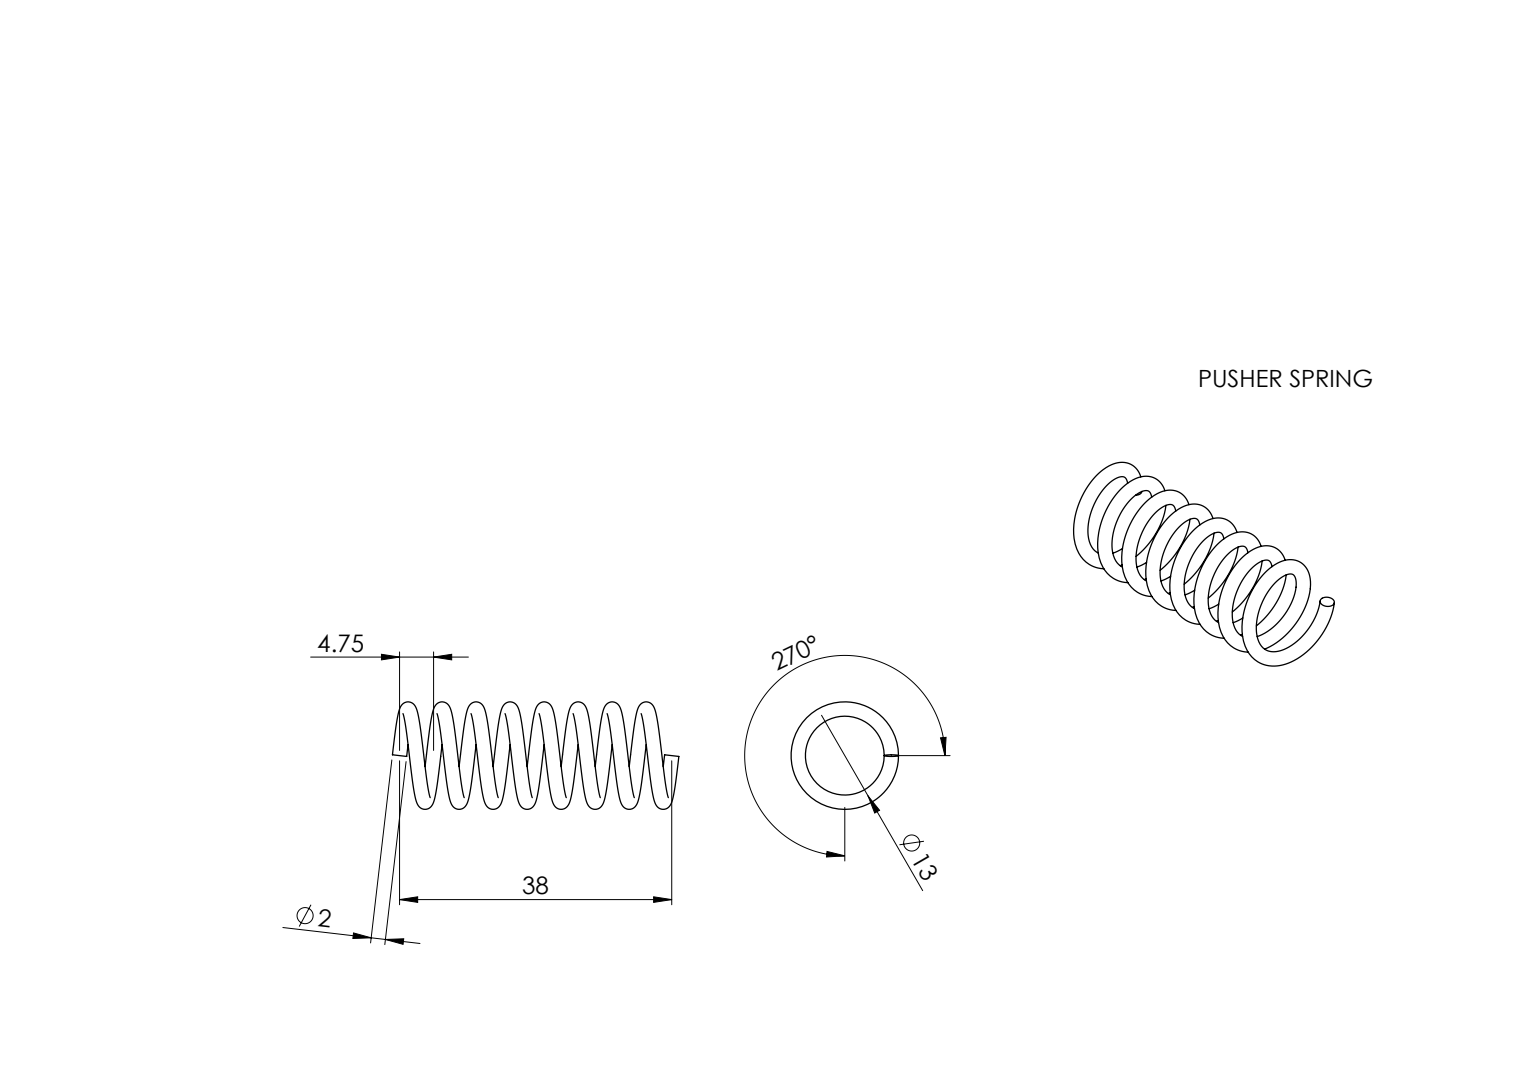
ISO-10303-21;
HEADER;
FILE_DESCRIPTION (('STEP AP214'),
    '1' );
FILE_NAME ('pusher spring.step',
    '2026-10-31T03:36:27',
    ( '' ),
    ( '' ),
    'SwSTEP 2.0',
    'SolidWorks 2026',
    '' );
FILE_SCHEMA (( 'AUTOMOTIVE_DESIGN' ));
ENDSEC;

DATA;
#2=CIRCLE ( 'NONE', #23019, 1.000000000000002220 ) ;
#26=CARTESIAN_POINT ( 'NONE',  ( -33.37127896937850124, 216.5309553116391612, 1.626142955000506873 ) ) ;
#28=( LENGTH_UNIT ( ) NAMED_UNIT ( * ) SI_UNIT ( .MILLI., .METRE. ) );
#30=CARTESIAN_POINT ( 'NONE',  ( -63.25669563604515844, 209.8844732041982297, -4.499999999999996447 ) ) ;
#31=CARTESIAN_POINT ( 'NONE',  ( -50.99330436395489841, 210.1155267958017134, -6.500000000000000888 ) ) ;
#37=CARTESIAN_POINT ( 'NONE',  ( -60.49330436395489130, 210.1155267958016850, -8.500000000000003553 ) ) ;
#42=CARTESIAN_POINT ( 'NONE',  ( -39.90997103062156270, 215.5714017266979852, 3.350049139982118618 ) ) ;
#53=CARTESIAN_POINT ( 'NONE',  ( -55.74330436395489841, 210.1155267958017134, -6.500000000000000888 ) ) ;
#71=( BOUNDED_CURVE ( )  B_SPLINE_CURVE ( 2, ( #25117, #31002, #36483, #31184, #33841, #22103, #11088, #7506, #25303, #25677, #37040, #22287, #37228, #16414, #5388, #22845, #19080, #4648, #7879, #11276, #5022, #24930, #13939, #16602, #28145, #33652, #16967, #25488, #30632, #10526, #31363, #36855, #10899, #7691, #16229, #4836, #13565, #22472, #28510, #14121, #27961, #34021, #8065, #19272, #19642, #36675, #30813, #10713, #22664, #5207, #2366, #16783, #28328, #1992, #34208, #8252, #19826, #3481, #14864, #31546, #34574, #20184, #28698, #32288, #14673, #14488, #2918, #17156, #23026, #25859, #2734, #8803, #31734, #28883, #12011, #11824, #37407, #31918, #8433, #630, #20376, #11637, #14307, #26045, #5947, #34761, #259, #29446, #34943, #8614, #26223, #17711, #6330, #5761, #23395, #72, #23211, #17527, #29061, #17341, #11458, #3105, #8987, #5571, #20744, #20558, #32102, #6133, #29251, #3292, #26411, #445, #23583, #35126, #9176, #17901, #15050, #26599, #12197, #34392, #20002, #7093, #10110, #21503, #12580, #29821, #21681, #33046, #32473, #15615, #24517, #12767, #24336, #33233, #18662, #30202, #27169, #26790, #4043, #21125, #18472, #15240, #20939, #21313, #35877, #26980, #35310, #4415, #12391, #4228, #1192, #9919, #1386, #15997, #12957, #1007, #27545, #6897, #30013, #18847, #24147, #35689, #36067, #15805, #32850, #27355, #9742, #7272, #30392, #1571, #23771, #9365, #6518, #18093, #29634, #3670, #821, #23961, #35504, #9551, #32664, #6705, #18277, #3855, #15431, #16364, #22423, #24885, #34157, #21865, #2129, #13326, #5344 ),
 .UNSPECIFIED., .F., .F. ) 
 B_SPLINE_CURVE_WITH_KNOTS ( ( 3, 2, 2, 2, 2, 2, 2, 2, 2, 2, 2, 2, 2, 2, 2, 2, 2, 2, 2, 2, 2, 2, 2, 2, 2, 2, 2, 2, 2, 2, 2, 2, 2, 2, 2, 2, 2, 2, 2, 2, 2, 2, 2, 2, 2, 2, 2, 2, 2, 2, 2, 2, 2, 2, 2, 2, 2, 2, 2, 2, 2, 2, 2, 2, 2, 2, 2, 2, 2, 2, 2, 2, 2, 2, 2, 2, 2, 2, 2, 2, 2, 2, 2, 2, 2, 2, 2, 2, 2, 2, 2, 2, 2, 2, 2, 2, 3 ),
 ( 0.000000000000000000, 0.01041666666666666609, 0.02083333333333333218, 0.03125000000000000000, 0.04166666666666666435, 0.05208333333333333565, 0.06250000000000000000, 0.07291666666666667129, 0.08333333333333332871, 0.09375000000000000000, 0.1041666666666666713, 0.1145833333333333287, 0.1250000000000000000, 0.1354166666666666574, 0.1458333333333333426, 0.1562500000000000000, 0.1666666666666666574, 0.1770833333333333426, 0.1875000000000000000, 0.1979166666666666574, 0.2083333333333333426, 0.2187500000000000000, 0.2291666666666666574, 0.2395833333333333426, 0.2500000000000000000, 0.2604166666666666852, 0.2708333333333333148, 0.2812500000000000000, 0.2916666666666666852, 0.3020833333333333148, 0.3125000000000000000, 0.3229166666666666852, 0.3333333333333333148, 0.3437500000000000000, 0.3541666666666666852, 0.3645833333333333148, 0.3750000000000000000, 0.3854166666666666852, 0.3958333333333333148, 0.4062500000000000000, 0.4166666666666666852, 0.4270833333333333148, 0.4375000000000000000, 0.4479166666666666852, 0.4583333333333333148, 0.4687500000000000000, 0.4791666666666666852, 0.4895833333333333148, 0.5000000000000000000, 0.5104166666666666297, 0.5208333333333333703, 0.5312500000000000000, 0.5416666666666666297, 0.5520833333333333703, 0.5625000000000000000, 0.5729166666666666297, 0.5833333333333333703, 0.5937500000000000000, 0.6041666666666666297, 0.6145833333333333703, 0.6250000000000000000, 0.6354166666666666297, 0.6458333333333333703, 0.6562500000000000000, 0.6666666666666666297, 0.6770833333333333703, 0.6875000000000000000, 0.6979166666666666297, 0.7083333333333333703, 0.7187500000000000000, 0.7291666666666666297, 0.7395833333333333703, 0.7500000000000000000, 0.7604166666666666297, 0.7708333333333333703, 0.7812500000000000000, 0.7916666666666666297, 0.8020833333333333703, 0.8125000000000000000, 0.8229166666666666297, 0.8333333333333333703, 0.8437500000000000000, 0.8541666666666666297, 0.8645833333333333703, 0.8750000000000000000, 0.8854166666666666297, 0.8958333333333333703, 0.9062500000000000000, 0.9166666666666666297, 0.9270833333333333703, 0.9375000000000000000, 0.9479166666666666297, 0.9583333333333333703, 0.9687500000000000000, 0.9791666666666666297, 0.9895833333333333703, 1.000000000000000000 ),
 .UNSPECIFIED. ) 
 CURVE ( )  GEOMETRIC_REPRESENTATION_ITEM ( )  RATIONAL_B_SPLINE_CURVE ( ( 1.000000000000000000, 0.9659258262890683122, 1.000000000000000000, 0.9659258262890683122, 1.000000000000000000, 0.9659258262890683122, 1.000000000000000000, 0.9659258262890683122, 1.000000000000000000, 0.9659258262890683122, 1.000000000000000000, 0.9659258262890683122, 1.000000000000000000, 0.9659258262890683122, 1.000000000000000000, 0.9659258262890683122, 1.000000000000000000, 0.9659258262890683122, 1.000000000000000000, 0.9659258262890683122, 1.000000000000000000, 0.9659258262890683122, 1.000000000000000000, 0.9659258262890683122, 1.000000000000000000, 0.9659258262890683122, 1.000000000000000000, 0.9659258262890683122, 1.000000000000000000, 0.9659258262890683122, 1.000000000000000000, 0.9659258262890683122, 1.000000000000000000, 0.9659258262890683122, 1.000000000000000000, 0.9659258262890683122, 1.000000000000000000, 0.9659258262890683122, 1.000000000000000000, 0.9659258262890683122, 1.000000000000000000, 0.9659258262890683122, 1.000000000000000000, 0.9659258262890683122, 1.000000000000000000, 0.9659258262890683122, 1.000000000000000000, 0.9659258262890683122, 1.000000000000000000, 0.9659258262890683122, 1.000000000000000000, 0.9659258262890683122, 1.000000000000000000, 0.9659258262890683122, 1.000000000000000000, 0.9659258262890683122, 1.000000000000000000, 0.9659258262890683122, 1.000000000000000000, 0.9659258262890683122, 1.000000000000000000, 0.9659258262890683122, 1.000000000000000000, 0.9659258262890683122, 1.000000000000000000, 0.9659258262890683122, 1.000000000000000000, 0.9659258262890683122, 1.000000000000000000, 0.9659258262890683122, 1.000000000000000000, 0.9659258262890683122, 1.000000000000000000, 0.9659258262890683122, 1.000000000000000000, 0.9659258262890683122, 1.000000000000000000, 0.9659258262890683122, 1.000000000000000000, 0.9659258262890683122, 1.000000000000000000, 0.9659258262890683122, 1.000000000000000000, 0.9659258262890683122, 1.000000000000000000, 0.9659258262890683122, 1.000000000000000000, 0.9659258262890683122, 1.000000000000000000, 0.9659258262890683122, 1.000000000000000000, 0.9659258262890683122, 1.000000000000000000, 0.9659258262890683122, 1.000000000000000000, 0.9659258262890683122, 1.000000000000000000, 0.9659258262890683122, 1.000000000000000000, 0.9659258262890683122, 1.000000000000000000, 0.9659258262890683122, 1.000000000000000000, 0.9659258262890683122, 1.000000000000000000, 0.9659258262890683122, 1.000000000000000000, 0.9659258262890683122, 1.000000000000000000, 0.9659258262890683122, 1.000000000000000000, 0.9659258262890683122, 1.000000000000000000, 0.9659258262890683122, 1.000000000000000000, 0.9659258262890683122, 1.000000000000000000, 0.9659258262890683122, 1.000000000000000000, 0.9659258262890683122, 1.000000000000000000, 0.9659258262890683122, 1.000000000000000000, 0.9659258262890683122, 1.000000000000000000, 0.9659258262890683122, 1.000000000000000000, 0.9659258262890683122, 1.000000000000000000, 0.9659258262890683122, 1.000000000000000000, 0.9659258262890683122, 1.000000000000000000, 0.9659258262890683122, 1.000000000000000000, 0.9659258262890683122, 1.000000000000000000, 0.9659258262890683122, 1.000000000000000000, 0.9659258262890683122, 1.000000000000000000, 0.9659258262890683122, 1.000000000000000000, 0.9659258262890683122, 1.000000000000000000, 0.9659258262890683122, 1.000000000000000000, 0.9659258262890683122, 1.000000000000000000, 0.9659258262890683122, 1.000000000000000000, 0.9659258262890683122, 1.000000000000000000, 0.9659258262890683122, 1.000000000000000000, 0.9659258262890683122, 1.000000000000000000, 0.9659258262890683122, 1.000000000000000000, 0.9659258262890683122, 1.000000000000000000, 0.9659258262890683122, 1.000000000000000000, 0.9659258262890683122, 1.000000000000000000, 0.9659258262890683122, 1.000000000000000000, 0.9659258262890683122, 1.000000000000000000, 0.9659258262890683122, 1.000000000000000000, 0.9659258262890683122, 1.000000000000000000, 0.9659258262890683122, 1.000000000000000000, 0.9659258262890683122, 1.000000000000000000, 0.9659258262890683122, 1.000000000000000000, 0.9659258262890683122, 1.000000000000000000, 0.9659258262890683122, 1.000000000000000000, 0.9659258262890683122, 1.000000000000000000, 0.9659258262890683122, 1.000000000000000000, 0.9659258262890683122, 1.000000000000000000, 0.9659258262890683122, 1.000000000000000000, 0.9659258262890683122, 1.000000000000000000 ) ) 
 REPRESENTATION_ITEM ( '' )  );
#72=CARTESIAN_POINT ( 'NONE',  ( -49.20461230271183695, 208.1428034533958851, -6.469044688360754414 ) ) ;
#74=CARTESIAN_POINT ( 'NONE',  ( -39.30877896937850124, 211.0902445701383101, -4.530955311639234040 ) ) ;
#77=CARTESIAN_POINT ( 'NONE',  ( -61.28497103062156981, 206.1606490808709111, -2.350049139982163027 ) ) ;
#78=CARTESIAN_POINT ( 'NONE',  ( -39.90997103062156270, 217.3034525342668815, 4.350049139982096413 ) ) ;
#83=CARTESIAN_POINT ( 'NONE',  ( -60.88169563604516554, 210.1155267958018271, 8.500000000000003553 ) ) ;
#96=CARTESIAN_POINT ( 'NONE',  ( -46.63913769728824121, 206.8500491399821044, -5.686928522499717253 ) ) ;
#124=CARTESIAN_POINT ( 'NONE',  ( -40.10788769728823411, 214.4690446883608104, 1.321298161741840893 ) ) ;
#129=CARTESIAN_POINT ( 'NONE',  ( -55.74330436395489841, 210.1155267958017134, -6.500000000000000888 ) ) ;
#180=CARTESIAN_POINT ( 'NONE',  ( -31.99330436395490196, 210.1155267958017134, -6.500000000000000888 ) ) ;
#216=CARTESIAN_POINT ( 'NONE',  ( -66.02752896937849414, 214.3500491399821897, 7.303452534266821949 ) ) ;
#218=FILL_AREA_STYLE ('',( #11593 ) ) ;
#220=CARTESIAN_POINT ( 'NONE',  ( -53.55877896937850124, 211.0902445701383101, -4.530955311639234040 ) ) ;
#221=CARTESIAN_POINT ( 'NONE',  ( -38.52455436395488420, 205.1570982666397356, 4.673758765035198159 ) ) ;
#227=CARTESIAN_POINT ( 'NONE',  ( -57.72247103062156270, 205.6499508600178956, 7.303452534266880569 ) ) ;
#233=CARTESIAN_POINT ( 'NONE',  ( -36.74330436395489841, 210.1155267958017134, -6.500000000000000888 ) ) ;
#244=CARTESIAN_POINT ( 'NONE',  ( -53.56622103062157692, 211.6261429550005744, 6.530955311639227823 ) ) ;
#259=CARTESIAN_POINT ( 'NONE',  ( -50.98586230271183695, 206.8500491399821328, 5.686928522499748340 ) ) ;
#262=CARTESIAN_POINT ( 'NONE',  ( -31.39211230271183339, 205.5309553116392465, 1.321298161741817356 ) ) ;
#266=CARTESIAN_POINT ( 'NONE',  ( -65.44122103062156270, 208.9097554298617752, -4.530955311639240257 ) ) ;
#267=CARTESIAN_POINT ( 'NONE',  ( -66.03497103062157692, 204.4285982733020148, -3.350049139982115509 ) ) ;
#271=CARTESIAN_POINT ( 'NONE',  ( -52.96502896937850124, 217.3034525342667962, -4.350049139982195001 ) ) ;
#281=CARTESIAN_POINT ( 'NONE',  ( -50.59747103062156270, 213.3500491399821328, -5.571401726697985168 ) ) ;
#307=CARTESIAN_POINT ( 'NONE',  ( -65.43377896937850835, 208.9097554298617183, 4.530955311639234040 ) ) ;
#311=CARTESIAN_POINT ( 'NONE',  ( -65.83705436395487709, 205.3262412349647263, -4.842901733360204020 ) ) ;
#312=CARTESIAN_POINT ( 'NONE',  ( -48.61086230271182984, 214.1499508600178387, -7.418979330068641964 ) ) ;
#327=CARTESIAN_POINT ( 'NONE',  ( -69.79538769728823411, 211.8571965466040012, -6.469044688360769513 ) ) ;
#365=CARTESIAN_POINT ( 'NONE',  ( -36.54538769728823411, 211.8571965466039444, -6.469044688360768625 ) ) ;
#400=CARTESIAN_POINT ( 'NONE',  ( -34.95461230271183695, 208.1428034533959135, -6.469044688360754414 ) ) ;
#403=CARTESIAN_POINT ( 'NONE',  ( -55.14211230271182984, 205.5309553116392465, 1.321298161741817356 ) ) ;
#404=CARTESIAN_POINT ( 'NONE',  ( -34.36830436395490551, 209.8844732041982581, 6.500000000000000888 ) ) ;
#410=CARTESIAN_POINT ( 'NONE',  ( -56.33705436395490551, 203.8621396198270475, -6.307003348497942419 ) ) ;
#417=CARTESIAN_POINT ( 'NONE',  ( -42.68080436395489841, 203.5000000000000000, -0.1155267958017335561 ) ) ;
#430=CARTESIAN_POINT ( 'NONE',  ( -58.51413769728823411, 213.1499508600178672, 5.686928522499718142 ) ) ;
#445=CARTESIAN_POINT ( 'NONE',  ( -46.03794563604517265, 205.3262412349648116, 4.842901733360249317 ) ) ;
#447=CARTESIAN_POINT ( 'NONE',  ( -64.64211230271182274, 203.5309553116391612, 1.857196546604092280 ) ) ;
#450=CARTESIAN_POINT ( 'NONE',  ( -63.26413769728823411, 212.1499508600178387, 3.954877714930865817 ) ) ;
#451=CARTESIAN_POINT ( 'NONE',  ( -32.38913769728823411, 205.8500491399820760, -7.418979330068584233 ) ) ;
#455=CARTESIAN_POINT ( 'NONE',  ( -56.72544563604517265, 216.3070033484980854, 6.137860380172893926 ) ) ;
#467=CARTESIAN_POINT ( 'NONE',  ( -46.83705436395489841, 205.3262412349647263, -4.842901733360204020 ) ) ;
#494=CARTESIAN_POINT ( 'NONE',  ( -33.18080436395489841, 205.4999999999999716, -0.1155267958017894420 ) ) ;
#498=CARTESIAN_POINT ( 'NONE',  ( -65.44122103062157692, 208.3738570449993404, -6.530955311639226935 ) ) ;
#499=CARTESIAN_POINT ( 'NONE',  ( -35.35044563604517265, 203.6929966515019430, -6.137860380172892150 ) ) ;
#504=CARTESIAN_POINT ( 'NONE',  ( -52.37127896937850124, 216.5309553116391612, 1.626142955000506873 ) ) ;
#548=CARTESIAN_POINT ( 'NONE',  ( -33.57663769728823411, 204.3130714775002730, 3.149950860017883603 ) ) ;
#566=FACE_OUTER_BOUND ( 'NONE', #21711, .T. ) ;
#583=CARTESIAN_POINT ( 'NONE',  ( -65.82961230271185116, 212.3930949314663792, 8.469044688360751749 ) ) ;
#587=CARTESIAN_POINT ( 'NONE',  ( -59.69419563604517265, 205.4999999999999716, 0.1155267958017633378 ) ) ;
#593=CARTESIAN_POINT ( 'NONE',  ( -61.68080436395489841, 201.5000000000000000, -0.1155267958017054536 ) ) ;
#600=CARTESIAN_POINT ( 'NONE',  ( -35.75372103062156981, 216.5309553116392181, -1.626142955000564383 ) ) ;
#613=CARTESIAN_POINT ( 'NONE',  ( -50.59747103062156270, 213.3500491399821328, -5.571401726697985168 ) ) ;
#630=CARTESIAN_POINT ( 'NONE',  ( -52.37127896937850124, 216.5309553116392181, 1.626142955000506429 ) ) ;
#632=CARTESIAN_POINT ( 'NONE',  ( -65.03794563604516554, 205.3262412349647832, 4.842901733360250205 ) ) ;
#635=CARTESIAN_POINT ( 'NONE',  ( -66.03497103062157692, 206.1606490808709111, -2.350049139982163027 ) ) ;
#636=CARTESIAN_POINT ( 'NONE',  ( -32.98288769728823411, 201.5309553116392181, -2.393094931466246855 ) ) ;
#641=CARTESIAN_POINT ( 'NONE',  ( -53.75669563604516554, 209.8844732041981729, -8.500000000000003553 ) ) ;
#652=CARTESIAN_POINT ( 'NONE',  ( -55.74330436395489841, 210.1155267958017134, -6.500000000000000888 ) ) ;
#680=CARTESIAN_POINT ( 'NONE',  ( -66.02752896937849414, 212.3500491399821613, 3.839350919129088435 ) ) ;
#684=CARTESIAN_POINT ( 'NONE',  ( -58.11830436395490551, 209.8844732041982581, 6.500000000000000888 ) ) ;
#685=CARTESIAN_POINT ( 'NONE',  ( -66.82663769728823411, 202.5810206699313767, 4.149950860017909804 ) ) ;
#690=CARTESIAN_POINT ( 'NONE',  ( -63.05877896937850835, 211.6261429550004607, -6.530955311639245586 ) ) ;
#697=CARTESIAN_POINT ( 'NONE',  ( -64.45163769728823411, 215.6869285224996986, -3.149950860017881382 ) ) ;
#736=CARTESIAN_POINT ( 'NONE',  ( -68.21205436395490551, 213.2096571498974242, 3.378800118222489601 ) ) ;
#777=CARTESIAN_POINT ( 'NONE',  ( -63.05877896937850835, 212.1620413398627534, -8.530955311639255356 ) ) ;
#780=CARTESIAN_POINT ( 'NONE',  ( -48.61086230271182984, 212.1499508600178387, -3.954877714930852495 ) ) ;
#781=CARTESIAN_POINT ( 'NONE',  ( -36.74330436395489841, 210.1155267958017134, -6.500000000000000888 ) ) ;
#786=CARTESIAN_POINT ( 'NONE',  ( -66.62872103062156270, 201.4690446883607819, 2.162041339862843525 ) ) ;
#793=CARTESIAN_POINT ( 'NONE',  ( -32.58705436395489841, 205.3262412349647548, -4.842901733360204908 ) ) ;
#821=CARTESIAN_POINT ( 'NONE',  ( -33.17336230271182984, 215.6869285224997270, 3.149950860017831200 ) ) ;
#823=CARTESIAN_POINT ( 'NONE',  ( -66.22544563604516554, 214.8429017333602360, 4.673758765035156415 ) ) ;
#828=CARTESIAN_POINT ( 'NONE',  ( -48.42038769728824832, 208.6787018382581778, 4.469044688360752637 ) ) ;
#829=CARTESIAN_POINT ( 'NONE',  ( -37.13913769728823411, 205.8500491399820760, -7.418979330068584233 ) ) ;
#833=CARTESIAN_POINT ( 'NONE',  ( -58.11086230271183695, 214.1499508600178387, -7.418979330068641964 ) ) ;
#842=CARTESIAN_POINT ( 'NONE',  ( -37.73288769728821279, 203.5309553116391612, -1.857196546604028775 ) ) ;
#871=CARTESIAN_POINT ( 'NONE',  ( -65.03794563604515133, 206.7903428501025758, 3.378800118222471838 ) ) ;
#875=CARTESIAN_POINT ( 'NONE',  ( -54.15997103062156981, 215.5714017266979852, 3.350049139982118618 ) ) ;
#876=CARTESIAN_POINT ( 'NONE',  ( -69.59747103062156270, 214.3500491399821044, -7.303452534266878793 ) ) ;
#881=CARTESIAN_POINT ( 'NONE',  ( -64.04836230271183695, 204.3130714775002446, -3.149950860017828091 ) ) ;
#888=CARTESIAN_POINT ( 'NONE',  ( -62.67038769728823411, 208.1428034533959703, 6.469044688360771289 ) ) ;
#893=CARTESIAN_POINT ( 'NONE',  ( -69.39955436395486288, 214.8429017333601792, -4.673758765035196383 ) ) ;
#965=CARTESIAN_POINT ( 'NONE',  ( -60.68377896937850835, 207.8379586601372750, 8.530955311639258909 ) ) ;
#969=CARTESIAN_POINT ( 'NONE',  ( -46.23586230271182984, 207.8500491399821613, 3.954877714930852495 ) ) ;
#974=CARTESIAN_POINT ( 'NONE',  ( -51.38913769728824121, 205.8500491399820760, -7.418979330068584233 ) ) ;
#1007=CARTESIAN_POINT ( 'NONE',  ( -37.32961230271182274, 211.8571965466040581, 6.469044688360755302 ) ) ;
#1008=CARTESIAN_POINT ( 'NONE',  ( -63.25669563604516554, 209.8844732041982013, -6.500000000000000888 ) ) ;
#1011=CARTESIAN_POINT ( 'NONE',  ( -44.85788769728823411, 214.4690446883608104, 1.321298161741840893 ) ) ;
#1012=CARTESIAN_POINT ( 'NONE',  ( -34.56622103062156981, 212.1620413398628671, 8.530955311639223382 ) ) ;
#1017=CARTESIAN_POINT ( 'NONE',  ( -50.78794563604517975, 203.8621396198271043, 6.307003348498029460 ) ) ;
#1031=CARTESIAN_POINT ( 'NONE',  ( -32.98288769728824121, 203.5309553116391612, -1.857196546604028775 ) ) ;
#1056=CARTESIAN_POINT ( 'NONE',  ( -34.17038769728823411, 208.6787018382581778, 4.469044688360752637 ) ) ;
#1061=CARTESIAN_POINT ( 'NONE',  ( -52.77455436395490551, 205.1570982666397356, 4.673758765035198159 ) ) ;
#1062=CARTESIAN_POINT ( 'NONE',  ( -67.61830436395490551, 209.8844732041983150, 8.500000000000003553 ) ) ;
#1069=CARTESIAN_POINT ( 'NONE',  ( -55.34002896937850124, 204.4285982733020433, 3.350049139982171020 ) ) ;
#1078=CARTESIAN_POINT ( 'NONE',  ( -69.39955436395487709, 214.8429017333601792, -4.673758765035197271 ) ) ;
#1082=CARTESIAN_POINT ( 'NONE',  ( -39.90997103062156270, 217.3034525342668815, 4.350049139982096413 ) ) ;
#1096=( BOUNDED_SURFACE ( )  B_SPLINE_SURFACE ( 3, 2, ( 
 ( #17208, #19878, #22527, #2787, #34446, #8486, #20056, #31601, #31421, #7933, #5265, #5624, #19508, #23080, #16843, #31054, #16469, #5076, #14361, #28202, #8124, #311, #26279, #498, #17583, #11877, #23446, #29308, #34999, #21179, #14915, #17398, #12254, #12064, #32344, #23638, #9227, #2973, #24016, #32154, #23824, #35366, #26464, #35561, #31973, #9418, #3160, #3347, #9042, #9605, #3538, #23266, #29499, #20993, #20801, #5816, #15293, #28938, #6003, #32528, #684, #35181, #14543, #6381, #26098, #17956, #11693, #20614, #34810, #26845, #15103, #26653, #129, #18145, #6571, #29687, #3721, #6194, #17766, #8855, #875, #12447, #20429, #29116, #14731, #13200, #6758, #1061, #29877, #18528, #30258, #30453, #27597, #13014, #12634, #9974, #15482, #33101, #21554, #24387, #16236, #1248, #24752, #18332, #24199, #3910, #30066, #4284, #4471, #1628, #24568, #35744, #36301, #27037, #9790, #27787, #30637, #16050, #36490, #10162, #1814, #7144, #10533, #7512, #15673, #13382, #32718, #24935, #21367, #12818, #32906, #10348, #21921, #33470, #35932, #6960, #18901, #4101, #18718, #19086, #27223, #15861, #27406, #1438, #36122, #4654, #21737, #33288, #7327, #2558, #14127, #25683, #8258, #19648, #16421, #10906, #37233, #25124, #31553, #22480, #13572, #17163, #28703, #28335, #13946, #31370, #16608, #5028, #16790, #33846, #28151, #2181, #8072, #13763, #37414, #31190, #33658, #28515, #2372, #11095, #25495, #37047, #19278, #2740, #34027, #11281, #22851, #5213, #14312, #10719, #34400, #19459, #22669 ),
 ( #34213, #25865, #5577, #22109, #22293, #8438, #16973, #19831, #7698, #5393, #30818, #20007, #27968, #25309, #36681, #4842, #1998, #7885, #31008, #36861, #635, #26606, #3297, #266, #23218, #31923, #29067, #34948, #3112, #26796, #20564, #23033, #17907, #17717, #450, #29256, #14869, #8621, #29639, #11829, #29451, #3486, #32106, #3676, #77, #15056, #8809, #8994, #14678, #15245, #9181, #28890, #35130, #12205, #26415, #11464, #20945, #34580, #11642, #23777, #6335, #6140, #20190, #12018, #31739, #23588, #17347, #5954, #2924, #32478, #20750, #32295, #5767, #35315, #9370, #6525, #18099, #23400, #26228, #14493, #26050, #34767, #20381, #17533, #6905, #18851, #12395, #6711, #35510, #24151, #35881, #36071, #33238, #18666, #18283, #7277, #9556, #3862, #33422, #36254, #10115, #4606, #15810, #7460, #27174, #16186, #13148, #21318, #19039, #828, #30591, #21131, #18477, #23967, #30398, #21686, #27549, #30018, #32669, #24522, #26985, #15620, #1577, #12585, #29826, #21869, #15436, #1011, #24702, #33051, #35694, #10297, #4421, #16002, #9746, #32856, #9924, #4048, #1198, #12771, #24341, #21507, #7098, #30207, #4234, #27360, #1390, #12963, #36998, #22247, #10668, #22430, #31142, #24890, #8392, #16557, #8208, #19784, #36814, #19961, #16371, #31321, #25074, #25263, #7835, #31504, #25445, #7650, #13897, #5349, #5161, #5526, #37184, #27735, #27916, #16926, #22617, #10857, #1766, #16740, #13332, #2325, #33611, #33798, #19227, #11227, #28287, #11041, #36440, #2505, #28468, #14078, #19594 ),
 ( #22798, #19408, #25628, #10479, #30771, #22058, #13517, #33978, #34164, #34349, #8019, #4793, #1946, #36628, #30958, #4976, #28103, #2135, #13714, #32060, #12156, #5905, #20893, #29406, #30, #23731, #32436, #35268, #25816, #34713, #9324, #23542, #26370, #6286, #23170, #17112, #3251, #5716, #31875, #17862, #28838, #28652, #587, #37361, #2689, #3438, #11784, #2872, #15007, #35087, #9137, #20702, #14825, #14632, #11415, #17485, #32246, #20140, #26559, #29017, #8572, #14265, #22983, #23352, #8948, #403, #11595, #8759, #34904, #14445, #20333, #3063, #26182, #220, #34533, #20521, #31687, #17297, #6089, #17673, #29210, #26001, #11970, #33197, #18239, #6480, #27511, #26748, #18052, #7238, #1159, #29783, #18812, #24483, #36029, #10073, #30166, #4003, #780, #32813, #21644, #9514, #15957, #6856, #35463, #1534, #13106, #12731, #35841, #15770, #969, #26938, #24298, #3814, #12545, #24110, #29973, #35654, #21831, #15578, #29594, #12920, #9883, #33005, #21464, #7055, #3631, #24661, #18432, #30356, #4380, #27132, #36213, #32627, #10255, #15391, #18625, #9700, #15200, #4193, #23922, #27320, #12348, #1348, #21087, #6664, #21277, #33572, #22574, #28251, #4933, #7425, #22388, #11185, #7980, #1723, #16328, #24848, #5310, #33938, #19553, #37143, #8170, #34120, #11002, #25223, #22206, #10627, #16144, #33755, #7795, #25029, #16888, #1907, #13857, #18994, #13292, #30551, #19184, #30914, #31102, #2280, #13675, #36398, #25405, #4568, #10444, #28424, #31282, #5123, #33385, #10817, #2465 ),
 ( #19745, #27876, #19372, #14039, #25588, #36956, #16703, #27695, #28062, #16515, #7608, #36772, #22019, #30733, #13477, #4756, #36588, #2097, #18152, #14922, #881, #35566, #29885, #35005, #12452, #690, #32726, #22759, #6576, #15109, #35188, #20999, #9233, #3916, #29693, #6763, #17963, #20808, #18337, #24021, #32350, #32536, #9612, #3546, #19925, #15489, #35372, #5485, #3726, #23831, #9048, #26471, #6388, #29505, #26660, #15299, #20620, #12261, #9424, #26852, #27043, #17068, #32160, #3354, #1069, #31463, #21186, #34308, #8352, #28608, #2645, #14221, #25771, #37323, #17772, #23452, #11884, #6199, #29314, #504, #12070, #23645, #4291, #9980, #1635, #16056, #13020, #24576, #36307, #1819, #33106, #1444, #33663, #27792, #4659, #27604, #10538, #7334, #36127, #24392, #24757, #33293, #7151, #12640, #7703, #27230, #1255, #30825, #10169, #18724, #24940, #12824, #21373, #4477, #27412, #32912, #18907, #13207, #21744, #4107, #6966, #30460, #10355, #30265, #4848, #13388, #22115, #16243, #36495, #35939, #21928, #15679, #33475, #7519, #27973, #16427, #19091, #30643, #35750, #21561, #19286, #24205, #15869, #9795, #18534, #30072, #13768, #17168, #16978, #11469, #2004, #22856, #31378, #13952, #37238, #25501, #20195, #34406, #23039, #34219, #37053, #34585, #28709, #11101, #11288, #2744, #19837, #36686, #31745, #14133, #22299, #8444, #2563, #25315, #5220, #22674, #8264, #5398, #20012, #36866, #28521, #25689, #31558, #5773, #33851, #10911, #19653, #8627, #10724, #5582, #17353, #14318, #37419 ),
 ( #25871, #13577, #25130, #7892, #2187, #19466, #31195, #22488, #31013, #5034, #2377, #16614, #28156, #34034, #8078, #28342, #16796, #6530, #20950, #6341, #26801, #23593, #29263, #3117, #3491, #12024, #11834, #28895, #12400, #5960, #17539, #9561, #26421, #23405, #3682, #29073, #83, #20755, #6145, #11647, #35135, #32301, #17722, #20387, #23223, #9187, #17911, #34954, #21137, #18104, #833, #32483, #15250, #14684, #29456, #31928, #12210, #455, #6717, #32674, #3303, #14873, #14498, #15062, #23973, #34772, #8999, #2930, #29644, #26612, #26055, #8813, #641, #26233, #23783, #35321, #271, #32111, #9376, #35516, #20569, #1583, #4053, #4239, #7282, #24708, #36445, #1017, #27179, #35887, #13337, #15441, #15815, #1771, #4426, #16192, #19045, #1395, #27742, #12590, #12776, #18483, #36260, #27365, #10303, #21874, #30023, #36076, #9931, #15626, #18856, #21692, #18672, #30214, #16008, #7466, #1203, #7103, #24896, #33426, #30596, #33242, #10485, #12970, #24527, #24346, #30404, #10120, #21512, #18289, #22065, #32864, #6912, #33616, #27556, #33056, #4611, #13153, #26989, #29832, #3868, #24156, #35699, #9751, #21324, #36634, #1952, #13903, #25451, #2140, #25823, #34355, #17120, #11234, #31510, #7841, #8215, #10673, #28475, #5168, #22990, #37370, #19599, #31149, #30775, #37004, #5533, #13522, #13720, #7655, #22252, #2696, #2514, #36820, #22806, #19968, #14272, #19413, #8400, #22623, #28658, #19232, #14085, #11047, #16746, #5355, #28293, #11423, #25635, #4798, #2332, #34170, #16376 ),
 ( #37191, #19790, #25079, #27921, #33804, #30963, #4981, #16563, #16933, #28109, #31327, #25268, #33982, #10862, #22435, #8025, #3637, #786, #15206, #5723, #14638, #26755, #3444, #6293, #23736, #3070, #12356, #20709, #23176, #11790, #35275, #8766, #34540, #18057, #17304, #8579, #9330, #29216, #20340, #20901, #15013, #26565, #593, #32252, #32068, #28845, #23358, #12163, #37, #6486, #34910, #26008, #29600, #20148, #3258, #26376, #17868, #29026, #17491, #14832, #31882, #26189, #227, #20526, #8954, #31694, #6096, #2879, #32442, #410, #23548, #11975, #35094, #14452, #11602, #17679, #34721, #5912, #9143, #29413, #26945, #10080, #35660, #1165, #6863, #1542, #27326, #29789, #4200, #24490, #7061, #13112, #4386, #24668, #974, #33204, #12926, #12737, #35469, #18632, #36219, #30172, #18245, #9707, #3820, #15964, #15777, #1354, #23928, #27517, #18818, #7244, #36036, #27138, #15584, #15398, #24304, #35847, #4010, #9521, #29980, #30362, #32633, #12551, #6671, #21093, #24117, #21283, #32819, #21650, #18439, #9889, #21472, #33012, #18920, #32738, #6774, #24033, #12837, #10368, #13031, #24771, #27617, #9991, #36321, #21199, #21385, #27056, #33307, #35952, #7347, #30471, #1082, #7162, #18547, #24217, #15881, #30276, #27243, #1266, #24587, #16069, #9807, #15692, #21943, #4492, #1648, #4302, #33488, #21572, #24404, #12652, #1458, #33118, #32925, #26864, #7533, #3928, #15501, #19106, #18735, #6977, #13220, #35762, #35578, #27425, #4119, #9622, #36139, #10180, #21756, #18349, #29897 ),
 ( #30657, #4672, #30086, #893, #12464, #27987, #36698, #33863, #2201, #7905, #31570, #25329, #27805, #22688, #22499, #5235, #34046, #19666, #13402, #34417, #5047, #34232, #8275, #36878, #8455, #4861, #19848, #13594, #13781, #19478, #20024, #13963, #33676, #2389, #31390, #31206, #16255, #25699, #1833, #16441, #5410, #11112, #10924, #24951, #16811, #36509, #28352, #22129, #10738, #7716, #37251, #25512, #37065, #10553, #16992, #19298, #30837, #2016, #25144, #8093, #28532, #2575, #14146, #22311, #11299, #31025, #16629, #22867, #28171, #14886, #9388, #20580, #652, #31939, #20962, #17923, #26068, #12222, #5592, #23793, #14329, #23234, #35332, #12035, #26433, #32312, #11658, #17179, #29275, #31755, #20398, #6354, #17365, #28720, #26622, #25883, #2757, #29468, #281, #28906, #3504, #23603, #35148, #9200, #3314, #3129, #37431, #5971, #20768, #8638, #15072, #17551, #34595, #11481, #23051, #11847, #34967, #467, #96, #34782, #23416, #2942, #8826, #29087, #14696, #26245, #20206, #9010, #5785, #14512, #32124, #6161, #17734, #35900, #29656, #13164, #21337, #12982, #24538, #4068, #24719, #21147, #36088, #29842, #30034, #12603, #36271, #30226, #12413, #18685, #10132, #9943, #10315, #4438, #32494, #32685, #21705, #27376, #15640, #6541, #21523, #18114, #7114, #842, #15452, #23985, #16019, #33070, #4252, #3692, #7294, #33255, #18868, #24358, #32876, #9761, #15260, #6923, #15826, #1406, #35529, #26813, #24167, #9573, #30416, #27567, #1596, #1031, #6729, #18302, #3878, #18494, #27004 ) ),
 .UNSPECIFIED., .T., .F., .F. ) 
 B_SPLINE_SURFACE_WITH_KNOTS ( ( 4, 3, 4 ),
 ( 3, 2, 2, 2, 2, 2, 2, 2, 2, 2, 2, 2, 2, 2, 2, 2, 2, 2, 2, 2, 2, 2, 2, 2, 2, 2, 2, 2, 2, 2, 2, 2, 2, 2, 2, 2, 2, 2, 2, 2, 2, 2, 2, 2, 2, 2, 2, 2, 2, 2, 2, 2, 2, 2, 2, 2, 2, 2, 2, 2, 2, 2, 2, 2, 2, 2, 2, 2, 2, 2, 2, 2, 2, 2, 2, 2, 2, 2, 2, 2, 2, 2, 2, 2, 2, 2, 2, 2, 2, 2, 2, 2, 2, 2, 2, 2, 3 ),
 ( 0.000000000000000000, 0.5000000000000000000, 1.000000000000000000 ),
 ( 0.000000000000000000, 0.01041666666666666609, 0.02083333333333333218, 0.03125000000000000000, 0.04166666666666666435, 0.05208333333333333565, 0.06250000000000000000, 0.07291666666666667129, 0.08333333333333332871, 0.09375000000000000000, 0.1041666666666666713, 0.1145833333333333287, 0.1250000000000000000, 0.1354166666666666574, 0.1458333333333333426, 0.1562500000000000000, 0.1666666666666666574, 0.1770833333333333426, 0.1875000000000000000, 0.1979166666666666574, 0.2083333333333333426, 0.2187500000000000000, 0.2291666666666666574, 0.2395833333333333426, 0.2500000000000000000, 0.2604166666666666852, 0.2708333333333333148, 0.2812500000000000000, 0.2916666666666666852, 0.3020833333333333148, 0.3125000000000000000, 0.3229166666666666852, 0.3333333333333333148, 0.3437500000000000000, 0.3541666666666666852, 0.3645833333333333148, 0.3750000000000000000, 0.3854166666666666852, 0.3958333333333333148, 0.4062500000000000000, 0.4166666666666666852, 0.4270833333333333148, 0.4375000000000000000, 0.4479166666666666852, 0.4583333333333333148, 0.4687500000000000000, 0.4791666666666666852, 0.4895833333333333148, 0.5000000000000000000, 0.5104166666666666297, 0.5208333333333333703, 0.5312500000000000000, 0.5416666666666666297, 0.5520833333333333703, 0.5625000000000000000, 0.5729166666666666297, 0.5833333333333333703, 0.5937500000000000000, 0.6041666666666666297, 0.6145833333333333703, 0.6250000000000000000, 0.6354166666666666297, 0.6458333333333333703, 0.6562500000000000000, 0.6666666666666666297, 0.6770833333333333703, 0.6875000000000000000, 0.6979166666666666297, 0.7083333333333333703, 0.7187500000000000000, 0.7291666666666666297, 0.7395833333333333703, 0.7500000000000000000, 0.7604166666666666297, 0.7708333333333333703, 0.7812500000000000000, 0.7916666666666666297, 0.8020833333333333703, 0.8125000000000000000, 0.8229166666666666297, 0.8333333333333333703, 0.8437500000000000000, 0.8541666666666666297, 0.8645833333333333703, 0.8750000000000000000, 0.8854166666666666297, 0.8958333333333333703, 0.9062500000000000000, 0.9166666666666666297, 0.9270833333333333703, 0.9375000000000000000, 0.9479166666666666297, 0.9583333333333333703, 0.9687500000000000000, 0.9791666666666666297, 0.9895833333333333703, 1.000000000000000000 ),
 .UNSPECIFIED. ) 
 GEOMETRIC_REPRESENTATION_ITEM ( )  RATIONAL_B_SPLINE_SURFACE ( (
 ( 1.000000000000000000, 0.9659258262890683122, 1.000000000000000000, 0.9659258262890683122, 1.000000000000000000, 0.9659258262890683122, 1.000000000000000000, 0.9659258262890683122, 1.000000000000000000, 0.9659258262890683122, 1.000000000000000000, 0.9659258262890683122, 1.000000000000000000, 0.9659258262890683122, 1.000000000000000000, 0.9659258262890683122, 1.000000000000000000, 0.9659258262890683122, 1.000000000000000000, 0.9659258262890683122, 1.000000000000000000, 0.9659258262890683122, 1.000000000000000000, 0.9659258262890683122, 1.000000000000000000, 0.9659258262890683122, 1.000000000000000000, 0.9659258262890683122, 1.000000000000000000, 0.9659258262890683122, 1.000000000000000000, 0.9659258262890683122, 1.000000000000000000, 0.9659258262890683122, 1.000000000000000000, 0.9659258262890683122, 1.000000000000000000, 0.9659258262890683122, 1.000000000000000000, 0.9659258262890683122, 1.000000000000000000, 0.9659258262890683122, 1.000000000000000000, 0.9659258262890683122, 1.000000000000000000, 0.9659258262890683122, 1.000000000000000000, 0.9659258262890683122, 1.000000000000000000, 0.9659258262890683122, 1.000000000000000000, 0.9659258262890683122, 1.000000000000000000, 0.9659258262890683122, 1.000000000000000000, 0.9659258262890683122, 1.000000000000000000, 0.9659258262890683122, 1.000000000000000000, 0.9659258262890683122, 1.000000000000000000, 0.9659258262890683122, 1.000000000000000000, 0.9659258262890683122, 1.000000000000000000, 0.9659258262890683122, 1.000000000000000000, 0.9659258262890683122, 1.000000000000000000, 0.9659258262890683122, 1.000000000000000000, 0.9659258262890683122, 1.000000000000000000, 0.9659258262890683122, 1.000000000000000000, 0.9659258262890683122, 1.000000000000000000, 0.9659258262890683122, 1.000000000000000000, 0.9659258262890683122, 1.000000000000000000, 0.9659258262890683122, 1.000000000000000000, 0.9659258262890683122, 1.000000000000000000, 0.9659258262890683122, 1.000000000000000000, 0.9659258262890683122, 1.000000000000000000, 0.9659258262890683122, 1.000000000000000000, 0.9659258262890683122, 1.000000000000000000, 0.9659258262890683122, 1.000000000000000000, 0.9659258262890683122, 1.000000000000000000, 0.9659258262890683122, 1.000000000000000000, 0.9659258262890683122, 1.000000000000000000, 0.9659258262890683122, 1.000000000000000000, 0.9659258262890683122, 1.000000000000000000, 0.9659258262890683122, 1.000000000000000000, 0.9659258262890683122, 1.000000000000000000, 0.9659258262890683122, 1.000000000000000000, 0.9659258262890683122, 1.000000000000000000, 0.9659258262890683122, 1.000000000000000000, 0.9659258262890683122, 1.000000000000000000, 0.9659258262890683122, 1.000000000000000000, 0.9659258262890683122, 1.000000000000000000, 0.9659258262890683122, 1.000000000000000000, 0.9659258262890683122, 1.000000000000000000, 0.9659258262890683122, 1.000000000000000000, 0.9659258262890683122, 1.000000000000000000, 0.9659258262890683122, 1.000000000000000000, 0.9659258262890683122, 1.000000000000000000, 0.9659258262890683122, 1.000000000000000000, 0.9659258262890683122, 1.000000000000000000, 0.9659258262890683122, 1.000000000000000000, 0.9659258262890683122, 1.000000000000000000, 0.9659258262890683122, 1.000000000000000000, 0.9659258262890683122, 1.000000000000000000, 0.9659258262890683122, 1.000000000000000000, 0.9659258262890683122, 1.000000000000000000, 0.9659258262890683122, 1.000000000000000000, 0.9659258262890683122, 1.000000000000000000, 0.9659258262890683122, 1.000000000000000000, 0.9659258262890683122, 1.000000000000000000, 0.9659258262890683122, 1.000000000000000000, 0.9659258262890683122, 1.000000000000000000, 0.9659258262890683122, 1.000000000000000000, 0.9659258262890683122, 1.000000000000000000, 0.9659258262890683122, 1.000000000000000000, 0.9659258262890683122, 1.000000000000000000, 0.9659258262890683122, 1.000000000000000000, 0.9659258262890683122, 1.000000000000000000, 0.9659258262890683122, 1.000000000000000000, 0.9659258262890683122, 1.000000000000000000, 0.9659258262890683122, 1.000000000000000000, 0.9659258262890683122, 1.000000000000000000, 0.9659258262890683122, 1.000000000000000000, 0.9659258262890683122, 1.000000000000000000, 0.9659258262890683122, 1.000000000000000000, 0.9659258262890683122, 1.000000000000000000, 0.9659258262890683122, 1.000000000000000000, 0.9659258262890683122, 1.000000000000000000),
 ( 0.3333333333333333703, 0.3219752754296894559, 0.3333333333333333703, 0.3219752754296894559, 0.3333333333333333703, 0.3219752754296894559, 0.3333333333333333703, 0.3219752754296894559, 0.3333333333333333703, 0.3219752754296894559, 0.3333333333333333703, 0.3219752754296894559, 0.3333333333333333703, 0.3219752754296894559, 0.3333333333333333703, 0.3219752754296894559, 0.3333333333333333703, 0.3219752754296894559, 0.3333333333333333703, 0.3219752754296894559, 0.3333333333333333703, 0.3219752754296894559, 0.3333333333333333703, 0.3219752754296894559, 0.3333333333333333703, 0.3219752754296894559, 0.3333333333333333703, 0.3219752754296894559, 0.3333333333333333703, 0.3219752754296894559, 0.3333333333333333703, 0.3219752754296894559, 0.3333333333333333703, 0.3219752754296894559, 0.3333333333333333703, 0.3219752754296894559, 0.3333333333333333703, 0.3219752754296894559, 0.3333333333333333703, 0.3219752754296894559, 0.3333333333333333703, 0.3219752754296894559, 0.3333333333333333703, 0.3219752754296894559, 0.3333333333333333703, 0.3219752754296894559, 0.3333333333333333703, 0.3219752754296894559, 0.3333333333333333703, 0.3219752754296894559, 0.3333333333333333703, 0.3219752754296894559, 0.3333333333333333703, 0.3219752754296894559, 0.3333333333333333703, 0.3219752754296894559, 0.3333333333333333703, 0.3219752754296894559, 0.3333333333333333703, 0.3219752754296894559, 0.3333333333333333703, 0.3219752754296894559, 0.3333333333333333703, 0.3219752754296894559, 0.3333333333333333703, 0.3219752754296894559, 0.3333333333333333703, 0.3219752754296894559, 0.3333333333333333703, 0.3219752754296894559, 0.3333333333333333703, 0.3219752754296894559, 0.3333333333333333703, 0.3219752754296894559, 0.3333333333333333703, 0.3219752754296894559, 0.3333333333333333703, 0.3219752754296894559, 0.3333333333333333703, 0.3219752754296894559, 0.3333333333333333703, 0.3219752754296894559, 0.3333333333333333703, 0.3219752754296894559, 0.3333333333333333703, 0.3219752754296894559, 0.3333333333333333703, 0.3219752754296894559, 0.3333333333333333703, 0.3219752754296894559, 0.3333333333333333703, 0.3219752754296894559, 0.3333333333333333703, 0.3219752754296894559, 0.3333333333333333703, 0.3219752754296894559, 0.3333333333333333703, 0.3219752754296894559, 0.3333333333333333703, 0.3219752754296894559, 0.3333333333333333703, 0.3219752754296894559, 0.3333333333333333703, 0.3219752754296894559, 0.3333333333333333703, 0.3219752754296894559, 0.3333333333333333703, 0.3219752754296894559, 0.3333333333333333703, 0.3219752754296894559, 0.3333333333333333703, 0.3219752754296894559, 0.3333333333333333703, 0.3219752754296894559, 0.3333333333333333703, 0.3219752754296894559, 0.3333333333333333703, 0.3219752754296894559, 0.3333333333333333703, 0.3219752754296894559, 0.3333333333333333703, 0.3219752754296894559, 0.3333333333333333703, 0.3219752754296894559, 0.3333333333333333703, 0.3219752754296894559, 0.3333333333333333703, 0.3219752754296894559, 0.3333333333333333703, 0.3219752754296894559, 0.3333333333333333703, 0.3219752754296894559, 0.3333333333333333703, 0.3219752754296894559, 0.3333333333333333703, 0.3219752754296894559, 0.3333333333333333703, 0.3219752754296894559, 0.3333333333333333703, 0.3219752754296894559, 0.3333333333333333703, 0.3219752754296894559, 0.3333333333333333703, 0.3219752754296894559, 0.3333333333333333703, 0.3219752754296894559, 0.3333333333333333703, 0.3219752754296894559, 0.3333333333333333703, 0.3219752754296894559, 0.3333333333333333703, 0.3219752754296894559, 0.3333333333333333703, 0.3219752754296894559, 0.3333333333333333703, 0.3219752754296894559, 0.3333333333333333703, 0.3219752754296894559, 0.3333333333333333703, 0.3219752754296894559, 0.3333333333333333703, 0.3219752754296894559, 0.3333333333333333703, 0.3219752754296894559, 0.3333333333333333703, 0.3219752754296894559, 0.3333333333333333703, 0.3219752754296894559, 0.3333333333333333703, 0.3219752754296894559, 0.3333333333333333703, 0.3219752754296894559, 0.3333333333333333703, 0.3219752754296894559, 0.3333333333333333703, 0.3219752754296894559, 0.3333333333333333703, 0.3219752754296894559, 0.3333333333333333703, 0.3219752754296894559, 0.3333333333333333703, 0.3219752754296894559, 0.3333333333333333703, 0.3219752754296894559, 0.3333333333333333703, 0.3219752754296894559, 0.3333333333333333703, 0.3219752754296894559, 0.3333333333333333703, 0.3219752754296894559, 0.3333333333333333703, 0.3219752754296894559, 0.3333333333333333703),
 ( 0.3333333333333333703, 0.3219752754296894559, 0.3333333333333333703, 0.3219752754296894559, 0.3333333333333333703, 0.3219752754296894559, 0.3333333333333333703, 0.3219752754296894559, 0.3333333333333333703, 0.3219752754296894559, 0.3333333333333333703, 0.3219752754296894559, 0.3333333333333333703, 0.3219752754296894559, 0.3333333333333333703, 0.3219752754296894559, 0.3333333333333333703, 0.3219752754296894559, 0.3333333333333333703, 0.3219752754296894559, 0.3333333333333333703, 0.3219752754296894559, 0.3333333333333333703, 0.3219752754296894559, 0.3333333333333333703, 0.3219752754296894559, 0.3333333333333333703, 0.3219752754296894559, 0.3333333333333333703, 0.3219752754296894559, 0.3333333333333333703, 0.3219752754296894559, 0.3333333333333333703, 0.3219752754296894559, 0.3333333333333333703, 0.3219752754296894559, 0.3333333333333333703, 0.3219752754296894559, 0.3333333333333333703, 0.3219752754296894559, 0.3333333333333333703, 0.3219752754296894559, 0.3333333333333333703, 0.3219752754296894559, 0.3333333333333333703, 0.3219752754296894559, 0.3333333333333333703, 0.3219752754296894559, 0.3333333333333333703, 0.3219752754296894559, 0.3333333333333333703, 0.3219752754296894559, 0.3333333333333333703, 0.3219752754296894559, 0.3333333333333333703, 0.3219752754296894559, 0.3333333333333333703, 0.3219752754296894559, 0.3333333333333333703, 0.3219752754296894559, 0.3333333333333333703, 0.3219752754296894559, 0.3333333333333333703, 0.3219752754296894559, 0.3333333333333333703, 0.3219752754296894559, 0.3333333333333333703, 0.3219752754296894559, 0.3333333333333333703, 0.3219752754296894559, 0.3333333333333333703, 0.3219752754296894559, 0.3333333333333333703, 0.3219752754296894559, 0.3333333333333333703, 0.3219752754296894559, 0.3333333333333333703, 0.3219752754296894559, 0.3333333333333333703, 0.3219752754296894559, 0.3333333333333333703, 0.3219752754296894559, 0.3333333333333333703, 0.3219752754296894559, 0.3333333333333333703, 0.3219752754296894559, 0.3333333333333333703, 0.3219752754296894559, 0.3333333333333333703, 0.3219752754296894559, 0.3333333333333333703, 0.3219752754296894559, 0.3333333333333333703, 0.3219752754296894559, 0.3333333333333333703, 0.3219752754296894559, 0.3333333333333333703, 0.3219752754296894559, 0.3333333333333333703, 0.3219752754296894559, 0.3333333333333333703, 0.3219752754296894559, 0.3333333333333333703, 0.3219752754296894559, 0.3333333333333333703, 0.3219752754296894559, 0.3333333333333333703, 0.3219752754296894559, 0.3333333333333333703, 0.3219752754296894559, 0.3333333333333333703, 0.3219752754296894559, 0.3333333333333333703, 0.3219752754296894559, 0.3333333333333333703, 0.3219752754296894559, 0.3333333333333333703, 0.3219752754296894559, 0.3333333333333333703, 0.3219752754296894559, 0.3333333333333333703, 0.3219752754296894559, 0.3333333333333333703, 0.3219752754296894559, 0.3333333333333333703, 0.3219752754296894559, 0.3333333333333333703, 0.3219752754296894559, 0.3333333333333333703, 0.3219752754296894559, 0.3333333333333333703, 0.3219752754296894559, 0.3333333333333333703, 0.3219752754296894559, 0.3333333333333333703, 0.3219752754296894559, 0.3333333333333333703, 0.3219752754296894559, 0.3333333333333333703, 0.3219752754296894559, 0.3333333333333333703, 0.3219752754296894559, 0.3333333333333333703, 0.3219752754296894559, 0.3333333333333333703, 0.3219752754296894559, 0.3333333333333333703, 0.3219752754296894559, 0.3333333333333333703, 0.3219752754296894559, 0.3333333333333333703, 0.3219752754296894559, 0.3333333333333333703, 0.3219752754296894559, 0.3333333333333333703, 0.3219752754296894559, 0.3333333333333333703, 0.3219752754296894559, 0.3333333333333333703, 0.3219752754296894559, 0.3333333333333333703, 0.3219752754296894559, 0.3333333333333333703, 0.3219752754296894559, 0.3333333333333333703, 0.3219752754296894559, 0.3333333333333333703, 0.3219752754296894559, 0.3333333333333333703, 0.3219752754296894559, 0.3333333333333333703, 0.3219752754296894559, 0.3333333333333333703, 0.3219752754296894559, 0.3333333333333333703, 0.3219752754296894559, 0.3333333333333333703, 0.3219752754296894559, 0.3333333333333333703, 0.3219752754296894559, 0.3333333333333333703, 0.3219752754296894559, 0.3333333333333333703, 0.3219752754296894559, 0.3333333333333333703, 0.3219752754296894559, 0.3333333333333333703, 0.3219752754296894559, 0.3333333333333333703, 0.3219752754296894559, 0.3333333333333333703, 0.3219752754296894559, 0.3333333333333333703),
 ( 1.000000000000000000, 0.9659258262890683122, 1.000000000000000000, 0.9659258262890683122, 1.000000000000000000, 0.9659258262890683122, 1.000000000000000000, 0.9659258262890683122, 1.000000000000000000, 0.9659258262890683122, 1.000000000000000000, 0.9659258262890683122, 1.000000000000000000, 0.9659258262890683122, 1.000000000000000000, 0.9659258262890683122, 1.000000000000000000, 0.9659258262890683122, 1.000000000000000000, 0.9659258262890683122, 1.000000000000000000, 0.9659258262890683122, 1.000000000000000000, 0.9659258262890683122, 1.000000000000000000, 0.9659258262890683122, 1.000000000000000000, 0.9659258262890683122, 1.000000000000000000, 0.9659258262890683122, 1.000000000000000000, 0.9659258262890683122, 1.000000000000000000, 0.9659258262890683122, 1.000000000000000000, 0.9659258262890683122, 1.000000000000000000, 0.9659258262890683122, 1.000000000000000000, 0.9659258262890683122, 1.000000000000000000, 0.9659258262890683122, 1.000000000000000000, 0.9659258262890683122, 1.000000000000000000, 0.9659258262890683122, 1.000000000000000000, 0.9659258262890683122, 1.000000000000000000, 0.9659258262890683122, 1.000000000000000000, 0.9659258262890683122, 1.000000000000000000, 0.9659258262890683122, 1.000000000000000000, 0.9659258262890683122, 1.000000000000000000, 0.9659258262890683122, 1.000000000000000000, 0.9659258262890683122, 1.000000000000000000, 0.9659258262890683122, 1.000000000000000000, 0.9659258262890683122, 1.000000000000000000, 0.9659258262890683122, 1.000000000000000000, 0.9659258262890683122, 1.000000000000000000, 0.9659258262890683122, 1.000000000000000000, 0.9659258262890683122, 1.000000000000000000, 0.9659258262890683122, 1.000000000000000000, 0.9659258262890683122, 1.000000000000000000, 0.9659258262890683122, 1.000000000000000000, 0.9659258262890683122, 1.000000000000000000, 0.9659258262890683122, 1.000000000000000000, 0.9659258262890683122, 1.000000000000000000, 0.9659258262890683122, 1.000000000000000000, 0.9659258262890683122, 1.000000000000000000, 0.9659258262890683122, 1.000000000000000000, 0.9659258262890683122, 1.000000000000000000, 0.9659258262890683122, 1.000000000000000000, 0.9659258262890683122, 1.000000000000000000, 0.9659258262890683122, 1.000000000000000000, 0.9659258262890683122, 1.000000000000000000, 0.9659258262890683122, 1.000000000000000000, 0.9659258262890683122, 1.000000000000000000, 0.9659258262890683122, 1.000000000000000000, 0.9659258262890683122, 1.000000000000000000, 0.9659258262890683122, 1.000000000000000000, 0.9659258262890683122, 1.000000000000000000, 0.9659258262890683122, 1.000000000000000000, 0.9659258262890683122, 1.000000000000000000, 0.9659258262890683122, 1.000000000000000000, 0.9659258262890683122, 1.000000000000000000, 0.9659258262890683122, 1.000000000000000000, 0.9659258262890683122, 1.000000000000000000, 0.9659258262890683122, 1.000000000000000000, 0.9659258262890683122, 1.000000000000000000, 0.9659258262890683122, 1.000000000000000000, 0.9659258262890683122, 1.000000000000000000, 0.9659258262890683122, 1.000000000000000000, 0.9659258262890683122, 1.000000000000000000, 0.9659258262890683122, 1.000000000000000000, 0.9659258262890683122, 1.000000000000000000, 0.9659258262890683122, 1.000000000000000000, 0.9659258262890683122, 1.000000000000000000, 0.9659258262890683122, 1.000000000000000000, 0.9659258262890683122, 1.000000000000000000, 0.9659258262890683122, 1.000000000000000000, 0.9659258262890683122, 1.000000000000000000, 0.9659258262890683122, 1.000000000000000000, 0.9659258262890683122, 1.000000000000000000, 0.9659258262890683122, 1.000000000000000000, 0.9659258262890683122, 1.000000000000000000, 0.9659258262890683122, 1.000000000000000000, 0.9659258262890683122, 1.000000000000000000, 0.9659258262890683122, 1.000000000000000000, 0.9659258262890683122, 1.000000000000000000, 0.9659258262890683122, 1.000000000000000000, 0.9659258262890683122, 1.000000000000000000, 0.9659258262890683122, 1.000000000000000000, 0.9659258262890683122, 1.000000000000000000, 0.9659258262890683122, 1.000000000000000000, 0.9659258262890683122, 1.000000000000000000, 0.9659258262890683122, 1.000000000000000000, 0.9659258262890683122, 1.000000000000000000, 0.9659258262890683122, 1.000000000000000000, 0.9659258262890683122, 1.000000000000000000, 0.9659258262890683122, 1.000000000000000000, 0.9659258262890683122, 1.000000000000000000),
 ( 0.3333333333333333703, 0.3219752754296894559, 0.3333333333333333703, 0.3219752754296894559, 0.3333333333333333703, 0.3219752754296894559, 0.3333333333333333703, 0.3219752754296894559, 0.3333333333333333703, 0.3219752754296894559, 0.3333333333333333703, 0.3219752754296894559, 0.3333333333333333703, 0.3219752754296894559, 0.3333333333333333703, 0.3219752754296894559, 0.3333333333333333703, 0.3219752754296894559, 0.3333333333333333703, 0.3219752754296894559, 0.3333333333333333703, 0.3219752754296894559, 0.3333333333333333703, 0.3219752754296894559, 0.3333333333333333703, 0.3219752754296894559, 0.3333333333333333703, 0.3219752754296894559, 0.3333333333333333703, 0.3219752754296894559, 0.3333333333333333703, 0.3219752754296894559, 0.3333333333333333703, 0.3219752754296894559, 0.3333333333333333703, 0.3219752754296894559, 0.3333333333333333703, 0.3219752754296894559, 0.3333333333333333703, 0.3219752754296894559, 0.3333333333333333703, 0.3219752754296894559, 0.3333333333333333703, 0.3219752754296894559, 0.3333333333333333703, 0.3219752754296894559, 0.3333333333333333703, 0.3219752754296894559, 0.3333333333333333703, 0.3219752754296894559, 0.3333333333333333703, 0.3219752754296894559, 0.3333333333333333703, 0.3219752754296894559, 0.3333333333333333703, 0.3219752754296894559, 0.3333333333333333703, 0.3219752754296894559, 0.3333333333333333703, 0.3219752754296894559, 0.3333333333333333703, 0.3219752754296894559, 0.3333333333333333703, 0.3219752754296894559, 0.3333333333333333703, 0.3219752754296894559, 0.3333333333333333703, 0.3219752754296894559, 0.3333333333333333703, 0.3219752754296894559, 0.3333333333333333703, 0.3219752754296894559, 0.3333333333333333703, 0.3219752754296894559, 0.3333333333333333703, 0.3219752754296894559, 0.3333333333333333703, 0.3219752754296894559, 0.3333333333333333703, 0.3219752754296894559, 0.3333333333333333703, 0.3219752754296894559, 0.3333333333333333703, 0.3219752754296894559, 0.3333333333333333703, 0.3219752754296894559, 0.3333333333333333703, 0.3219752754296894559, 0.3333333333333333703, 0.3219752754296894559, 0.3333333333333333703, 0.3219752754296894559, 0.3333333333333333703, 0.3219752754296894559, 0.3333333333333333703, 0.3219752754296894559, 0.3333333333333333703, 0.3219752754296894559, 0.3333333333333333703, 0.3219752754296894559, 0.3333333333333333703, 0.3219752754296894559, 0.3333333333333333703, 0.3219752754296894559, 0.3333333333333333703, 0.3219752754296894559, 0.3333333333333333703, 0.3219752754296894559, 0.3333333333333333703, 0.3219752754296894559, 0.3333333333333333703, 0.3219752754296894559, 0.3333333333333333703, 0.3219752754296894559, 0.3333333333333333703, 0.3219752754296894559, 0.3333333333333333703, 0.3219752754296894559, 0.3333333333333333703, 0.3219752754296894559, 0.3333333333333333703, 0.3219752754296894559, 0.3333333333333333703, 0.3219752754296894559, 0.3333333333333333703, 0.3219752754296894559, 0.3333333333333333703, 0.3219752754296894559, 0.3333333333333333703, 0.3219752754296894559, 0.3333333333333333703, 0.3219752754296894559, 0.3333333333333333703, 0.3219752754296894559, 0.3333333333333333703, 0.3219752754296894559, 0.3333333333333333703, 0.3219752754296894559, 0.3333333333333333703, 0.3219752754296894559, 0.3333333333333333703, 0.3219752754296894559, 0.3333333333333333703, 0.3219752754296894559, 0.3333333333333333703, 0.3219752754296894559, 0.3333333333333333703, 0.3219752754296894559, 0.3333333333333333703, 0.3219752754296894559, 0.3333333333333333703, 0.3219752754296894559, 0.3333333333333333703, 0.3219752754296894559, 0.3333333333333333703, 0.3219752754296894559, 0.3333333333333333703, 0.3219752754296894559, 0.3333333333333333703, 0.3219752754296894559, 0.3333333333333333703, 0.3219752754296894559, 0.3333333333333333703, 0.3219752754296894559, 0.3333333333333333703, 0.3219752754296894559, 0.3333333333333333703, 0.3219752754296894559, 0.3333333333333333703, 0.3219752754296894559, 0.3333333333333333703, 0.3219752754296894559, 0.3333333333333333703, 0.3219752754296894559, 0.3333333333333333703, 0.3219752754296894559, 0.3333333333333333703, 0.3219752754296894559, 0.3333333333333333703, 0.3219752754296894559, 0.3333333333333333703, 0.3219752754296894559, 0.3333333333333333703, 0.3219752754296894559, 0.3333333333333333703, 0.3219752754296894559, 0.3333333333333333703, 0.3219752754296894559, 0.3333333333333333703, 0.3219752754296894559, 0.3333333333333333703, 0.3219752754296894559, 0.3333333333333333703),
 ( 0.3333333333333333703, 0.3219752754296894559, 0.3333333333333333703, 0.3219752754296894559, 0.3333333333333333703, 0.3219752754296894559, 0.3333333333333333703, 0.3219752754296894559, 0.3333333333333333703, 0.3219752754296894559, 0.3333333333333333703, 0.3219752754296894559, 0.3333333333333333703, 0.3219752754296894559, 0.3333333333333333703, 0.3219752754296894559, 0.3333333333333333703, 0.3219752754296894559, 0.3333333333333333703, 0.3219752754296894559, 0.3333333333333333703, 0.3219752754296894559, 0.3333333333333333703, 0.3219752754296894559, 0.3333333333333333703, 0.3219752754296894559, 0.3333333333333333703, 0.3219752754296894559, 0.3333333333333333703, 0.3219752754296894559, 0.3333333333333333703, 0.3219752754296894559, 0.3333333333333333703, 0.3219752754296894559, 0.3333333333333333703, 0.3219752754296894559, 0.3333333333333333703, 0.3219752754296894559, 0.3333333333333333703, 0.3219752754296894559, 0.3333333333333333703, 0.3219752754296894559, 0.3333333333333333703, 0.3219752754296894559, 0.3333333333333333703, 0.3219752754296894559, 0.3333333333333333703, 0.3219752754296894559, 0.3333333333333333703, 0.3219752754296894559, 0.3333333333333333703, 0.3219752754296894559, 0.3333333333333333703, 0.3219752754296894559, 0.3333333333333333703, 0.3219752754296894559, 0.3333333333333333703, 0.3219752754296894559, 0.3333333333333333703, 0.3219752754296894559, 0.3333333333333333703, 0.3219752754296894559, 0.3333333333333333703, 0.3219752754296894559, 0.3333333333333333703, 0.3219752754296894559, 0.3333333333333333703, 0.3219752754296894559, 0.3333333333333333703, 0.3219752754296894559, 0.3333333333333333703, 0.3219752754296894559, 0.3333333333333333703, 0.3219752754296894559, 0.3333333333333333703, 0.3219752754296894559, 0.3333333333333333703, 0.3219752754296894559, 0.3333333333333333703, 0.3219752754296894559, 0.3333333333333333703, 0.3219752754296894559, 0.3333333333333333703, 0.3219752754296894559, 0.3333333333333333703, 0.3219752754296894559, 0.3333333333333333703, 0.3219752754296894559, 0.3333333333333333703, 0.3219752754296894559, 0.3333333333333333703, 0.3219752754296894559, 0.3333333333333333703, 0.3219752754296894559, 0.3333333333333333703, 0.3219752754296894559, 0.3333333333333333703, 0.3219752754296894559, 0.3333333333333333703, 0.3219752754296894559, 0.3333333333333333703, 0.3219752754296894559, 0.3333333333333333703, 0.3219752754296894559, 0.3333333333333333703, 0.3219752754296894559, 0.3333333333333333703, 0.3219752754296894559, 0.3333333333333333703, 0.3219752754296894559, 0.3333333333333333703, 0.3219752754296894559, 0.3333333333333333703, 0.3219752754296894559, 0.3333333333333333703, 0.3219752754296894559, 0.3333333333333333703, 0.3219752754296894559, 0.3333333333333333703, 0.3219752754296894559, 0.3333333333333333703, 0.3219752754296894559, 0.3333333333333333703, 0.3219752754296894559, 0.3333333333333333703, 0.3219752754296894559, 0.3333333333333333703, 0.3219752754296894559, 0.3333333333333333703, 0.3219752754296894559, 0.3333333333333333703, 0.3219752754296894559, 0.3333333333333333703, 0.3219752754296894559, 0.3333333333333333703, 0.3219752754296894559, 0.3333333333333333703, 0.3219752754296894559, 0.3333333333333333703, 0.3219752754296894559, 0.3333333333333333703, 0.3219752754296894559, 0.3333333333333333703, 0.3219752754296894559, 0.3333333333333333703, 0.3219752754296894559, 0.3333333333333333703, 0.3219752754296894559, 0.3333333333333333703, 0.3219752754296894559, 0.3333333333333333703, 0.3219752754296894559, 0.3333333333333333703, 0.3219752754296894559, 0.3333333333333333703, 0.3219752754296894559, 0.3333333333333333703, 0.3219752754296894559, 0.3333333333333333703, 0.3219752754296894559, 0.3333333333333333703, 0.3219752754296894559, 0.3333333333333333703, 0.3219752754296894559, 0.3333333333333333703, 0.3219752754296894559, 0.3333333333333333703, 0.3219752754296894559, 0.3333333333333333703, 0.3219752754296894559, 0.3333333333333333703, 0.3219752754296894559, 0.3333333333333333703, 0.3219752754296894559, 0.3333333333333333703, 0.3219752754296894559, 0.3333333333333333703, 0.3219752754296894559, 0.3333333333333333703, 0.3219752754296894559, 0.3333333333333333703, 0.3219752754296894559, 0.3333333333333333703, 0.3219752754296894559, 0.3333333333333333703, 0.3219752754296894559, 0.3333333333333333703, 0.3219752754296894559, 0.3333333333333333703, 0.3219752754296894559, 0.3333333333333333703, 0.3219752754296894559, 0.3333333333333333703),
 ( 1.000000000000000000, 0.9659258262890683122, 1.000000000000000000, 0.9659258262890683122, 1.000000000000000000, 0.9659258262890683122, 1.000000000000000000, 0.9659258262890683122, 1.000000000000000000, 0.9659258262890683122, 1.000000000000000000, 0.9659258262890683122, 1.000000000000000000, 0.9659258262890683122, 1.000000000000000000, 0.9659258262890683122, 1.000000000000000000, 0.9659258262890683122, 1.000000000000000000, 0.9659258262890683122, 1.000000000000000000, 0.9659258262890683122, 1.000000000000000000, 0.9659258262890683122, 1.000000000000000000, 0.9659258262890683122, 1.000000000000000000, 0.9659258262890683122, 1.000000000000000000, 0.9659258262890683122, 1.000000000000000000, 0.9659258262890683122, 1.000000000000000000, 0.9659258262890683122, 1.000000000000000000, 0.9659258262890683122, 1.000000000000000000, 0.9659258262890683122, 1.000000000000000000, 0.9659258262890683122, 1.000000000000000000, 0.9659258262890683122, 1.000000000000000000, 0.9659258262890683122, 1.000000000000000000, 0.9659258262890683122, 1.000000000000000000, 0.9659258262890683122, 1.000000000000000000, 0.9659258262890683122, 1.000000000000000000, 0.9659258262890683122, 1.000000000000000000, 0.9659258262890683122, 1.000000000000000000, 0.9659258262890683122, 1.000000000000000000, 0.9659258262890683122, 1.000000000000000000, 0.9659258262890683122, 1.000000000000000000, 0.9659258262890683122, 1.000000000000000000, 0.9659258262890683122, 1.000000000000000000, 0.9659258262890683122, 1.000000000000000000, 0.9659258262890683122, 1.000000000000000000, 0.9659258262890683122, 1.000000000000000000, 0.9659258262890683122, 1.000000000000000000, 0.9659258262890683122, 1.000000000000000000, 0.9659258262890683122, 1.000000000000000000, 0.9659258262890683122, 1.000000000000000000, 0.9659258262890683122, 1.000000000000000000, 0.9659258262890683122, 1.000000000000000000, 0.9659258262890683122, 1.000000000000000000, 0.9659258262890683122, 1.000000000000000000, 0.9659258262890683122, 1.000000000000000000, 0.9659258262890683122, 1.000000000000000000, 0.9659258262890683122, 1.000000000000000000, 0.9659258262890683122, 1.000000000000000000, 0.9659258262890683122, 1.000000000000000000, 0.9659258262890683122, 1.000000000000000000, 0.9659258262890683122, 1.000000000000000000, 0.9659258262890683122, 1.000000000000000000, 0.9659258262890683122, 1.000000000000000000, 0.9659258262890683122, 1.000000000000000000, 0.9659258262890683122, 1.000000000000000000, 0.9659258262890683122, 1.000000000000000000, 0.9659258262890683122, 1.000000000000000000, 0.9659258262890683122, 1.000000000000000000, 0.9659258262890683122, 1.000000000000000000, 0.9659258262890683122, 1.000000000000000000, 0.9659258262890683122, 1.000000000000000000, 0.9659258262890683122, 1.000000000000000000, 0.9659258262890683122, 1.000000000000000000, 0.9659258262890683122, 1.000000000000000000, 0.9659258262890683122, 1.000000000000000000, 0.9659258262890683122, 1.000000000000000000, 0.9659258262890683122, 1.000000000000000000, 0.9659258262890683122, 1.000000000000000000, 0.9659258262890683122, 1.000000000000000000, 0.9659258262890683122, 1.000000000000000000, 0.9659258262890683122, 1.000000000000000000, 0.9659258262890683122, 1.000000000000000000, 0.9659258262890683122, 1.000000000000000000, 0.9659258262890683122, 1.000000000000000000, 0.9659258262890683122, 1.000000000000000000, 0.9659258262890683122, 1.000000000000000000, 0.9659258262890683122, 1.000000000000000000, 0.9659258262890683122, 1.000000000000000000, 0.9659258262890683122, 1.000000000000000000, 0.9659258262890683122, 1.000000000000000000, 0.9659258262890683122, 1.000000000000000000, 0.9659258262890683122, 1.000000000000000000, 0.9659258262890683122, 1.000000000000000000, 0.9659258262890683122, 1.000000000000000000, 0.9659258262890683122, 1.000000000000000000, 0.9659258262890683122, 1.000000000000000000, 0.9659258262890683122, 1.000000000000000000, 0.9659258262890683122, 1.000000000000000000, 0.9659258262890683122, 1.000000000000000000, 0.9659258262890683122, 1.000000000000000000, 0.9659258262890683122, 1.000000000000000000, 0.9659258262890683122, 1.000000000000000000, 0.9659258262890683122, 1.000000000000000000, 0.9659258262890683122, 1.000000000000000000, 0.9659258262890683122, 1.000000000000000000, 0.9659258262890683122, 1.000000000000000000, 0.9659258262890683122, 1.000000000000000000) ) ) 
 REPRESENTATION_ITEM ( '' )  SURFACE ( )  );
#1155=CARTESIAN_POINT ( 'NONE',  ( -52.76711230271184405, 218.4690446883607535, -2.393094931466363651 ) ) ;
#1159=CARTESIAN_POINT ( 'NONE',  ( -50.19419563604517975, 205.4999999999999716, 0.1155267958017633378 ) ) ;
#1165=CARTESIAN_POINT ( 'NONE',  ( -53.56622103062157692, 212.1620413398628671, 8.530955311639223382 ) ) ;
#1192=CARTESIAN_POINT ( 'NONE',  ( -38.31919563604516554, 216.5000000000000000, -0.1155267958017906493 ) ) ;
#1194=CARTESIAN_POINT ( 'NONE',  ( -57.71502896937850124, 215.5714017266979567, -3.350049139982168800 ) ) ;
#1198=CARTESIAN_POINT ( 'NONE',  ( -42.68080436395489841, 205.4999999999999716, -0.1155267958017894420 ) ) ;
#1199=CARTESIAN_POINT ( 'NONE',  ( -51.78497103062156981, 204.4285982733020148, -3.350049139982115509 ) ) ;
#1203=CARTESIAN_POINT ( 'NONE',  ( -45.04836230271183695, 202.5810206699313767, -4.149950860017804111 ) ) ;
#1215=ADVANCED_FACE ( 'NONE', ( #29833 ), #3119, .T. ) ;
#1244=CARTESIAN_POINT ( 'NONE',  ( -50.78794563604517975, 206.7903428501025758, 3.378800118222471838 ) ) ;
#1248=CARTESIAN_POINT ( 'NONE',  ( -50.00372103062157692, 216.5309553116391612, -1.626142955000564383 ) ) ;
#1249=CARTESIAN_POINT ( 'NONE',  ( -30.99627896937850480, 201.4690446883607251, -2.162041339862721845 ) ) ;
#1255=CARTESIAN_POINT ( 'NONE',  ( -47.02752896937850124, 213.3500491399821613, 5.571401726697954970 ) ) ;
#1262=CARTESIAN_POINT ( 'NONE',  ( -49.40997103062156981, 215.5714017266979852, 3.350049139982118618 ) ) ;
#1266=CARTESIAN_POINT ( 'NONE',  ( -38.52455436395490551, 203.6929966515020283, 6.137860380172978303 ) ) ;
#1344=CARTESIAN_POINT ( 'NONE',  ( -51.77752896937850124, 214.3500491399821897, 7.303452534266821949 ) ) ;
#1348=CARTESIAN_POINT ( 'NONE',  ( -39.70461230271183695, 208.6787018382582346, -4.469044688360757966 ) ) ;
#1354=CARTESIAN_POINT ( 'NONE',  ( -48.81622103062156981, 212.1620413398628671, 8.530955311639223382 ) ) ;
#1386=CARTESIAN_POINT ( 'NONE',  ( -37.92336230271182984, 215.6869285224997270, 3.149950860017831200 ) ) ;
#1387=CARTESIAN_POINT ( 'NONE',  ( -49.99627896937850124, 203.4690446883607535, -1.626142955000504209 ) ) ;
#1390=CARTESIAN_POINT ( 'NONE',  ( -41.09747103062157692, 212.3500491399821613, -3.839350919129076445 ) ) ;
#1391=CARTESIAN_POINT ( 'NONE',  ( -62.27455436395490551, 205.1570982666397356, 4.673758765035198159 ) ) ;
#1395=CARTESIAN_POINT ( 'NONE',  ( -48.80877896937850124, 212.1620413398627534, -8.530955311639255356 ) ) ;
#1406=CARTESIAN_POINT ( 'NONE',  ( -34.56622103062155560, 211.6261429550005744, 6.530955311639227823 ) ) ;
#1434=CARTESIAN_POINT ( 'NONE',  ( -59.29836230271182984, 206.0451222850691977, -2.149950860017851184 ) ) ;
#1438=CARTESIAN_POINT ( 'NONE',  ( -41.69122103062155560, 208.3738570449993404, -6.530955311639226935 ) ) ;
#1439=CARTESIAN_POINT ( 'NONE',  ( -52.97247103062156270, 205.6499508600178956, 7.303452534266880569 ) ) ;
#1444=CARTESIAN_POINT ( 'NONE',  ( -49.99627896937850124, 203.4690446883607535, -1.626142955000504209 ) ) ;
#1453=CARTESIAN_POINT ( 'NONE',  ( -56.73288769728823411, 203.5309553116391896, -1.857196546604028997 ) ) ;
#1458=CARTESIAN_POINT ( 'NONE',  ( -35.95163769728824121, 217.4189793300686233, -4.149950860017907139 ) ) ;
#1482=CARTESIAN_POINT ( 'NONE',  ( -62.07663769728824121, 206.0451222850691408, 2.149950860017832532 ) ) ;
#1529=CARTESIAN_POINT ( 'NONE',  ( -53.75669563604516554, 209.8844732041981729, -8.500000000000003553 ) ) ;
#1534=CARTESIAN_POINT ( 'NONE',  ( -47.22544563604517265, 213.3788001182224718, 3.209657149897419348 ) ) ;
#1542=CARTESIAN_POINT ( 'NONE',  ( -53.17038769728823411, 207.6069050685337913, 8.469044688360781947 ) ) ;
#1571=CARTESIAN_POINT ( 'NONE',  ( -34.55877896937849414, 211.6261429550004891, -6.530955311639245586 ) ) ;
#1572=CARTESIAN_POINT ( 'NONE',  ( -57.91294563604515133, 214.6737587650350747, -4.842901733360249317 ) ) ;
#1577=CARTESIAN_POINT ( 'NONE',  ( -45.84747103062156981, 212.3500491399821613, -3.839350919129076445 ) ) ;
#1578=CARTESIAN_POINT ( 'NONE',  ( -57.72247103062156270, 206.6499508600178672, 5.571401726697986057 ) ) ;
#1583=CARTESIAN_POINT ( 'NONE',  ( -51.97544563604517265, 216.3070033484980854, 6.137860380172893926 ) ) ;
#1596=CARTESIAN_POINT ( 'NONE',  ( -33.18080436395490551, 203.5000000000000000, -0.1155267958017335561 ) ) ;
#1624=CARTESIAN_POINT ( 'NONE',  ( -54.35044563604515844, 206.6211998817775566, -3.209657149897419348 ) ) ;
#1628=CARTESIAN_POINT ( 'NONE',  ( -48.42038769728821990, 208.1428034533959703, 6.469044688360770401 ) ) ;
#1629=CARTESIAN_POINT ( 'NONE',  ( -51.58705436395489841, 203.8621396198270475, -6.307003348497942419 ) ) ;
#1635=CARTESIAN_POINT ( 'NONE',  ( -51.38169563604516554, 210.1155267958017703, 6.500000000000000888 ) ) ;
#1644=CARTESIAN_POINT ( 'NONE',  ( -52.57663769728823411, 204.3130714775002730, 3.149950860017883603 ) ) ;
#1648=CARTESIAN_POINT ( 'NONE',  ( -37.13913769728823411, 205.8500491399820760, -7.418979330068584233 ) ) ;
#1672=CARTESIAN_POINT ( 'NONE',  ( -50.39955436395490551, 213.3788001182225003, -3.209657149897400252 ) ) ;
#1719=CARTESIAN_POINT ( 'NONE',  ( -49.60044563604517265, 203.6929966515019430, -6.137860380172892150 ) ) ;
#1723=CARTESIAN_POINT ( 'NONE',  ( -37.32961230271184405, 211.3212981617417938, 4.469044688360757966 ) ) ;
#1762=CARTESIAN_POINT ( 'NONE',  ( -49.60044563604517265, 205.1570982666397072, -4.673758765035155527 ) ) ;
#1766=CARTESIAN_POINT ( 'NONE',  ( -34.76413769728823411, 212.1499508600178387, 3.954877714930865817 ) ) ;
#1767=CARTESIAN_POINT ( 'NONE',  ( -58.51413769728823411, 213.1499508600178672, 5.686928522499718142 ) ) ;
#1771=CARTESIAN_POINT ( 'NONE',  ( -49.60044563604517265, 203.6929966515019430, -6.137860380172892150 ) ) ;
#1809=CARTESIAN_POINT ( 'NONE',  ( -56.72544563604517265, 213.3788001182224718, 3.209657149897419348 ) ) ;
#1814=CARTESIAN_POINT ( 'NONE',  ( -46.24330436395489841, 210.1155267958017134, -6.500000000000000888 ) ) ;
#1815=CARTESIAN_POINT ( 'NONE',  ( -61.28497103062156981, 202.6965474657331185, -4.350049139982091084 ) ) ;
#1819=CARTESIAN_POINT ( 'NONE',  ( -50.39211230271182274, 203.5309553116391612, 1.857196546604092280 ) ) ;
#1828=CARTESIAN_POINT ( 'NONE',  ( -51.38913769728823411, 206.8500491399821044, -5.686928522499717253 ) ) ;
#1833=CARTESIAN_POINT ( 'NONE',  ( -62.47247103062156981, 206.6499508600178672, 5.571401726697986057 ) ) ;
#1857=CARTESIAN_POINT ( 'NONE',  ( -55.94122103062156981, 208.9097554298617752, -4.530955311639240257 ) ) ;
#1903=DIRECTION ( 'NONE',  ( -0.9933043639548644332, 0.1155267958017622554, 0.000000000000000000 ) ) ;
#1904=CARTESIAN_POINT ( 'NONE',  ( -40.29836230271183695, 202.5810206699313767, -4.149950860017804111 ) ) ;
#1907=CARTESIAN_POINT ( 'NONE',  ( -33.76711230271183695, 214.4690446883608104, -1.321298161741814914 ) ) ;
#1942=CARTESIAN_POINT ( 'NONE',  ( -55.34002896937850124, 204.4285982733020433, 3.350049139982171020 ) ) ;
#1946=CARTESIAN_POINT ( 'NONE',  ( -65.63169563604516554, 210.1155267958017703, 4.499999999999996447 ) ) ;
#1947=CARTESIAN_POINT ( 'NONE',  ( -53.96205436395489130, 214.6737587650352168, 4.842901733360204908 ) ) ;
#1952=CARTESIAN_POINT ( 'NONE',  ( -39.11086230271183695, 214.1499508600178387, -7.418979330068641964 ) ) ;
#1992=CARTESIAN_POINT ( 'NONE',  ( -57.51711230271182984, 216.4690446883607535, -1.857196546604089393 ) ) ;
#1994=CARTESIAN_POINT ( 'NONE',  ( -55.53794563604517975, 206.7903428501025758, 3.378800118222471838 ) ) ;
#1998=CARTESIAN_POINT ( 'NONE',  ( -66.82663769728823411, 206.0451222850691408, 2.149950860017832532 ) ) ;
#2000=CARTESIAN_POINT ( 'NONE',  ( -58.51413769728822700, 214.1499508600179240, 7.418979330068584233 ) ) ;
#2004=CARTESIAN_POINT ( 'NONE',  ( -38.31919563604516554, 216.5000000000000000, -0.1155267958017906493 ) ) ;
#2013=CARTESIAN_POINT ( 'NONE',  ( -54.75372103062155560, 216.5309553116392181, -1.626142955000564383 ) ) ;
#2016=CARTESIAN_POINT ( 'NONE',  ( -58.71205436395488420, 214.6737587650352168, 4.842901733360204908 ) ) ;
#2043=CARTESIAN_POINT ( 'NONE',  ( -55.54538769728824832, 211.3212981617418222, -4.469044688360751749 ) ) ;
#2050=( GEOMETRIC_REPRESENTATION_CONTEXT ( 3 ) GLOBAL_UNCERTAINTY_ASSIGNED_CONTEXT ( ( #9714 ) ) GLOBAL_UNIT_ASSIGNED_CONTEXT ( ( #28, #2687, #34711 ) ) REPRESENTATION_CONTEXT ( 'NONE', 'WORKASPACE' ) );
#2094=CARTESIAN_POINT ( 'NONE',  ( -40.49627896937850835, 201.4690446883607251, -2.162041339862721845 ) ) ;
#2097=CARTESIAN_POINT ( 'NONE',  ( -64.64211230271182274, 203.5309553116391612, 1.857196546604092280 ) ) ;
#2100=CARTESIAN_POINT ( 'NONE',  ( -37.73288769728821279, 203.5309553116391612, -1.857196546604028775 ) ) ;
#2129=CARTESIAN_POINT ( 'NONE',  ( -30.40252896937849769, 206.6499508600178387, -5.571401726697954970 ) ) ;
#2130=CARTESIAN_POINT ( 'NONE',  ( -42.67336230271183695, 215.6869285224997270, 3.149950860017831200 ) ) ;
#2135=CARTESIAN_POINT ( 'NONE',  ( -64.64211230271182274, 205.5309553116392465, 1.321298161741817356 ) ) ;
#2136=CARTESIAN_POINT ( 'NONE',  ( -43.07663769728823411, 204.3130714775002730, 3.149950860017883603 ) ) ;
#2140=CARTESIAN_POINT ( 'NONE',  ( -38.51711230271182984, 218.4690446883607535, -2.393094931466363651 ) ) ;
#2153=AXIS2_PLACEMENT_3D ( 'NONE', #3610, #32227, #12521 ) ;
#2178=CARTESIAN_POINT ( 'NONE',  ( -37.13169563604516554, 210.1155267958017703, 4.499999999999996447 ) ) ;
#2181=CARTESIAN_POINT ( 'NONE',  ( -36.14955436395490551, 214.8429017333601792, -4.673758765035196383 ) ) ;
#2182=CARTESIAN_POINT ( 'NONE',  ( -58.31622103062156981, 212.1620413398628671, 8.530955311639223382 ) ) ;
#2187=CARTESIAN_POINT ( 'NONE',  ( -67.21502896937850835, 217.3034525342667962, -4.350049139982195001 ) ) ;
#2197=CARTESIAN_POINT ( 'NONE',  ( -46.44122103062156270, 208.3738570449994256, -6.530955311639227823 ) ) ;
#2201=CARTESIAN_POINT ( 'NONE',  ( -68.40997103062156270, 215.5714017266979852, 3.350049139982118618 ) ) ;
#2227=CARTESIAN_POINT ( 'NONE',  ( -52.77455436395490551, 206.6211998817774997, 3.209657149897401585 ) ) ;
#2277=CARTESIAN_POINT ( 'NONE',  ( -46.43377896937850835, 207.8379586601372750, 8.530955311639258909 ) ) ;
#2280=CARTESIAN_POINT ( 'NONE',  ( -32.18377896937850124, 208.9097554298617183, 4.530955311639234040 ) ) ;
#2284=CARTESIAN_POINT ( 'NONE',  ( -43.27455436395490551, 205.1570982666397356, 4.673758765035198159 ) ) ;
#2322=CARTESIAN_POINT ( 'NONE',  ( -43.06919563604516554, 216.5000000000000000, -0.1155267958017906493 ) ) ;
#2325=CARTESIAN_POINT ( 'NONE',  ( -34.17038769728823411, 208.6787018382581778, 4.469044688360752637 ) ) ;
#2326=CARTESIAN_POINT ( 'NONE',  ( -43.47247103062156981, 206.6499508600178672, 5.571401726697986057 ) ) ;
#2332=CARTESIAN_POINT ( 'NONE',  ( -30.40252896937850124, 205.6499508600178103, -7.303452534266820173 ) ) ;
#2350=CARTESIAN_POINT ( 'NONE',  ( -65.24330436395489130, 210.1155267958017134, -6.500000000000000888 ) ) ;
#2366=CARTESIAN_POINT ( 'NONE',  ( -58.11086230271183695, 213.1499508600178387, -5.686928522499747451 ) ) ;
#2368=CARTESIAN_POINT ( 'NONE',  ( -38.51711230271182984, 214.4690446883608104, -1.321298161741814914 ) ) ;
#2372=CARTESIAN_POINT ( 'NONE',  ( -34.76413769728823411, 213.1499508600178672, 5.686928522499718142 ) ) ;
#2373=CARTESIAN_POINT ( 'NONE',  ( -39.71205436395491262, 216.1378603801730094, 6.307003348497944195 ) ) ;
#2377=CARTESIAN_POINT ( 'NONE',  ( -66.02752896937849414, 214.3500491399821897, 7.303452534266821949 ) ) ;
#2389=CARTESIAN_POINT ( 'NONE',  ( -63.46205436395489841, 214.6737587650352168, 4.842901733360204908 ) ) ;
#2414=CARTESIAN_POINT ( 'NONE',  ( -40.50372103062156981, 214.5309553116392749, -1.090244570138262148 ) ) ;
#2462=CARTESIAN_POINT ( 'NONE',  ( -39.50669563604516554, 209.8844732041981729, -8.500000000000003553 ) ) ;
#2465=CARTESIAN_POINT ( 'NONE',  ( -30.00669563604516554, 209.8844732041982297, -4.499999999999996447 ) ) ;
#2468=CARTESIAN_POINT ( 'NONE',  ( -48.42038769728821990, 208.1428034533959703, 6.469044688360770401 ) ) ;
#2500=CARTESIAN_POINT ( 'NONE',  ( -41.09002896937850124, 204.4285982733020433, 3.350049139982171020 ) ) ;
#2502=( NAMED_UNIT ( * ) SI_UNIT ( $, .STERADIAN. ) SOLID_ANGLE_UNIT ( ) );
#2505=CARTESIAN_POINT ( 'NONE',  ( -32.58705436395489841, 206.7903428501026042, -3.378800118222489157 ) ) ;
#2508=CARTESIAN_POINT ( 'NONE',  ( -39.31622103062156270, 211.6261429550005744, 6.530955311639227823 ) ) ;
#2514=CARTESIAN_POINT ( 'NONE',  ( -33.96502896937850124, 217.3034525342667962, -4.350049139982195001 ) ) ;
#2536=CARTESIAN_POINT ( 'NONE',  ( -65.63913769728823411, 206.8500491399821044, -5.686928522499717253 ) ) ;
#2555=CARTESIAN_POINT ( 'NONE',  ( -35.94419563604516554, 205.4999999999999716, 0.1155267958017633378 ) ) ;
#2558=CARTESIAN_POINT ( 'NONE',  ( -40.50372103062156981, 216.5309553116391612, -1.626142955000564383 ) ) ;
#2559=CARTESIAN_POINT ( 'NONE',  ( -44.65997103062156981, 217.3034525342668815, 4.350049139982096413 ) ) ;
#2563=CARTESIAN_POINT ( 'NONE',  ( -33.96502896937850124, 215.5714017266979567, -3.350049139982168800 ) ) ;
#2575=CARTESIAN_POINT ( 'NONE',  ( -57.92038769728821990, 208.1428034533959703, 6.469044688360770401 ) ) ;
#2598=CARTESIAN_POINT ( 'NONE',  ( -50.00372103062156981, 214.5309553116392749, -1.090244570138262148 ) ) ;
#2645=CARTESIAN_POINT ( 'NONE',  ( -54.15252896937850124, 206.6499508600178387, -5.571401726697954970 ) ) ;
#2648=CARTESIAN_POINT ( 'NONE',  ( -40.30580436395489841, 216.5000000000000000, 0.1155267958017343610 ) ) ;
#2685=CARTESIAN_POINT ( 'NONE',  ( -37.92336230271182984, 215.6869285224997270, 3.149950860017831200 ) ) ;
#2687=( NAMED_UNIT ( * ) PLANE_ANGLE_UNIT ( ) SI_UNIT ( $, .RADIAN. ) );
#2689=CARTESIAN_POINT ( 'NONE',  ( -59.29836230271182984, 206.0451222850691977, -2.149950860017851184 ) ) ;
#2690=CARTESIAN_POINT ( 'NONE',  ( -42.08705436395489841, 205.3262412349647263, -4.842901733360204020 ) ) ;
#2696=CARTESIAN_POINT ( 'NONE',  ( -34.16294563604517265, 216.1378603801729241, -6.307003348498026796 ) ) ;
#2734=CARTESIAN_POINT ( 'NONE',  ( -54.15252896937850124, 206.6499508600178387, -5.571401726697954970 ) ) ;
#2737=CARTESIAN_POINT ( 'NONE',  ( -40.89211230271183695, 205.5309553116392465, 1.321298161741817356 ) ) ;
#2740=CARTESIAN_POINT ( 'NONE',  ( -33.77455436395490551, 205.1570982666397356, 4.673758765035198159 ) ) ;
#2741=CARTESIAN_POINT ( 'NONE',  ( -45.64955436395490551, 216.3070033484980002, -6.137860380172975638 ) ) ;
#2744=CARTESIAN_POINT ( 'NONE',  ( -35.35044563604516554, 205.1570982666397072, -4.673758765035155527 ) ) ;
#2757=CARTESIAN_POINT ( 'NONE',  ( -50.99330436395489841, 210.1155267958017134, -6.500000000000000888 ) ) ;
#2783=CARTESIAN_POINT ( 'NONE',  ( -47.43080436395489841, 205.4999999999999716, -0.1155267958017894420 ) ) ;
#2787=CARTESIAN_POINT ( 'NONE',  ( -69.39955436395486288, 214.8429017333601792, -4.673758765035196383 ) ) ;
#2835=CARTESIAN_POINT ( 'NONE',  ( -39.71205436395490551, 214.6737587650352168, 4.842901733360204908 ) ) ;
#2869=CARTESIAN_POINT ( 'NONE',  ( -42.47544563604516554, 214.8429017333602360, 4.673758765035156415 ) ) ;
#2872=CARTESIAN_POINT ( 'NONE',  ( -58.70461230271184405, 208.6787018382582346, -4.469044688360757966 ) ) ;
#2873=CARTESIAN_POINT ( 'NONE',  ( -38.92038769728823411, 208.1428034533959703, 6.469044688360770401 ) ) ;
#2879=CARTESIAN_POINT ( 'NONE',  ( -56.73288769728824832, 201.5309553116392181, -2.393094931466246855 ) ) ;
#2885=CARTESIAN_POINT ( 'NONE',  ( -47.82663769728823411, 204.3130714775002730, 3.149950860017883603 ) ) ;
#2898=CARTESIAN_POINT ( 'NONE',  ( -58.11830436395490551, 209.8844732041982581, 6.500000000000000888 ) ) ;
#2918=CARTESIAN_POINT ( 'NONE',  ( -54.94419563604517265, 203.5000000000000000, 0.1155267958017914542 ) ) ;
#2921=CARTESIAN_POINT ( 'NONE',  ( -38.71502896937850124, 213.8393509191290889, -2.350049139982142155 ) ) ;
#2924=CARTESIAN_POINT ( 'NONE',  ( -56.53497103062156270, 206.1606490808709111, -2.350049139982163027 ) ) ;
#2925=CARTESIAN_POINT ( 'NONE',  ( -46.63913769728824121, 205.8500491399820760, -7.418979330068584233 ) ) ;
#2930=CARTESIAN_POINT ( 'NONE',  ( -54.74627896937850835, 201.4690446883607251, -2.162041339862721845 ) ) ;
#2942=CARTESIAN_POINT ( 'NONE',  ( -46.04538769728823411, 211.8571965466039444, -6.469044688360768625 ) ) ;
#2969=CARTESIAN_POINT ( 'NONE',  ( -39.31622103062156981, 211.0902445701382533, 4.530955311639240257 ) ) ;
#2973=CARTESIAN_POINT ( 'NONE',  ( -62.67038769728823411, 208.1428034533959703, 6.469044688360770401 ) ) ;
#3024=CARTESIAN_POINT ( 'NONE',  ( -66.82663769728823411, 206.0451222850691408, 2.149950860017832532 ) ) ;
#3059=CARTESIAN_POINT ( 'NONE',  ( -33.76711230271183695, 216.4690446883607535, -1.857196546604089393 ) ) ;
#3061=SHAPE_REPRESENTATION_RELATIONSHIP ( 'NONE' , 'NONE' ,  #6520, #19224 ) ;
#3063=CARTESIAN_POINT ( 'NONE',  ( -53.95461230271185116, 208.6787018382582346, -4.469044688360757966 ) ) ;
#3064=CARTESIAN_POINT ( 'NONE',  ( -34.96205436395488420, 214.6737587650352168, 4.842901733360204908 ) ) ;
#3070=CARTESIAN_POINT ( 'NONE',  ( -65.04538769728823411, 212.3930949314662371, -8.469044688360781947 ) ) ;
#3076=CARTESIAN_POINT ( 'NONE',  ( -41.29538769728821990, 211.8571965466040012, -6.469044688360769513 ) ) ;
#3088=CARTESIAN_POINT ( 'NONE',  ( -53.76413769728823411, 213.1499508600178672, 5.686928522499718142 ) ) ;
#3105=CARTESIAN_POINT ( 'NONE',  ( -48.01711230271182984, 216.4690446883607535, -1.857196546604089393 ) ) ;
#3107=CARTESIAN_POINT ( 'NONE',  ( -30.40252896937850124, 207.6499508600178387, -3.839350919129087547 ) ) ;
#3112=CARTESIAN_POINT ( 'NONE',  ( -64.45163769728823411, 213.9548777149308592, -2.149950860017830756 ) ) ;
#3113=CARTESIAN_POINT ( 'NONE',  ( -38.92038769728823411, 207.6069050685337913, 8.469044688360781947 ) ) ;
#3117=CARTESIAN_POINT ( 'NONE',  ( -63.45461230271184405, 207.6069050685336492, -8.469044688360751749 ) ) ;
#3119=PLANE ( 'NONE',  #34362 ) ;
#3129=CARTESIAN_POINT ( 'NONE',  ( -49.21205436395490551, 214.6737587650352168, 4.842901733360204908 ) ) ;
#3156=CARTESIAN_POINT ( 'NONE',  ( -40.89955436395489841, 213.3788001182225003, -3.209657149897400252 ) ) ;
#3160=CARTESIAN_POINT ( 'NONE',  ( -60.88913769728823411, 206.8500491399821044, -5.686928522499717253 ) ) ;
#3161=CARTESIAN_POINT ( 'NONE',  ( -36.34002896937849414, 202.6965474657332038, 4.350049139982197666 ) ) ;
#3212=CARTESIAN_POINT ( 'NONE',  ( -63.85788769728821990, 214.4690446883608104, 1.321298161741840893 ) ) ;
#3247=CARTESIAN_POINT ( 'NONE',  ( -34.36086230271183695, 213.1499508600178387, -5.686928522499747451 ) ) ;
#3251=CARTESIAN_POINT ( 'NONE',  ( -60.88169563604516554, 210.1155267958017703, 4.499999999999996447 ) ) ;
#3258=CARTESIAN_POINT ( 'NONE',  ( -59.30580436395490551, 218.5000000000000000, 0.1155267958017064944 ) ) ;
#3265=CARTESIAN_POINT ( 'NONE',  ( -45.45163769728822700, 215.6869285224996986, -3.149950860017881382 ) ) ;
#3276=CARTESIAN_POINT ( 'NONE',  ( -57.32663769728823411, 204.3130714775002730, 3.149950860017883603 ) ) ;
#3288=MECHANICAL_DESIGN_GEOMETRIC_PRESENTATION_REPRESENTATION('',(#23270),#32860);
#3292=CARTESIAN_POINT ( 'NONE',  ( -46.43377896937850124, 208.3738570449995109, 6.530955311639247363 ) ) ;
#3294=CARTESIAN_POINT ( 'NONE',  ( -65.43377896937850835, 208.3738570449995109, 6.530955311639247363 ) ) ;
#3297=CARTESIAN_POINT ( 'NONE',  ( -65.63913769728821990, 207.8500491399821613, -3.954877714930864485 ) ) ;
#3298=CARTESIAN_POINT ( 'NONE',  ( -37.93080436395490551, 201.5000000000000000, -0.1155267958017054536 ) ) ;
#3303=CARTESIAN_POINT ( 'NONE',  ( -56.13169563604517265, 210.1155267958018271, 8.500000000000003553 ) ) ;
#3314=CARTESIAN_POINT ( 'NONE',  ( -49.40997103062156981, 215.5714017266979852, 3.350049139982118618 ) ) ;
#3342=CARTESIAN_POINT ( 'NONE',  ( -32.38913769728823411, 207.8500491399821613, -3.954877714930864485 ) ) ;
#3347=CARTESIAN_POINT ( 'NONE',  ( -60.69122103062155560, 208.3738570449993404, -6.530955311639226935 ) ) ;
#3348=CARTESIAN_POINT ( 'NONE',  ( -30.60044563604516199, 203.6929966515019430, -6.137860380172892150 ) ) ;
#3354=CARTESIAN_POINT ( 'NONE',  ( -55.53794563604516554, 205.3262412349647832, 4.842901733360250205 ) ) ;
#3379=AXIS2_PLACEMENT_3D ( 'NONE', #7264, #18463, #30385 ) ;
#3401=CARTESIAN_POINT ( 'NONE',  ( -33.97247103062156270, 206.6499508600178672, 5.571401726697986057 ) ) ;
#3434=CARTESIAN_POINT ( 'NONE',  ( -30.40252896937849769, 206.6499508600178387, -5.571401726697954970 ) ) ;
#3438=CARTESIAN_POINT ( 'NONE',  ( -59.10044563604517265, 206.6211998817775566, -3.209657149897419348 ) ) ;
#3439=CARTESIAN_POINT ( 'NONE',  ( -37.93080436395489841, 203.5000000000000000, -0.1155267958017335561 ) ) ;
#3444=CARTESIAN_POINT ( 'NONE',  ( -65.63913769728821990, 205.8500491399820760, -7.418979330068584233 ) ) ;
#3450=CARTESIAN_POINT ( 'NONE',  ( -35.95163769728823411, 215.6869285224996986, -3.149950860017881382 ) ) ;
#3465=CARTESIAN_POINT ( 'NONE',  ( -55.34747103062156981, 213.3500491399821328, -5.571401726697985168 ) ) ;
#3481=CARTESIAN_POINT ( 'NONE',  ( -56.72544563604516554, 214.8429017333602360, 4.673758765035156415 ) ) ;
#3483=CARTESIAN_POINT ( 'NONE',  ( -30.00669563604516554, 209.8844732041982297, -4.499999999999996447 ) ) ;
#3486=CARTESIAN_POINT ( 'NONE',  ( -61.87872103062156981, 205.4690446883607535, 1.090244570138264368 ) ) ;
#3487=CARTESIAN_POINT ( 'NONE',  ( -64.05580436395490551, 216.5000000000000000, 0.1155267958017343610 ) ) ;
#3491=CARTESIAN_POINT ( 'NONE',  ( -63.25669563604515844, 209.8844732041981729, -8.500000000000003553 ) ) ;
#3504=CARTESIAN_POINT ( 'NONE',  ( -50.20163769728823411, 215.6869285224996986, -3.149950860017881382 ) ) ;
#3534=CARTESIAN_POINT ( 'NONE',  ( -37.13913769728823411, 207.8500491399821613, -3.954877714930864485 ) ) ;
#3538=CARTESIAN_POINT ( 'NONE',  ( -60.09747103062156981, 213.3500491399821328, -5.571401726697985168 ) ) ;
#3540=CARTESIAN_POINT ( 'NONE',  ( -69.20163769728823411, 217.4189793300686233, -4.149950860017907139 ) ) ;
#3546=CARTESIAN_POINT ( 'NONE',  ( -59.49627896937850124, 203.4690446883607535, -1.626142955000504209 ) ) ;
#3554=CARTESIAN_POINT ( 'NONE',  ( -67.02455436395489130, 205.1570982666397640, 4.673758765035199048 ) ) ;
#3592=CARTESIAN_POINT ( 'NONE',  ( -64.84747103062156270, 212.3500491399821613, -3.839350919129076445 ) ) ;
#3610=CARTESIAN_POINT ( 'NONE',  ( -30.00669563604516910, 209.8844732041982013, -6.500000000000000888 ) ) ;
#3626=CARTESIAN_POINT ( 'NONE',  ( -63.65252896937850124, 205.6499508600178103, -7.303452534266820173 ) ) ;
#3631=CARTESIAN_POINT ( 'NONE',  ( -43.06919563604516554, 214.5000000000000284, -0.1155267958017627827 ) ) ;
#3637=CARTESIAN_POINT ( 'NONE',  ( -66.82663769728823411, 202.5810206699313767, 4.149950860017909804 ) ) ;
#3643=CARTESIAN_POINT ( 'NONE',  ( -36.14955436395489841, 214.8429017333601792, -4.673758765035197271 ) ) ;
#3670=CARTESIAN_POINT ( 'NONE',  ( -33.37127896937850124, 216.5309553116392181, 1.626142955000506429 ) ) ;
#3672=CARTESIAN_POINT ( 'NONE',  ( -31.59002896937850124, 206.1606490808709111, 2.350049139982143931 ) ) ;
#3676=CARTESIAN_POINT ( 'NONE',  ( -61.48288769728824121, 205.5309553116392465, -1.321298161741839117 ) ) ;
#3677=CARTESIAN_POINT ( 'NONE',  ( -33.18080436395489841, 201.5000000000000000, -0.1155267958017054536 ) ) ;
#3682=CARTESIAN_POINT ( 'NONE',  ( -61.27752896937849414, 214.3500491399821897, 7.303452534266821949 ) ) ;
#3692=CARTESIAN_POINT ( 'NONE',  ( -36.54538769728823411, 211.8571965466039444, -6.469044688360768625 ) ) ;
#3717=CARTESIAN_POINT ( 'NONE',  ( -67.61086230271183695, 212.1499508600178387, -3.954877714930852495 ) ) ;
#3721=CARTESIAN_POINT ( 'NONE',  ( -54.95163769728823411, 215.6869285224996986, -3.149950860017881382 ) ) ;
#3722=CARTESIAN_POINT ( 'NONE',  ( -34.16294563604517265, 216.1378603801729241, -6.307003348498026796 ) ) ;
#3726=CARTESIAN_POINT ( 'NONE',  ( -58.50669563604516554, 209.8844732041982013, -6.500000000000000888 ) ) ;
#3734=CARTESIAN_POINT ( 'NONE',  ( -69.59747103062156270, 213.3500491399821328, -5.571401726697985168 ) ) ;
#3772=CARTESIAN_POINT ( 'NONE',  ( -68.40997103062156270, 213.8393509191290889, 2.350049139982164359 ) ) ;
#3809=CARTESIAN_POINT ( 'NONE',  ( -31.98586230271182984, 206.8500491399821328, 5.686928522499748340 ) ) ;
#3814=CARTESIAN_POINT ( 'NONE',  ( -45.64211230271183695, 205.5309553116392465, 1.321298161741817356 ) ) ;
#3820=CARTESIAN_POINT ( 'NONE',  ( -49.40997103062157692, 217.3034525342668815, 4.350049139982096413 ) ) ;
#3828=CARTESIAN_POINT ( 'NONE',  ( -31.99330436395490196, 210.1155267958017134, -6.500000000000000888 ) ) ;
#3855=CARTESIAN_POINT ( 'NONE',  ( -31.78794563604516554, 205.3262412349648116, 4.842901733360249317 ) ) ;
#3857=CARTESIAN_POINT ( 'NONE',  ( -33.37127896937850124, 214.5309553116392749, 1.090244570138288127 ) ) ;
#3862=CARTESIAN_POINT ( 'NONE',  ( -50.79538769728824121, 211.3212981617418222, -4.469044688360751749 ) ) ;
#3864=CARTESIAN_POINT ( 'NONE',  ( -69.59747103062156270, 213.3500491399821328, -5.571401726697985168 ) ) ;
#3868=CARTESIAN_POINT ( 'NONE',  ( -40.29836230271183695, 202.5810206699313767, -4.149950860017804111 ) ) ;
#3878=CARTESIAN_POINT ( 'NONE',  ( -32.38913769728823411, 206.8500491399821044, -5.686928522499717253 ) ) ;
#3906=CARTESIAN_POINT ( 'NONE',  ( -62.86086230271182984, 212.1499508600178387, -3.954877714930852495 ) ) ;
#3910=CARTESIAN_POINT ( 'NONE',  ( -49.21205436395490551, 214.6737587650352168, 4.842901733360204908 ) ) ;
#3911=CARTESIAN_POINT ( 'NONE',  ( -69.00372103062157692, 218.5309553116391896, -2.162041339862839084 ) ) ;
#3916=CARTESIAN_POINT ( 'NONE',  ( -61.47544563604515133, 214.8429017333602360, 4.673758765035156415 ) ) ;
#3923=CARTESIAN_POINT ( 'NONE',  ( -62.47247103062156981, 206.6499508600178672, 5.571401726697986057 ) ) ;
#3928=CARTESIAN_POINT ( 'NONE',  ( -34.96205436395489841, 216.1378603801730094, 6.307003348497944195 ) ) ;
#4000=CARTESIAN_POINT ( 'NONE',  ( -55.73586230271182984, 205.8500491399821613, 7.418979330068642852 ) ) ;
#4003=CARTESIAN_POINT ( 'NONE',  ( -48.80877896937850124, 211.0902445701383101, -4.530955311639234040 ) ) ;
#4010=CARTESIAN_POINT ( 'NONE',  ( -46.63913769728824121, 205.8500491399820760, -7.418979330068584233 ) ) ;
#4019=CARTESIAN_POINT ( 'NONE',  ( -33.77455436395489841, 205.1570982666397640, 4.673758765035199048 ) ) ;
#4043=CARTESIAN_POINT ( 'NONE',  ( -40.69419563604516554, 203.5000000000000000, 0.1155267958017914542 ) ) ;
#4044=CARTESIAN_POINT ( 'NONE',  ( -58.70461230271182984, 208.1428034533959135, -6.469044688360754414 ) ) ;
#4048=CARTESIAN_POINT ( 'NONE',  ( -42.87872103062157692, 205.4690446883607535, 1.090244570138264368 ) ) ;
#4049=CARTESIAN_POINT ( 'NONE',  ( -66.82663769728823411, 204.3130714775002730, 3.149950860017883603 ) ) ;
#4053=CARTESIAN_POINT ( 'NONE',  ( -51.77752896937850124, 214.3500491399821897, 7.303452534266821949 ) ) ;
#4068=CARTESIAN_POINT ( 'NONE',  ( -42.48288769728824121, 203.5309553116391612, -1.857196546604028775 ) ) ;
#4097=CARTESIAN_POINT ( 'NONE',  ( -51.18377896937850835, 208.9097554298617183, 4.530955311639234040 ) ) ;
#4101=CARTESIAN_POINT ( 'NONE',  ( -42.87872103062156981, 203.4690446883607535, 1.626142955000567936 ) ) ;
#4102=CARTESIAN_POINT ( 'NONE',  ( -64.45163769728823411, 217.4189793300686233, -4.149950860017907139 ) ) ;
#4107=CARTESIAN_POINT ( 'NONE',  ( -44.45461230271182274, 208.1428034533959135, -6.469044688360754414 ) ) ;
#4115=CARTESIAN_POINT ( 'NONE',  ( -54.95163769728823411, 215.6869285224996986, -3.149950860017881382 ) ) ;
#4119=CARTESIAN_POINT ( 'NONE',  ( -33.18080436395489841, 201.5000000000000000, -0.1155267958017054536 ) ) ;
#4191=CARTESIAN_POINT ( 'NONE',  ( -56.32961230271183695, 212.3930949314663792, 8.469044688360751749 ) ) ;
#4193=CARTESIAN_POINT ( 'NONE',  ( -40.49627896937850835, 205.4690446883607535, -1.090244570138286351 ) ) ;
#4200=CARTESIAN_POINT ( 'NONE',  ( -52.57663769728824832, 202.5810206699313767, 4.149950860017909804 ) ) ;
#4228=CARTESIAN_POINT ( 'NONE',  ( -38.51711230271183695, 216.4690446883607535, -1.857196546604089393 ) ) ;
#4230=CARTESIAN_POINT ( 'NONE',  ( -53.16294563604517265, 214.6737587650350747, -4.842901733360249317 ) ) ;
#4234=CARTESIAN_POINT ( 'NONE',  ( -41.49330436395490551, 210.1155267958017703, -4.499999999999996447 ) ) ;
#4235=CARTESIAN_POINT ( 'NONE',  ( -51.38913769728823411, 206.8500491399821044, -5.686928522499717253 ) ) ;
#4239=CARTESIAN_POINT ( 'NONE',  ( -51.57961230271184405, 212.3930949314663792, 8.469044688360751749 ) ) ;
#4252=CARTESIAN_POINT ( 'NONE',  ( -36.74330436395489841, 210.1155267958017134, -6.500000000000000888 ) ) ;
#4280=CARTESIAN_POINT ( 'NONE',  ( -55.34002896937850124, 206.1606490808709111, 2.350049139982143931 ) ) ;
#4284=CARTESIAN_POINT ( 'NONE',  ( -48.81622103062156270, 211.6261429550005744, 6.530955311639227823 ) ) ;
#4285=CARTESIAN_POINT ( 'NONE',  ( -53.56622103062157692, 212.1620413398628671, 8.530955311639223382 ) ) ;
#4291=CARTESIAN_POINT ( 'NONE',  ( -51.77752896937849414, 213.3500491399821613, 5.571401726697954970 ) ) ;
#4298=CARTESIAN_POINT ( 'NONE',  ( -52.97247103062156981, 206.6499508600178672, 5.571401726697986057 ) ) ;
#4302=CARTESIAN_POINT ( 'NONE',  ( -36.94122103062156981, 207.8379586601371329, -8.530955311639223382 ) ) ;
#4312=CARTESIAN_POINT ( 'NONE',  ( -61.68080436395489841, 203.5000000000000000, -0.1155267958017335561 ) ) ;
#4327=CARTESIAN_POINT ( 'NONE',  ( -50.99330436395489841, 210.1155267958017703, -4.499999999999996447 ) ) ;
#4376=CARTESIAN_POINT ( 'NONE',  ( -56.52752896937850124, 214.3500491399821897, 7.303452534266821949 ) ) ;
#4380=CARTESIAN_POINT ( 'NONE',  ( -42.27752896937850835, 212.3500491399821613, 3.839350919129088435 ) ) ;
#4386=CARTESIAN_POINT ( 'NONE',  ( -51.78497103062156981, 202.6965474657331185, -4.350049139982091084 ) ) ;
#4415=CARTESIAN_POINT ( 'NONE',  ( -38.91294563604516554, 214.6737587650350747, -4.842901733360248429 ) ) ;
#4417=CARTESIAN_POINT ( 'NONE',  ( -59.29836230271183695, 204.3130714775002446, -3.149950860017828091 ) ) ;
#4421=CARTESIAN_POINT ( 'NONE',  ( -43.86830436395490551, 209.8844732041982297, 4.499999999999996447 ) ) ;
#4422=CARTESIAN_POINT ( 'NONE',  ( -63.26413769728824121, 213.1499508600178672, 5.686928522499718142 ) ) ;
#4426=CARTESIAN_POINT ( 'NONE',  ( -49.40252896937850124, 205.6499508600178103, -7.303452534266820173 ) ) ;
#4438=CARTESIAN_POINT ( 'NONE',  ( -39.71205436395490551, 214.6737587650352168, 4.842901733360204908 ) ) ;
#4467=CARTESIAN_POINT ( 'NONE',  ( -55.93377896937850124, 208.9097554298617183, 4.530955311639234040 ) ) ;
#4471=CARTESIAN_POINT ( 'NONE',  ( -48.61830436395490551, 209.8844732041982581, 6.500000000000000888 ) ) ;
#4472=CARTESIAN_POINT ( 'NONE',  ( -52.18080436395490551, 201.5000000000000000, -0.1155267958017054536 ) ) ;
#4477=CARTESIAN_POINT ( 'NONE',  ( -45.64211230271183695, 203.5309553116391612, 1.857196546604092280 ) ) ;
#4488=CARTESIAN_POINT ( 'NONE',  ( -54.35788769728821990, 216.4690446883607535, 1.857196546604031662 ) ) ;
#4492=CARTESIAN_POINT ( 'NONE',  ( -37.33705436395491262, 203.8621396198270475, -6.307003348497942419 ) ) ;
#4518=CARTESIAN_POINT ( 'NONE',  ( -51.58705436395489841, 206.7903428501026042, -3.378800118222489157 ) ) ;
#4559=ORIENTED_EDGE ( 'NONE', *, *, #15916, .F. ) ;
#4564=CARTESIAN_POINT ( 'NONE',  ( -59.89211230271182274, 201.5309553116392181, 2.393094931466368980 ) ) ;
#4568=CARTESIAN_POINT ( 'NONE',  ( -31.39211230271183339, 205.5309553116392465, 1.321298161741817356 ) ) ;
#4603=CARTESIAN_POINT ( 'NONE',  ( -51.77752896937849414, 213.3500491399821613, 5.571401726697954970 ) ) ;
#4606=CARTESIAN_POINT ( 'NONE',  ( -50.00372103062156981, 214.5309553116392749, -1.090244570138262148 ) ) ;
#4607=CARTESIAN_POINT ( 'NONE',  ( -60.69122103062155560, 208.3738570449993404, -6.530955311639226935 ) ) ;
#4611=CARTESIAN_POINT ( 'NONE',  ( -41.09002896937850124, 202.6965474657332038, 4.350049139982197666 ) ) ;
#4648=CARTESIAN_POINT ( 'NONE',  ( -64.64211230271182274, 203.5309553116391896, 1.857196546604092724 ) ) ;
#4650=CARTESIAN_POINT ( 'NONE',  ( -60.09002896937850124, 206.1606490808709111, 2.350049139982143931 ) ) ;
#4651=DIRECTION ( 'NONE',  ( 0.000000000000000000, 0.000000000000000000, 1.000000000000000000 ) ) ;
#4654=CARTESIAN_POINT ( 'NONE',  ( -41.29538769728821990, 211.8571965466039444, -6.469044688360768625 ) ) ;
#4655=CARTESIAN_POINT ( 'NONE',  ( -52.37872103062156981, 201.4690446883607819, 2.162041339862843525 ) ) ;
#4659=CARTESIAN_POINT ( 'NONE',  ( -49.40252896937850124, 206.6499508600178387, -5.571401726697954970 ) ) ;
#4668=CARTESIAN_POINT ( 'NONE',  ( -53.76413769728823411, 213.1499508600178672, 5.686928522499718142 ) ) ;
#4672=CARTESIAN_POINT ( 'NONE',  ( -69.79538769728823411, 211.8571965466039444, -6.469044688360768625 ) ) ;
#4700=CARTESIAN_POINT ( 'NONE',  ( -57.72247103062156270, 207.6499508600178387, 3.839350919129076445 ) ) ;
#4752=CARTESIAN_POINT ( 'NONE',  ( -41.09002896937850124, 202.6965474657332038, 4.350049139982197666 ) ) ;
#4756=CARTESIAN_POINT ( 'NONE',  ( -65.03794563604516554, 205.3262412349647832, 4.842901733360250205 ) ) ;
#4790=CARTESIAN_POINT ( 'NONE',  ( -59.49627896937850124, 203.4690446883607535, -1.626142955000504209 ) ) ;
#4793=CARTESIAN_POINT ( 'NONE',  ( -65.82961230271185116, 211.3212981617417938, 4.469044688360757966 ) ) ;
#4794=CARTESIAN_POINT ( 'NONE',  ( -54.55580436395489841, 216.5000000000000000, 0.1155267958017343610 ) ) ;
#4798=CARTESIAN_POINT ( 'NONE',  ( -30.60044563604516199, 203.6929966515019430, -6.137860380172892150 ) ) ;
#4836=CARTESIAN_POINT ( 'NONE',  ( -61.07961230271182274, 211.8571965466040581, 6.469044688360755302 ) ) ;
#4838=CARTESIAN_POINT ( 'NONE',  ( -57.51711230271184405, 214.4690446883608104, -1.321298161741814914 ) ) ;
#4842=CARTESIAN_POINT ( 'NONE',  ( -67.02455436395489130, 206.6211998817774997, 3.209657149897401585 ) ) ;
#4843=CARTESIAN_POINT ( 'NONE',  ( -59.10788769728823411, 218.4690446883607535, 2.393094931466250408 ) ) ;
#4848=CARTESIAN_POINT ( 'NONE',  ( -43.46502896937849414, 215.5714017266979567, -3.350049139982168800 ) ) ;
#4857=CARTESIAN_POINT ( 'NONE',  ( -53.36830436395489841, 209.8844732041982581, 6.500000000000000888 ) ) ;
#4861=CARTESIAN_POINT ( 'NONE',  ( -65.04538769728824832, 211.8571965466039444, -6.469044688360768625 ) ) ;
#4886=CARTESIAN_POINT ( 'NONE',  ( -61.08705436395490551, 206.7903428501026042, -3.378800118222489157 ) ) ;
#4930=CARTESIAN_POINT ( 'NONE',  ( -47.42336230271184405, 217.4189793300686233, 4.149950860017807663 ) ) ;
#4933=CARTESIAN_POINT ( 'NONE',  ( -38.31919563604515844, 214.5000000000000284, -0.1155267958017627827 ) ) ;
#4936=CARTESIAN_POINT ( 'NONE',  ( -38.32663769728824121, 204.3130714775002730, 3.149950860017883603 ) ) ;
#4972=CARTESIAN_POINT ( 'NONE',  ( -46.63169563604516554, 210.1155267958017703, 6.500000000000000888 ) ) ;
#4976=CARTESIAN_POINT ( 'NONE',  ( -65.03794563604515133, 206.7903428501025758, 3.378800118222471838 ) ) ;
#4977=CARTESIAN_POINT ( 'NONE',  ( -52.37872103062156270, 203.4690446883607535, 1.626142955000567936 ) ) ;
#4981=CARTESIAN_POINT ( 'NONE',  ( -68.80580436395490551, 218.5000000000000000, 0.1155267958017064944 ) ) ;
#4994=DIRECTION ( 'NONE',  ( 0.1155267958017759666, 0.9933043639548631010, -1.378486719154166141E-14 ) ) ;
#5001=FACE_OUTER_BOUND ( 'NONE', #5661, .T. ) ;
#5022=CARTESIAN_POINT ( 'NONE',  ( -64.04836230271183695, 204.3130714775002446, -3.149950860017828091 ) ) ;
#5024=CARTESIAN_POINT ( 'NONE',  ( -41.88169563604517265, 210.1155267958017703, 4.499999999999996447 ) ) ;
#5028=CARTESIAN_POINT ( 'NONE',  ( -36.94122103062157692, 208.3738570449993404, -6.530955311639226935 ) ) ;
#5030=CARTESIAN_POINT ( 'NONE',  ( -60.49330436395489130, 210.1155267958016850, -8.500000000000003553 ) ) ;
#5034=CARTESIAN_POINT ( 'NONE',  ( -66.22544563604516554, 216.3070033484980854, 6.137860380172893926 ) ) ;
#5042=CARTESIAN_POINT ( 'NONE',  ( -42.08705436395489841, 205.3262412349647548, -4.842901733360204908 ) ) ;
#5047=CARTESIAN_POINT ( 'NONE',  ( -66.03497103062157692, 204.4285982733020148, -3.350049139982115509 ) ) ;
#5073=CARTESIAN_POINT ( 'NONE',  ( -53.96205436395491262, 213.2096571498974242, 3.378800118222489601 ) ) ;
#5076=CARTESIAN_POINT ( 'NONE',  ( -66.62872103062152007, 203.4690446883607535, 1.626142955000567936 ) ) ;
#5120=CARTESIAN_POINT ( 'NONE',  ( -43.06919563604516554, 218.5000000000000000, -0.1155267958018185298 ) ) ;
#5123=CARTESIAN_POINT ( 'NONE',  ( -30.60044563604516199, 206.6211998817775566, -3.209657149897419348 ) ) ;
#5126=CARTESIAN_POINT ( 'NONE',  ( -44.46205436395488420, 214.6737587650352168, 4.842901733360204908 ) ) ;
#5157=CARTESIAN_POINT ( 'NONE',  ( -40.29836230271182984, 204.3130714775002446, -3.149950860017828091 ) ) ;
#5161=CARTESIAN_POINT ( 'NONE',  ( -36.34747103062156981, 212.3500491399821613, -3.839350919129076445 ) ) ;
#5163=CARTESIAN_POINT ( 'NONE',  ( -47.43080436395489841, 203.5000000000000000, -0.1155267958017335561 ) ) ;
#5168=CARTESIAN_POINT ( 'NONE',  ( -36.53794563604517265, 203.8621396198271043, 6.307003348498029460 ) ) ;
#5190=CARTESIAN_POINT ( 'NONE',  ( -67.02455436395489130, 205.1570982666397356, 4.673758765035198159 ) ) ;
#5207=CARTESIAN_POINT ( 'NONE',  ( -58.30877896937849414, 211.6261429550004891, -6.530955311639245586 ) ) ;
#5209=CARTESIAN_POINT ( 'NONE',  ( -43.46502896937849414, 213.8393509191290889, -2.350049139982142155 ) ) ;
#5213=CARTESIAN_POINT ( 'NONE',  ( -32.98288769728824121, 203.5309553116391612, -1.857196546604028775 ) ) ;
#5214=CARTESIAN_POINT ( 'NONE',  ( -43.67038769728823411, 207.6069050685337913, 8.469044688360781947 ) ) ;
#5220=CARTESIAN_POINT ( 'NONE',  ( -33.56919563604517265, 216.5000000000000000, -0.1155267958017906493 ) ) ;
#5235=CARTESIAN_POINT ( 'NONE',  ( -67.02455436395489130, 205.1570982666397356, 4.673758765035198159 ) ) ;
#5259=CARTESIAN_POINT ( 'NONE',  ( -42.28497103062156270, 206.1606490808709111, -2.350049139982163027 ) ) ;
#5265=CARTESIAN_POINT ( 'NONE',  ( -68.01413769728823411, 213.1499508600178672, 5.686928522499718142 ) ) ;
#5308=CARTESIAN_POINT ( 'NONE',  ( -44.85044563604516554, 203.6929966515019430, -6.137860380172892150 ) ) ;
#5310=CARTESIAN_POINT ( 'NONE',  ( -36.73586230271183695, 207.8500491399821613, 3.954877714930852495 ) ) ;
#5313=CARTESIAN_POINT ( 'NONE',  ( -47.62872103062154849, 203.4690446883607535, 1.626142955000567936 ) ) ;
#5344=CARTESIAN_POINT ( 'NONE',  ( -30.00669563604516910, 209.8844732041982013, -6.500000000000000888 ) ) ;
#5345=CARTESIAN_POINT ( 'NONE',  ( -40.49627896937849414, 203.4690446883607535, -1.626142955000504209 ) ) ;
#5347=SURFACE_SIDE_STYLE ('',( #31319 ) ) ;
#5349=CARTESIAN_POINT ( 'NONE',  ( -36.54538769728824121, 211.3212981617418222, -4.469044688360751749 ) ) ;
#5350=CARTESIAN_POINT ( 'NONE',  ( -46.04538769728823411, 211.8571965466039444, -6.469044688360768625 ) ) ;
#5355=CARTESIAN_POINT ( 'NONE',  ( -31.39211230271183339, 201.5309553116392181, 2.393094931466368980 ) ) ;
#5371=CARTESIAN_POINT ( 'NONE',  ( -66.43080436395490551, 203.5000000000000000, -0.1155267958017335561 ) ) ;
#5388=CARTESIAN_POINT ( 'NONE',  ( -65.23586230271183695, 206.8500491399821328, 5.686928522499748340 ) ) ;
#5390=CARTESIAN_POINT ( 'NONE',  ( -39.11086230271183695, 212.1499508600178387, -3.954877714930852495 ) ) ;
#5393=CARTESIAN_POINT ( 'NONE',  ( -68.21205436395490551, 213.2096571498974242, 3.378800118222489601 ) ) ;
#5394=CARTESIAN_POINT ( 'NONE',  ( -50.39955436395490551, 216.3070033484980002, -6.137860380172975638 ) ) ;
#5398=CARTESIAN_POINT ( 'NONE',  ( -32.97544563604516554, 214.8429017333602360, 4.673758765035156415 ) ) ;
#5410=CARTESIAN_POINT ( 'NONE',  ( -62.07663769728823411, 204.3130714775002730, 3.149950860017883603 ) ) ;
#5435=CARTESIAN_POINT ( 'NONE',  ( -45.64955436395490551, 213.3788001182225003, -3.209657149897400252 ) ) ;
#5485=CARTESIAN_POINT ( 'NONE',  ( -58.70461230271182984, 208.1428034533959135, -6.469044688360754414 ) ) ;
#5489=CARTESIAN_POINT ( 'NONE',  ( -46.44122103062156270, 208.3738570449993404, -6.530955311639226935 ) ) ;
#5523=CARTESIAN_POINT ( 'NONE',  ( -38.51711230271183695, 216.4690446883607535, -1.857196546604089393 ) ) ;
#5526=CARTESIAN_POINT ( 'NONE',  ( -36.14955436395489841, 213.3788001182225003, -3.209657149897400252 ) ) ;
#5527=CARTESIAN_POINT ( 'NONE',  ( -48.22247103062156270, 206.6499508600178672, 5.571401726697986057 ) ) ;
#5533=CARTESIAN_POINT ( 'NONE',  ( -35.15252896937850124, 205.6499508600178103, -7.303452534266820173 ) ) ;
#5553=CARTESIAN_POINT ( 'NONE',  ( -63.26413769728824121, 213.1499508600178672, 5.686928522499718142 ) ) ;
#5571=CARTESIAN_POINT ( 'NONE',  ( -47.62127896937848703, 216.5309553116392181, 1.626142955000506429 ) ) ;
#5573=CARTESIAN_POINT ( 'NONE',  ( -46.63169563604517265, 210.1155267958017703, 4.499999999999996447 ) ) ;
#5577=CARTESIAN_POINT ( 'NONE',  ( -69.59747103062156270, 212.3500491399821613, -3.839350919129076445 ) ) ;
#5578=CARTESIAN_POINT ( 'NONE',  ( -48.02455436395490551, 203.6929966515020283, 6.137860380172978303 ) ) ;
#5582=CARTESIAN_POINT ( 'NONE',  ( -30.60044563604515488, 205.1570982666397072, -4.673758765035155527 ) ) ;
#5592=CARTESIAN_POINT ( 'NONE',  ( -54.55580436395489841, 216.5000000000000000, 0.1155267958017343610 ) ) ;
#5620=CARTESIAN_POINT ( 'NONE',  ( -45.84747103062156981, 212.3500491399821613, -3.839350919129076445 ) ) ;
#5624=CARTESIAN_POINT ( 'NONE',  ( -67.81622103062156270, 211.6261429550005744, 6.530955311639227823 ) ) ;
#5661=EDGE_LOOP ( 'NONE', ( #4559, #32064, #23894, #12330 ) ) ;
#5677=CARTESIAN_POINT ( 'NONE',  ( -44.85788769728821990, 216.4690446883607535, 1.857196546604031662 ) ) ;
#5708=ORIENTED_EDGE ( 'NONE', *, *, #9030, .F. ) ;
#5712=CARTESIAN_POINT ( 'NONE',  ( -41.88169563604517265, 210.1155267958017703, 6.500000000000000888 ) ) ;
#5716=CARTESIAN_POINT ( 'NONE',  ( -60.68377896937850835, 208.9097554298617183, 4.530955311639234040 ) ) ;
#5717=CARTESIAN_POINT ( 'NONE',  ( -46.24330436395489841, 210.1155267958017134, -6.500000000000000888 ) ) ;
#5723=CARTESIAN_POINT ( 'NONE',  ( -66.23288769728823411, 201.5309553116392181, -2.393094931466246855 ) ) ;
#5729=CARTESIAN_POINT ( 'NONE',  ( -39.71205436395490551, 214.6737587650351884, 4.842901733360205796 ) ) ;
#5741=CARTESIAN_POINT ( 'NONE',  ( -50.99330436395489841, 210.1155267958017134, -6.500000000000000888 ) ) ;
#5761=CARTESIAN_POINT ( 'NONE',  ( -49.60044563604517265, 205.1570982666397072, -4.673758765035155527 ) ) ;
#5763=CARTESIAN_POINT ( 'NONE',  ( -38.12127896937850835, 214.5309553116392749, 1.090244570138288127 ) ) ;
#5767=CARTESIAN_POINT ( 'NONE',  ( -55.74330436395489841, 210.1155267958017703, -4.499999999999996447 ) ) ;
#5768=CARTESIAN_POINT ( 'NONE',  ( -41.69122103062156270, 207.8379586601371329, -8.530955311639223382 ) ) ;
#5773=CARTESIAN_POINT ( 'NONE',  ( -31.78794563604516554, 205.3262412349647832, 4.842901733360250205 ) ) ;
#5785=CARTESIAN_POINT ( 'NONE',  ( -44.65997103062156981, 215.5714017266979852, 3.350049139982118618 ) ) ;
#5812=CARTESIAN_POINT ( 'NONE',  ( -39.90997103062156270, 213.8393509191290889, 2.350049139982164359 ) ) ;
#5816=CARTESIAN_POINT ( 'NONE',  ( -59.10788769728823411, 216.4690446883607535, 1.857196546604031662 ) ) ;
#5866=CARTESIAN_POINT ( 'NONE',  ( -35.15997103062156270, 215.5714017266979852, 3.350049139982118618 ) ) ;
#5901=CARTESIAN_POINT ( 'NONE',  ( -35.15252896937850124, 206.6499508600178387, -5.571401726697954970 ) ) ;
#5905=CARTESIAN_POINT ( 'NONE',  ( -63.85044563604516554, 206.6211998817775566, -3.209657149897419348 ) ) ;
#5906=CARTESIAN_POINT ( 'NONE',  ( -36.34747103062156981, 213.3500491399821328, -5.571401726697985168 ) ) ;
#5912=CARTESIAN_POINT ( 'NONE',  ( -54.75372103062156270, 218.5309553116391896, -2.162041339862839084 ) ) ;
#5917=CARTESIAN_POINT ( 'NONE',  ( -37.53497103062156981, 204.4285982733020148, -3.350049139982115509 ) ) ;
#5929=CARTESIAN_POINT ( 'NONE',  ( -60.69122103062155560, 208.3738570449993404, -6.530955311639226935 ) ) ;
#5947=CARTESIAN_POINT ( 'NONE',  ( -51.38169563604516554, 210.1155267958017703, 6.500000000000000888 ) ) ;
#5950=CARTESIAN_POINT ( 'NONE',  ( -32.38169563604516554, 210.1155267958017703, 4.499999999999996447 ) ) ;
#5954=CARTESIAN_POINT ( 'NONE',  ( -56.73288769728824832, 205.5309553116392465, -1.321298161741839117 ) ) ;
#5955=CARTESIAN_POINT ( 'NONE',  ( -43.47247103062156981, 205.6499508600178956, 7.303452534266880569 ) ) ;
#5960=CARTESIAN_POINT ( 'NONE',  ( -62.26711230271183695, 218.4690446883607535, -2.393094931466363651 ) ) ;
#5971=CARTESIAN_POINT ( 'NONE',  ( -48.81622103062156270, 211.6261429550005744, 6.530955311639227823 ) ) ;
#5999=CARTESIAN_POINT ( 'NONE',  ( -38.52455436395490551, 206.6211998817774997, 3.209657149897401585 ) ) ;
#6003=CARTESIAN_POINT ( 'NONE',  ( -58.51413769728823411, 213.1499508600178672, 5.686928522499718142 ) ) ;
#6004=CARTESIAN_POINT ( 'NONE',  ( -42.07961230271182984, 212.3930949314663792, 8.469044688360751749 ) ) ;
#6015=CARTESIAN_POINT ( 'NONE',  ( -67.22247103062156270, 206.6499508600178672, 5.571401726697986057 ) ) ;
#6049=CARTESIAN_POINT ( 'NONE',  ( -66.23288769728823411, 205.5309553116392465, -1.321298161741839117 ) ) ;
#6086=CARTESIAN_POINT ( 'NONE',  ( -68.00669563604516554, 209.8844732041981729, -8.500000000000003553 ) ) ;
#6089=CARTESIAN_POINT ( 'NONE',  ( -52.56919563604517265, 214.5000000000000284, -0.1155267958017627827 ) ) ;
#6090=CARTESIAN_POINT ( 'NONE',  ( -34.76413769728823411, 213.1499508600178672, 5.686928522499718142 ) ) ;
#6096=CARTESIAN_POINT ( 'NONE',  ( -56.93080436395490551, 201.5000000000000000, -0.1155267958017054536 ) ) ;
#6102=CARTESIAN_POINT ( 'NONE',  ( -39.31622103062156270, 211.6261429550005744, 6.530955311639228711 ) ) ;
#6117=CARTESIAN_POINT ( 'NONE',  ( -54.55580436395489841, 216.5000000000000000, 0.1155267958017343610 ) ) ;
#6133=CARTESIAN_POINT ( 'NONE',  ( -46.82961230271183695, 211.8571965466040581, 6.469044688360755302 ) ) ;
#6135=CARTESIAN_POINT ( 'NONE',  ( -33.56919563604517265, 214.5000000000000284, -0.1155267958017627827 ) ) ;
#6140=CARTESIAN_POINT ( 'NONE',  ( -57.92038769728823411, 208.6787018382581778, 4.469044688360752637 ) ) ;
#6141=CARTESIAN_POINT ( 'NONE',  ( -64.64955436395490551, 214.8429017333601792, -4.673758765035196383 ) ) ;
#6145=CARTESIAN_POINT ( 'NONE',  ( -60.48586230271183695, 205.8500491399821613, 7.418979330068642852 ) ) ;
#6161=CARTESIAN_POINT ( 'NONE',  ( -44.06622103062156981, 211.6261429550005744, 6.530955311639227823 ) ) ;
#6190=CARTESIAN_POINT ( 'NONE',  ( -63.65252896937850124, 207.6499508600178387, -3.839350919129087547 ) ) ;
#6194=CARTESIAN_POINT ( 'NONE',  ( -54.75372103062154849, 216.5309553116391612, -1.626142955000564383 ) ) ;
#6195=CARTESIAN_POINT ( 'NONE',  ( -33.76711230271183695, 218.4690446883607535, -2.393094931466363651 ) ) ;
#6199=CARTESIAN_POINT ( 'NONE',  ( -52.76711230271183695, 216.4690446883607535, -1.857196546604089393 ) ) ;
#6208=CARTESIAN_POINT ( 'NONE',  ( -64.84747103062156270, 213.3500491399821328, -5.571401726697985168 ) ) ;
#6248=CARTESIAN_POINT ( 'NONE',  ( -67.42038769728826253, 208.6787018382581778, 4.469044688360752637 ) ) ;
#6283=CARTESIAN_POINT ( 'NONE',  ( -34.75669563604516554, 209.8844732041982013, -6.500000000000000888 ) ) ;
#6286=CARTESIAN_POINT ( 'NONE',  ( -61.47544563604516554, 213.3788001182224718, 3.209657149897419348 ) ) ;
#6287=CARTESIAN_POINT ( 'NONE',  ( -37.13913769728823411, 206.8500491399821044, -5.686928522499717253 ) ) ;
#6293=CARTESIAN_POINT ( 'NONE',  ( -65.44122103062156270, 207.8379586601371329, -8.530955311639223382 ) ) ;
#6302=CARTESIAN_POINT ( 'NONE',  ( -37.93080436395489841, 203.5000000000000000, -0.1155267958017335561 ) ) ;
#6314=CARTESIAN_POINT ( 'NONE',  ( -60.49330436395489841, 210.1155267958017134, -6.500000000000000888 ) ) ;
#6330=CARTESIAN_POINT ( 'NONE',  ( -49.79836230271183695, 204.3130714775002446, -3.149950860017828091 ) ) ;
#6332=CARTESIAN_POINT ( 'NONE',  ( -30.99627896937850480, 205.4690446883607535, -1.090244570138286351 ) ) ;
#6335=CARTESIAN_POINT ( 'NONE',  ( -58.11830436395491262, 209.8844732041982297, 4.499999999999996447 ) ) ;
#6336=CARTESIAN_POINT ( 'NONE',  ( -65.04538769728824832, 211.8571965466039444, -6.469044688360768625 ) ) ;
#6341=CARTESIAN_POINT ( 'NONE',  ( -64.24627896937850835, 201.4690446883607251, -2.162041339862721845 ) ) ;
#6354=CARTESIAN_POINT ( 'NONE',  ( -51.98288769728821990, 203.5309553116391612, -1.857196546604028775 ) ) ;
#6377=CARTESIAN_POINT ( 'NONE',  ( -67.80877896937849414, 211.0902445701383101, -4.530955311639234040 ) ) ;
#6381=CARTESIAN_POINT ( 'NONE',  ( -57.52455436395488420, 205.1570982666397356, 4.673758765035198159 ) ) ;
#6382=CARTESIAN_POINT ( 'NONE',  ( -30.40252896937850124, 205.6499508600178103, -7.303452534266820173 ) ) ;
#6388=CARTESIAN_POINT ( 'NONE',  ( -57.71502896937850124, 215.5714017266979567, -3.350049139982168800 ) ) ;
#6397=CARTESIAN_POINT ( 'NONE',  ( -67.61830436395489130, 209.8844732041982581, 6.500000000000000888 ) ) ;
#6436=CARTESIAN_POINT ( 'NONE',  ( -32.98288769728824121, 203.5309553116391612, -1.857196546604028775 ) ) ;
#6476=CARTESIAN_POINT ( 'NONE',  ( -66.42336230271182274, 217.4189793300686233, 4.149950860017807663 ) ) ;
#6480=CARTESIAN_POINT ( 'NONE',  ( -51.18377896937850835, 208.9097554298617183, 4.530955311639234040 ) ) ;
#6486=CARTESIAN_POINT ( 'NONE',  ( -60.29538769728823411, 212.3930949314662371, -8.469044688360781947 ) ) ;
#6518=CARTESIAN_POINT ( 'NONE',  ( -33.96502896937850124, 215.5714017266979567, -3.350049139982168800 ) ) ;
#6520=SHAPE_REPRESENTATION ( 'pusher spring', ( #17215 ), #2050 ) ;
#6521=CARTESIAN_POINT ( 'NONE',  ( -64.04836230271183695, 204.3130714775002446, -3.149950860017828091 ) ) ;
#6525=CARTESIAN_POINT ( 'NONE',  ( -55.14955436395491262, 213.3788001182225003, -3.209657149897400252 ) ) ;
#6526=CARTESIAN_POINT ( 'NONE',  ( -36.74330436395489130, 210.1155267958016850, -8.500000000000003553 ) ) ;
#6530=CARTESIAN_POINT ( 'NONE',  ( -64.64211230271182274, 201.5309553116392181, 2.393094931466368980 ) ) ;
#6541=CARTESIAN_POINT ( 'NONE',  ( -38.52455436395488420, 205.1570982666397356, 4.673758765035198159 ) ) ;
#6567=CARTESIAN_POINT ( 'NONE',  ( -32.98288769728823411, 205.5309553116392465, -1.321298161741839117 ) ) ;
#6571=CARTESIAN_POINT ( 'NONE',  ( -55.34747103062156981, 213.3500491399821328, -5.571401726697985168 ) ) ;
#6572=CARTESIAN_POINT ( 'NONE',  ( -36.14211230271182984, 201.5309553116392181, 2.393094931466368980 ) ) ;
#6576=CARTESIAN_POINT ( 'NONE',  ( -62.46502896937850124, 215.5714017266979567, -3.350049139982168800 ) ) ;
#6584=CARTESIAN_POINT ( 'NONE',  ( -62.27455436395490551, 205.1570982666397640, 4.673758765035199048 ) ) ;
#6623=CARTESIAN_POINT ( 'NONE',  ( -67.22247103062156270, 207.6499508600178387, 3.839350919129076445 ) ) ;
#6661=CARTESIAN_POINT ( 'NONE',  ( -66.62127896937849414, 218.5309553116392465, 2.162041339862725842 ) ) ;
#6664=CARTESIAN_POINT ( 'NONE',  ( -39.30877896937850124, 211.0902445701383101, -4.530955311639234040 ) ) ;
#6665=CARTESIAN_POINT ( 'NONE',  ( -33.37872103062156981, 203.4690446883607535, 1.626142955000567936 ) ) ;
#6671=CARTESIAN_POINT ( 'NONE',  ( -45.45163769728823411, 217.4189793300686233, -4.149950860017907139 ) ) ;
#6680=CARTESIAN_POINT ( 'NONE',  ( -32.19122103062156981, 208.3738570449994256, -6.530955311639227823 ) ) ;
#6705=CARTESIAN_POINT ( 'NONE',  ( -32.18377896937850124, 208.3738570449995109, 6.530955311639247363 ) ) ;
#6707=CARTESIAN_POINT ( 'NONE',  ( -62.26711230271183695, 216.4690446883607535, -1.857196546604089393 ) ) ;
#6711=CARTESIAN_POINT ( 'NONE',  ( -52.77455436395490551, 206.6211998817774997, 3.209657149897401585 ) ) ;
#6713=CARTESIAN_POINT ( 'NONE',  ( -34.96205436395489841, 216.1378603801730094, 6.307003348497944195 ) ) ;
#6717=CARTESIAN_POINT ( 'NONE',  ( -56.52752896937850124, 214.3500491399821897, 7.303452534266821949 ) ) ;
#6729=CARTESIAN_POINT ( 'NONE',  ( -32.78497103062156981, 204.4285982733020148, -3.350049139982115509 ) ) ;
#6754=CARTESIAN_POINT ( 'NONE',  ( -33.97247103062156270, 207.6499508600178387, 3.839350919129076445 ) ) ;
#6758=CARTESIAN_POINT ( 'NONE',  ( -52.97247103062156981, 206.6499508600178672, 5.571401726697986057 ) ) ;
#6759=CARTESIAN_POINT ( 'NONE',  ( -68.80580436395490551, 218.5000000000000000, 0.1155267958017064944 ) ) ;
#6763=CARTESIAN_POINT ( 'NONE',  ( -61.07961230271182274, 211.8571965466040297, 6.469044688360755302 ) ) ;
#6770=CARTESIAN_POINT ( 'NONE',  ( -66.43080436395490551, 203.5000000000000000, -0.1155267958017335561 ) ) ;
#6774=CARTESIAN_POINT ( 'NONE',  ( -43.07663769728824121, 202.5810206699313767, 4.149950860017909804 ) ) ;
#6851=CARTESIAN_POINT ( 'NONE',  ( -61.07961230271182984, 212.3930949314663792, 8.469044688360751749 ) ) ;
#6856=CARTESIAN_POINT ( 'NONE',  ( -47.62127896937850124, 214.5309553116392749, 1.090244570138288127 ) ) ;
#6863=CARTESIAN_POINT ( 'NONE',  ( -53.36830436395490551, 209.8844732041983150, 8.500000000000003553 ) ) ;
#6870=CARTESIAN_POINT ( 'NONE',  ( -33.37872103062156981, 203.4690446883607535, 1.626142955000567936 ) ) ;
#6897=CARTESIAN_POINT ( 'NONE',  ( -36.93377896937850124, 208.3738570449995109, 6.530955311639247363 ) ) ;
#6898=CARTESIAN_POINT ( 'NONE',  ( -51.97544563604516554, 214.8429017333602360, 4.673758765035156415 ) ) ;
#6902=( GEOMETRIC_REPRESENTATION_CONTEXT ( 3 ) GLOBAL_UNCERTAINTY_ASSIGNED_CONTEXT ( ( #18444 ) ) GLOBAL_UNIT_ASSIGNED_CONTEXT ( ( #20330, #31871, #2502 ) ) REPRESENTATION_CONTEXT ( 'NONE', 'WORKASPACE' ) );
#6905=CARTESIAN_POINT ( 'NONE',  ( -53.36830436395490551, 209.8844732041982297, 4.499999999999996447 ) ) ;
#6907=CARTESIAN_POINT ( 'NONE',  ( -67.42038769728823411, 208.1428034533959703, 6.469044688360770401 ) ) ;
#6912=CARTESIAN_POINT ( 'NONE',  ( -41.88169563604517265, 210.1155267958018271, 8.500000000000003553 ) ) ;
#6923=CARTESIAN_POINT ( 'NONE',  ( -34.96205436395488420, 214.6737587650352168, 4.842901733360204908 ) ) ;
#6955=CARTESIAN_POINT ( 'NONE',  ( -61.67336230271184405, 213.9548777149308023, 2.149950860017852960 ) ) ;
#6960=CARTESIAN_POINT ( 'NONE',  ( -43.27455436395490551, 205.1570982666397356, 4.673758765035198159 ) ) ;
#6961=CARTESIAN_POINT ( 'NONE',  ( -67.81622103062157692, 212.1620413398628671, 8.530955311639223382 ) ) ;
#6966=CARTESIAN_POINT ( 'NONE',  ( -44.25669563604516554, 209.8844732041982013, -6.500000000000000888 ) ) ;
#6973=CARTESIAN_POINT ( 'NONE',  ( -56.53497103062156270, 204.4285982733020148, -3.350049139982115509 ) ) ;
#6977=CARTESIAN_POINT ( 'NONE',  ( -34.17038769728823411, 207.6069050685337913, 8.469044688360781947 ) ) ;
#7048=ORIENTED_EDGE ( 'NONE', *, *, #33116, .F. ) ;
#7052=CARTESIAN_POINT ( 'NONE',  ( -49.20461230271185116, 207.6069050685336492, -8.469044688360751749 ) ) ;
#7055=CARTESIAN_POINT ( 'NONE',  ( -43.26711230271184405, 214.4690446883608104, -1.321298161741814914 ) ) ;
#7061=CARTESIAN_POINT ( 'NONE',  ( -52.18080436395490551, 201.5000000000000000, -0.1155267958017054536 ) ) ;
#7093=CARTESIAN_POINT ( 'NONE',  ( -44.05877896937849414, 211.6261429550004891, -6.530955311639245586 ) ) ;
#7095=CARTESIAN_POINT ( 'NONE',  ( -52.37127896937850124, 216.5309553116391612, 1.626142955000506873 ) ) ;
#7098=CARTESIAN_POINT ( 'NONE',  ( -41.88913769728823411, 207.8500491399821613, -3.954877714930864485 ) ) ;
#7099=CARTESIAN_POINT ( 'NONE',  ( -52.97247103062156981, 206.6499508600178672, 5.571401726697986057 ) ) ;
#7103=CARTESIAN_POINT ( 'NONE',  ( -44.85044563604516554, 203.6929966515019430, -6.137860380172892150 ) ) ;
#7114=CARTESIAN_POINT ( 'NONE',  ( -37.93080436395489841, 203.5000000000000000, -0.1155267958017335561 ) ) ;
#7140=CARTESIAN_POINT ( 'NONE',  ( -60.88169563604516554, 210.1155267958017703, 4.499999999999996447 ) ) ;
#7144=CARTESIAN_POINT ( 'NONE',  ( -46.04538769728823411, 211.8571965466039444, -6.469044688360768625 ) ) ;
#7145=CARTESIAN_POINT ( 'NONE',  ( -57.12872103062156270, 201.4690446883607819, 2.162041339862843525 ) ) ;
#7151=CARTESIAN_POINT ( 'NONE',  ( -47.81919563604517265, 216.5000000000000000, -0.1155267958017906493 ) ) ;
#7157=CARTESIAN_POINT ( 'NONE',  ( -57.92038769728822700, 208.1428034533959703, 6.469044688360771289 ) ) ;
#7162=CARTESIAN_POINT ( 'NONE',  ( -39.71205436395491262, 216.1378603801730094, 6.307003348497944195 ) ) ;
#7172=CARTESIAN_POINT ( 'NONE',  ( -62.07663769728823411, 204.3130714775002730, 3.149950860017883603 ) ) ;
#7190=CARTESIAN_POINT ( 'NONE',  ( -51.38913769728824121, 207.8500491399821613, -3.954877714930864485 ) ) ;
#7235=CARTESIAN_POINT ( 'NONE',  ( -57.31919563604516554, 218.5000000000000000, -0.1155267958018185298 ) ) ;
#7238=CARTESIAN_POINT ( 'NONE',  ( -50.39211230271182984, 205.5309553116392465, 1.321298161741817356 ) ) ;
#7244=CARTESIAN_POINT ( 'NONE',  ( -48.02455436395490551, 203.6929966515020283, 6.137860380172978303 ) ) ;
#7250=CARTESIAN_POINT ( 'NONE',  ( -32.78497103062156981, 204.4285982733020148, -3.350049139982115509 ) ) ;
#7264=CARTESIAN_POINT ( 'NONE',  ( -31.00000000000003553, 209.9999999999999716, -6.500000000000000888 ) ) ;
#7272=CARTESIAN_POINT ( 'NONE',  ( -34.95461230271183695, 208.1428034533958851, -6.469044688360754414 ) ) ;
#7274=CARTESIAN_POINT ( 'NONE',  ( -57.31919563604516554, 216.5000000000000000, -0.1155267958017906493 ) ) ;
#7277=CARTESIAN_POINT ( 'NONE',  ( -51.19122103062157692, 208.9097554298617752, -4.530955311639240257 ) ) ;
#7278=CARTESIAN_POINT ( 'NONE',  ( -58.90997103062156270, 215.5714017266979852, 3.350049139982118618 ) ) ;
#7282=CARTESIAN_POINT ( 'NONE',  ( -51.38169563604516554, 210.1155267958018271, 8.500000000000003553 ) ) ;
#7294=CARTESIAN_POINT ( 'NONE',  ( -36.34747103062156981, 213.3500491399821328, -5.571401726697985168 ) ) ;
#7322=CARTESIAN_POINT ( 'NONE',  ( -48.61086230271182984, 212.1499508600178387, -3.954877714930852495 ) ) ;
#7327=CARTESIAN_POINT ( 'NONE',  ( -40.70163769728823411, 215.6869285224996986, -3.149950860017881382 ) ) ;
#7328=CARTESIAN_POINT ( 'NONE',  ( -52.57663769728824832, 202.5810206699313767, 4.149950860017909804 ) ) ;
#7334=CARTESIAN_POINT ( 'NONE',  ( -48.80877896937850835, 211.6261429550004607, -6.530955311639245586 ) ) ;
#7342=CARTESIAN_POINT ( 'NONE',  ( -55.74330436395489841, 210.1155267958017134, -6.500000000000000888 ) ) ;
#7347=CARTESIAN_POINT ( 'NONE',  ( -40.30580436395490551, 218.5000000000000000, 0.1155267958017064944 ) ) ;
#7371=CARTESIAN_POINT ( 'NONE',  ( -59.50372103062157692, 214.5309553116392749, -1.090244570138262148 ) ) ;
#7421=CARTESIAN_POINT ( 'NONE',  ( -49.40252896937850124, 205.6499508600178103, -7.303452534266820173 ) ) ;
#7425=CARTESIAN_POINT ( 'NONE',  ( -38.12127896937850835, 214.5309553116392749, 1.090244570138288127 ) ) ;
#7457=CARTESIAN_POINT ( 'NONE',  ( -50.98586230271183695, 206.8500491399821328, 5.686928522499748340 ) ) ;
#7460=CARTESIAN_POINT ( 'NONE',  ( -49.60788769728823411, 214.4690446883608104, 1.321298161741840893 ) ) ;
#7461=CARTESIAN_POINT ( 'NONE',  ( -59.10788769728823411, 216.4690446883607535, 1.857196546604031662 ) ) ;
#7466=CARTESIAN_POINT ( 'NONE',  ( -45.24627896937850835, 201.4690446883607251, -2.162041339862721845 ) ) ;
#7493=ORIENTED_EDGE ( 'NONE', *, *, #24996, .F. ) ;
#7506=CARTESIAN_POINT ( 'NONE',  ( -66.62127896937847993, 216.5309553116392181, 1.626142955000506429 ) ) ;
#7508=CARTESIAN_POINT ( 'NONE',  ( -56.13169563604517265, 210.1155267958017703, 4.499999999999996447 ) ) ;
#7512=CARTESIAN_POINT ( 'NONE',  ( -45.64955436395490551, 214.8429017333601792, -4.673758765035196383 ) ) ;
#7514=CARTESIAN_POINT ( 'NONE',  ( -55.34747103062157692, 214.3500491399821044, -7.303452534266878793 ) ) ;
#7519=CARTESIAN_POINT ( 'NONE',  ( -41.68377896937849414, 208.3738570449995109, 6.530955311639247363 ) ) ;
#7528=CARTESIAN_POINT ( 'NONE',  ( -57.12872103062157692, 203.4690446883607535, 1.626142955000567936 ) ) ;
#7533=CARTESIAN_POINT ( 'NONE',  ( -35.15997103062156270, 217.3034525342668815, 4.350049139982096413 ) ) ;
#7557=CARTESIAN_POINT ( 'NONE',  ( -55.74330436395489841, 210.1155267958017703, -4.499999999999996447 ) ) ;
#7604=CARTESIAN_POINT ( 'NONE',  ( -54.74627896937850835, 201.4690446883607251, -2.162041339862721845 ) ) ;
#7608=CARTESIAN_POINT ( 'NONE',  ( -66.02752896937849414, 213.3500491399821613, 5.571401726697954970 ) ) ;
#7646=CARTESIAN_POINT ( 'NONE',  ( -49.00669563604516554, 209.8844732041982013, -6.500000000000000888 ) ) ;
#7650=CARTESIAN_POINT ( 'NONE',  ( -36.94122103062156981, 208.9097554298617752, -4.530955311639240257 ) ) ;
#7651=CARTESIAN_POINT ( 'NONE',  ( -54.95163769728823411, 215.6869285224996986, -3.149950860017881382 ) ) ;
#7655=CARTESIAN_POINT ( 'NONE',  ( -34.55877896937850124, 212.1620413398627534, -8.530955311639255356 ) ) ;
#7691=CARTESIAN_POINT ( 'NONE',  ( -61.47544563604515844, 214.8429017333602360, 4.673758765035156415 ) ) ;
#7693=CARTESIAN_POINT ( 'NONE',  ( -53.55877896937850124, 211.0902445701383101, -4.530955311639234040 ) ) ;
#7698=CARTESIAN_POINT ( 'NONE',  ( -68.40997103062156270, 213.8393509191290889, 2.350049139982164359 ) ) ;
#7699=CARTESIAN_POINT ( 'NONE',  ( -59.70163769728823411, 217.4189793300686233, -4.149950860017907139 ) ) ;
#7703=CARTESIAN_POINT ( 'NONE',  ( -47.42336230271183695, 215.6869285224997270, 3.149950860017831200 ) ) ;
#7712=CARTESIAN_POINT ( 'NONE',  ( -58.31622103062156270, 211.6261429550005744, 6.530955311639228711 ) ) ;
#7716=CARTESIAN_POINT ( 'NONE',  ( -60.29538769728823411, 211.8571965466039444, -6.469044688360768625 ) ) ;
#7740=CARTESIAN_POINT ( 'NONE',  ( -61.68080436395489841, 205.4999999999999716, -0.1155267958017894420 ) ) ;
#7791=CARTESIAN_POINT ( 'NONE',  ( -47.22544563604517265, 216.3070033484980854, 6.137860380172893926 ) ) ;
#7795=CARTESIAN_POINT ( 'NONE',  ( -34.36086230271182984, 212.1499508600178387, -3.954877714930852495 ) ) ;
#7800=CARTESIAN_POINT ( 'NONE',  ( -38.12872103062154849, 203.4690446883607535, 1.626142955000567936 ) ) ;
#7831=CARTESIAN_POINT ( 'NONE',  ( -48.01711230271182274, 216.4690446883607535, -1.857196546604089393 ) ) ;
#7835=CARTESIAN_POINT ( 'NONE',  ( -37.53497103062155560, 206.1606490808709111, -2.350049139982163027 ) ) ;
#7837=CARTESIAN_POINT ( 'NONE',  ( -54.35788769728821279, 216.4690446883607535, 1.857196546604031662 ) ) ;
#7841=CARTESIAN_POINT ( 'NONE',  ( -37.32961230271184405, 212.3930949314663792, 8.469044688360751749 ) ) ;
#7879=CARTESIAN_POINT ( 'NONE',  ( -64.44419563604516554, 203.5000000000000000, 0.1155267958017914542 ) ) ;
#7881=CARTESIAN_POINT ( 'NONE',  ( -51.38169563604516554, 210.1155267958017703, 4.499999999999996447 ) ) ;
#7885=CARTESIAN_POINT ( 'NONE',  ( -66.62872103062156270, 205.4690446883607535, 1.090244570138264368 ) ) ;
#7887=CARTESIAN_POINT ( 'NONE',  ( -60.09747103062157692, 214.3500491399821044, -7.303452534266878793 ) ) ;
#7892=CARTESIAN_POINT ( 'NONE',  ( -67.41294563604516554, 216.1378603801729241, -6.307003348498026796 ) ) ;
#7901=CARTESIAN_POINT ( 'NONE',  ( -42.87872103062156981, 203.4690446883607535, 1.626142955000567936 ) ) ;
#7905=CARTESIAN_POINT ( 'NONE',  ( -68.21205436395489130, 214.6737587650352168, 4.842901733360204908 ) ) ;
#7931=CARTESIAN_POINT ( 'NONE',  ( -55.34747103062157692, 212.3500491399821613, -3.839350919129076445 ) ) ;
#7933=CARTESIAN_POINT ( 'NONE',  ( -68.21205436395489130, 214.6737587650352168, 4.842901733360204908 ) ) ;
#7977=CARTESIAN_POINT ( 'NONE',  ( -47.62127896937850124, 218.5309553116392465, 2.162041339862725842 ) ) ;
#7980=CARTESIAN_POINT ( 'NONE',  ( -37.52752896937849414, 212.3500491399821613, 3.839350919129088435 ) ) ;
#7984=CARTESIAN_POINT ( 'NONE',  ( -42.48288769728824121, 203.5309553116391612, -1.857196546604028775 ) ) ;
#8014=CARTESIAN_POINT ( 'NONE',  ( -40.89211230271181563, 203.5309553116391612, 1.857196546604092280 ) ) ;
#8019=CARTESIAN_POINT ( 'NONE',  ( -66.02752896937849414, 212.3500491399821613, 3.839350919129088435 ) ) ;
#8020=CARTESIAN_POINT ( 'NONE',  ( -44.85788769728821990, 216.4690446883607535, 1.857196546604031662 ) ) ;
#8025=CARTESIAN_POINT ( 'NONE',  ( -67.02455436395489130, 203.6929966515020283, 6.137860380172978303 ) ) ;
#8045=CARTESIAN_POINT ( 'NONE',  ( -64.25372103062154849, 216.5309553116391612, -1.626142955000564383 ) ) ;
#8065=CARTESIAN_POINT ( 'NONE',  ( -59.69419563604516554, 203.5000000000000000, 0.1155267958017914542 ) ) ;
#8067=CARTESIAN_POINT ( 'NONE',  ( -42.87127896937849414, 214.5309553116392749, 1.090244570138288127 ) ) ;
#8072=CARTESIAN_POINT ( 'NONE',  ( -35.95163769728823411, 215.6869285224996986, -3.149950860017881382 ) ) ;
#8074=CARTESIAN_POINT ( 'NONE',  ( -40.70163769728823411, 217.4189793300686233, -4.149950860017907139 ) ) ;
#8078=CARTESIAN_POINT ( 'NONE',  ( -65.23586230271183695, 205.8500491399821613, 7.418979330068642852 ) ) ;
#8087=CARTESIAN_POINT ( 'NONE',  ( -40.70163769728823411, 215.6869285224996986, -3.149950860017881382 ) ) ;
#8093=CARTESIAN_POINT ( 'NONE',  ( -58.31622103062155560, 211.6261429550005744, 6.530955311639227823 ) ) ;
#8120=CARTESIAN_POINT ( 'NONE',  ( -44.65997103062156981, 213.8393509191290889, 2.350049139982164359 ) ) ;
#8124=CARTESIAN_POINT ( 'NONE',  ( -66.03497103062157692, 204.4285982733020148, -3.350049139982115509 ) ) ;
#8167=CARTESIAN_POINT ( 'NONE',  ( -45.04836230271183695, 202.5810206699313767, -4.149950860017804111 ) ) ;
#8170=CARTESIAN_POINT ( 'NONE',  ( -35.94419563604516554, 205.4999999999999716, 0.1155267958017633378 ) ) ;
#8173=CARTESIAN_POINT ( 'NONE',  ( -46.04538769728823411, 211.8571965466039444, -6.469044688360768625 ) ) ;
#8204=CARTESIAN_POINT ( 'NONE',  ( -45.04836230271183695, 204.3130714775002446, -3.149950860017828091 ) ) ;
#8208=CARTESIAN_POINT ( 'NONE',  ( -39.11830436395489841, 209.8844732041982297, 4.499999999999996447 ) ) ;
#8209=CARTESIAN_POINT ( 'NONE',  ( -39.51413769728823411, 213.1499508600178672, 5.686928522499718142 ) ) ;
#8215=CARTESIAN_POINT ( 'NONE',  ( -37.13169563604516554, 210.1155267958018271, 8.500000000000003553 ) ) ;
#8234=CARTESIAN_POINT ( 'NONE',  ( -69.20163769728823411, 215.6869285224996986, -3.149950860017881382 ) ) ;
#8252=CARTESIAN_POINT ( 'NONE',  ( -57.12127896937849414, 216.5309553116392181, 1.626142955000506429 ) ) ;
#8254=CARTESIAN_POINT ( 'NONE',  ( -43.66294563604516554, 213.2096571498974527, -3.378800118222469617 ) ) ;
#8258=CARTESIAN_POINT ( 'NONE',  ( -39.90997103062156270, 215.5714017266979852, 3.350049139982118618 ) ) ;
#8259=CARTESIAN_POINT ( 'NONE',  ( -49.21205436395490551, 216.1378603801730094, 6.307003348497944195 ) ) ;
#8264=CARTESIAN_POINT ( 'NONE',  ( -33.17336230271182984, 215.6869285224997270, 3.149950860017831200 ) ) ;
#8275=CARTESIAN_POINT ( 'NONE',  ( -65.63913769728823411, 206.8500491399821044, -5.686928522499717253 ) ) ;
#8301=CARTESIAN_POINT ( 'NONE',  ( -43.86830436395490551, 209.8844732041982297, 4.499999999999996447 ) ) ;
#8321=MANIFOLD_SOLID_BREP ( 'Sweep1', #35605 ) ;
#8352=CARTESIAN_POINT ( 'NONE',  ( -54.54836230271182984, 204.3130714775002446, -3.149950860017828091 ) ) ;
#8356=CARTESIAN_POINT ( 'NONE',  ( -41.88913769728823411, 206.8500491399821044, -5.686928522499717253 ) ) ;
#8389=CARTESIAN_POINT ( 'NONE',  ( -48.61086230271182984, 213.1499508600178387, -5.686928522499747451 ) ) ;
#8392=CARTESIAN_POINT ( 'NONE',  ( -39.51413769728823411, 212.1499508600178387, 3.954877714930865817 ) ) ;
#8393=CARTESIAN_POINT ( 'NONE',  ( -45.45163769728822700, 215.6869285224996986, -3.149950860017881382 ) ) ;
#8400=CARTESIAN_POINT ( 'NONE',  ( -32.77752896937849414, 214.3500491399821897, 7.303452534266821949 ) ) ;
#8416=CARTESIAN_POINT ( 'NONE',  ( -65.44122103062157692, 208.3738570449993404, -6.530955311639226935 ) ) ;
#8433=CARTESIAN_POINT ( 'NONE',  ( -52.56919563604516554, 216.5000000000000000, -0.1155267958017906493 ) ) ;
#8435=CARTESIAN_POINT ( 'NONE',  ( -48.21502896937850124, 213.8393509191290889, -2.350049139982142155 ) ) ;
#8438=CARTESIAN_POINT ( 'NONE',  ( -69.00372103062157692, 214.5309553116392749, -1.090244570138262148 ) ) ;
#8439=CARTESIAN_POINT ( 'NONE',  ( -47.62872103062157692, 201.4690446883607819, 2.162041339862843525 ) ) ;
#8444=CARTESIAN_POINT ( 'NONE',  ( -34.16294563604515133, 214.6737587650350747, -4.842901733360249317 ) ) ;
#8455=CARTESIAN_POINT ( 'NONE',  ( -65.24330436395489130, 210.1155267958017134, -6.500000000000000888 ) ) ;
#8481=CARTESIAN_POINT ( 'NONE',  ( -42.48288769728823411, 205.5309553116392465, -1.321298161741839117 ) ) ;
#8486=CARTESIAN_POINT ( 'NONE',  ( -69.00372103062157692, 216.5309553116391612, -1.626142955000564383 ) ) ;
#8535=CARTESIAN_POINT ( 'NONE',  ( -43.07663769728823411, 204.3130714775002730, 3.149950860017883603 ) ) ;
#8569=CARTESIAN_POINT ( 'NONE',  ( -36.73586230271183695, 206.8500491399821328, 5.686928522499748340 ) ) ;
#8572=CARTESIAN_POINT ( 'NONE',  ( -56.13169563604517265, 210.1155267958017703, 4.499999999999996447 ) ) ;
#8573=CARTESIAN_POINT ( 'NONE',  ( -39.71205436395490551, 214.6737587650352168, 4.842901733360204908 ) ) ;
#8579=CARTESIAN_POINT ( 'NONE',  ( -63.06622103062156270, 212.1620413398628671, 8.530955311639223382 ) ) ;
#8595=CARTESIAN_POINT ( 'NONE',  ( -55.54538769728823411, 211.8571965466039444, -6.469044688360768625 ) ) ;
#8614=CARTESIAN_POINT ( 'NONE',  ( -50.39211230271182984, 203.5309553116391896, 1.857196546604092724 ) ) ;
#8617=CARTESIAN_POINT ( 'NONE',  ( -40.69419563604516554, 205.4999999999999716, 0.1155267958017633378 ) ) ;
#8621=CARTESIAN_POINT ( 'NONE',  ( -62.67038769728824121, 208.6787018382581778, 4.469044688360752637 ) ) ;
#8622=CARTESIAN_POINT ( 'NONE',  ( -42.28497103062156270, 202.6965474657331185, -4.350049139982091084 ) ) ;
#8627=CARTESIAN_POINT ( 'NONE',  ( -30.99627896937850124, 203.4690446883607535, -1.626142955000504209 ) ) ;
#8638=CARTESIAN_POINT ( 'NONE',  ( -48.42038769728821990, 208.1428034533959703, 6.469044688360770401 ) ) ;
#8665=CARTESIAN_POINT ( 'NONE',  ( -48.02455436395490551, 206.6211998817774997, 3.209657149897401585 ) ) ;
#8720=CARTESIAN_POINT ( 'NONE',  ( -65.04538769728823411, 211.3212981617418222, -4.469044688360751749 ) ) ;
#8755=CARTESIAN_POINT ( 'NONE',  ( -64.84002896937849414, 202.6965474657332038, 4.350049139982197666 ) ) ;
#8759=CARTESIAN_POINT ( 'NONE',  ( -54.74627896937850835, 205.4690446883607535, -1.090244570138286351 ) ) ;
#8760=CARTESIAN_POINT ( 'NONE',  ( -46.44122103062156270, 208.3738570449993404, -6.530955311639226935 ) ) ;
#8766=CARTESIAN_POINT ( 'NONE',  ( -63.85788769728821990, 218.4690446883607535, 2.393094931466250408 ) ) ;
#8773=CARTESIAN_POINT ( 'NONE',  ( -46.63913769728824121, 206.8500491399821044, -5.686928522499717253 ) ) ;
#8785=CARTESIAN_POINT ( 'NONE',  ( -54.95163769728823411, 215.6869285224996986, -3.149950860017881382 ) ) ;
#8803=CARTESIAN_POINT ( 'NONE',  ( -53.95461230271182984, 208.1428034533958851, -6.469044688360754414 ) ) ;
#8805=CARTESIAN_POINT ( 'NONE',  ( -44.85044563604516554, 206.6211998817775566, -3.209657149897419348 ) ) ;
#8809=CARTESIAN_POINT ( 'NONE',  ( -60.88913769728824121, 207.8500491399821613, -3.954877714930864485 ) ) ;
#8810=CARTESIAN_POINT ( 'NONE',  ( -50.99330436395489841, 210.1155267958016850, -8.500000000000003553 ) ) ;
#8813=CARTESIAN_POINT ( 'NONE',  ( -53.95461230271185116, 207.6069050685336492, -8.469044688360751749 ) ) ;
#8826=CARTESIAN_POINT ( 'NONE',  ( -45.84747103062156981, 213.3500491399821328, -5.571401726697985168 ) ) ;
#8851=CARTESIAN_POINT ( 'NONE',  ( -39.51413769728823411, 212.1499508600178387, 3.954877714930865817 ) ) ;
#8855=CARTESIAN_POINT ( 'NONE',  ( -54.35788769728821279, 216.4690446883607535, 1.857196546604031662 ) ) ;
#8856=CARTESIAN_POINT ( 'NONE',  ( -41.28794563604517265, 203.8621396198271043, 6.307003348498029460 ) ) ;
#8867=CARTESIAN_POINT ( 'NONE',  ( -68.40997103062156270, 215.5714017266979852, 3.350049139982118618 ) ) ;
#8903=CARTESIAN_POINT ( 'NONE',  ( -65.44122103062156270, 208.9097554298617752, -4.530955311639240257 ) ) ;
#8928=ORIENTED_EDGE ( 'NONE', *, *, #21219, .F. ) ;
#8942=CARTESIAN_POINT ( 'NONE',  ( -30.79836230271183695, 204.3130714775002446, -3.149950860017828091 ) ) ;
#8948=CARTESIAN_POINT ( 'NONE',  ( -55.34002896937850124, 206.1606490808709111, 2.350049139982143931 ) ) ;
#8949=CARTESIAN_POINT ( 'NONE',  ( -32.58705436395489841, 205.3262412349647263, -4.842901733360204020 ) ) ;
#8954=CARTESIAN_POINT ( 'NONE',  ( -57.32663769728824121, 202.5810206699313767, 4.149950860017909804 ) ) ;
#8960=CARTESIAN_POINT ( 'NONE',  ( -36.94122103062156981, 208.3738570449994256, -6.530955311639227823 ) ) ;
#8972=CARTESIAN_POINT ( 'NONE',  ( -56.73288769728823411, 203.5309553116391612, -1.857196546604028775 ) ) ;
#8987=CARTESIAN_POINT ( 'NONE',  ( -47.81919563604517265, 216.5000000000000000, -0.1155267958017906493 ) ) ;
#8990=CARTESIAN_POINT ( 'NONE',  ( -66.02752896937849414, 213.3500491399821613, 5.571401726697954970 ) ) ;
#8994=CARTESIAN_POINT ( 'NONE',  ( -60.69122103062156981, 208.9097554298617752, -4.530955311639240257 ) ) ;
#8995=CARTESIAN_POINT ( 'NONE',  ( -65.63913769728823411, 206.8500491399821044, -5.686928522499717253 ) ) ;
#8999=CARTESIAN_POINT ( 'NONE',  ( -54.94419563604517265, 201.5000000000000000, 0.1155267958018195706 ) ) ;
#9010=CARTESIAN_POINT ( 'NONE',  ( -44.85788769728821990, 216.4690446883607535, 1.857196546604031662 ) ) ;
#9030=EDGE_CURVE ( 'NONE', #16114, #29947, #29132, .T. ) ;
#9038=CARTESIAN_POINT ( 'NONE',  ( -64.44419563604517975, 205.4999999999999716, 0.1155267958017633378 ) ) ;
#9042=CARTESIAN_POINT ( 'NONE',  ( -60.49330436395489841, 210.1155267958017134, -6.500000000000000888 ) ) ;
#9043=CARTESIAN_POINT ( 'NONE',  ( -43.86086230271183695, 214.1499508600178387, -7.418979330068641964 ) ) ;
#9048=CARTESIAN_POINT ( 'NONE',  ( -58.11086230271183695, 213.1499508600178387, -5.686928522499747451 ) ) ;
#9057=CARTESIAN_POINT ( 'NONE',  ( -65.44122103062156270, 208.3738570449994256, -6.530955311639227823 ) ) ;
#9095=CARTESIAN_POINT ( 'NONE',  ( -35.55580436395490551, 216.5000000000000000, 0.1155267958017343610 ) ) ;
#9134=CARTESIAN_POINT ( 'NONE',  ( -33.96502896937850124, 215.5714017266979567, -3.350049139982168800 ) ) ;
#9137=CARTESIAN_POINT ( 'NONE',  ( -58.11086230271183695, 212.1499508600178387, -3.954877714930852495 ) ) ;
#9138=CARTESIAN_POINT ( 'NONE',  ( -34.17038769728823411, 208.1428034533959703, 6.469044688360770401 ) ) ;
#9143=CARTESIAN_POINT ( 'NONE',  ( -54.55580436395489841, 218.5000000000000000, 0.1155267958017064944 ) ) ;
#9148=CARTESIAN_POINT ( 'NONE',  ( -41.49330436395490551, 210.1155267958017134, -6.500000000000000888 ) ) ;
#9160=CARTESIAN_POINT ( 'NONE',  ( -54.35788769728821279, 216.4690446883607535, 1.857196546604031662 ) ) ;
#9176=CARTESIAN_POINT ( 'NONE',  ( -45.44419563604516554, 203.5000000000000000, 0.1155267958017914542 ) ) ;
#9177=CARTESIAN_POINT ( 'NONE',  ( -63.85044563604516554, 205.1570982666397072, -4.673758765035155527 ) ) ;
#9181=CARTESIAN_POINT ( 'NONE',  ( -60.09747103062157692, 212.3500491399821613, -3.839350919129076445 ) ) ;
#9182=CARTESIAN_POINT ( 'NONE',  ( -33.37872103062156981, 201.4690446883607819, 2.162041339862843525 ) ) ;
#9187=CARTESIAN_POINT ( 'NONE',  ( -59.10044563604517265, 203.6929966515019430, -6.137860380172892150 ) ) ;
#9200=CARTESIAN_POINT ( 'NONE',  ( -49.60788769728823411, 216.4690446883607535, 1.857196546604031662 ) ) ;
#9223=CARTESIAN_POINT ( 'NONE',  ( -34.36830436395490551, 209.8844732041982297, 4.499999999999996447 ) ) ;
#9227=CARTESIAN_POINT ( 'NONE',  ( -62.86830436395490551, 209.8844732041982581, 6.500000000000000888 ) ) ;
#9228=CARTESIAN_POINT ( 'NONE',  ( -66.43080436395490551, 201.5000000000000000, -0.1155267958017054536 ) ) ;
#9233=CARTESIAN_POINT ( 'NONE',  ( -61.67336230271183695, 215.6869285224997270, 3.149950860017831200 ) ) ;
#9283=CARTESIAN_POINT ( 'NONE',  ( -36.74330436395489841, 210.1155267958017134, -6.500000000000000888 ) ) ;
#9309=STYLED_ITEM ( 'NONE', ( #11413 ), #19224 ) ;
#9321=CARTESIAN_POINT ( 'NONE',  ( -65.03794563604515133, 203.8621396198271043, 6.307003348498029460 ) ) ;
#9324=CARTESIAN_POINT ( 'NONE',  ( -62.06919563604516554, 214.5000000000000284, -0.1155267958017627827 ) ) ;
#9325=CARTESIAN_POINT ( 'NONE',  ( -32.19122103062156981, 208.3738570449993404, -6.530955311639226935 ) ) ;
#9330=CARTESIAN_POINT ( 'NONE',  ( -62.86830436395490551, 209.8844732041983150, 8.500000000000003553 ) ) ;
#9365=CARTESIAN_POINT ( 'NONE',  ( -34.16294563604515844, 214.6737587650350747, -4.842901733360248429 ) ) ;
#9367=CARTESIAN_POINT ( 'NONE',  ( -68.00669563604516554, 209.8844732041982013, -6.500000000000000888 ) ) ;
#9370=CARTESIAN_POINT ( 'NONE',  ( -55.34747103062157692, 212.3500491399821613, -3.839350919129076445 ) ) ;
#9371=CARTESIAN_POINT ( 'NONE',  ( -67.81622103062156270, 211.6261429550005744, 6.530955311639227823 ) ) ;
#9376=CARTESIAN_POINT ( 'NONE',  ( -52.56919563604517265, 218.5000000000000000, -0.1155267958018185298 ) ) ;
#9388=CARTESIAN_POINT ( 'NONE',  ( -56.13913769728823411, 206.8500491399821044, -5.686928522499717253 ) ) ;
#9413=CARTESIAN_POINT ( 'NONE',  ( -35.35788769728823411, 214.4690446883608104, 1.321298161741840893 ) ) ;
#9418=CARTESIAN_POINT ( 'NONE',  ( -61.08705436395488420, 205.3262412349647263, -4.842901733360204020 ) ) ;
#9419=CARTESIAN_POINT ( 'NONE',  ( -31.98586230271182984, 205.8500491399821613, 7.418979330068642852 ) ) ;
#9424=CARTESIAN_POINT ( 'NONE',  ( -56.52752896937850124, 213.3500491399821613, 5.571401726697954970 ) ) ;
#9430=CARTESIAN_POINT ( 'NONE',  ( -63.65997103062156981, 215.5714017266979852, 3.350049139982118618 ) ) ;
#9470=CARTESIAN_POINT ( 'NONE',  ( -64.05580436395490551, 214.5000000000000284, 0.1155267958017899832 ) ) ;
#9510=CARTESIAN_POINT ( 'NONE',  ( -31.19419563604516910, 203.5000000000000000, 0.1155267958017914542 ) ) ;
#9514=CARTESIAN_POINT ( 'NONE',  ( -48.01711230271184405, 214.4690446883608104, -1.321298161741814914 ) ) ;
#9521=CARTESIAN_POINT ( 'NONE',  ( -46.44122103062156981, 207.8379586601371329, -8.530955311639223382 ) ) ;
#9551=CARTESIAN_POINT ( 'NONE',  ( -32.57961230271183695, 211.8571965466040581, 6.469044688360755302 ) ) ;
#9553=CARTESIAN_POINT ( 'NONE',  ( -62.66294563604517975, 214.6737587650350747, -4.842901733360249317 ) ) ;
#9556=CARTESIAN_POINT ( 'NONE',  ( -50.99330436395489841, 210.1155267958017703, -4.499999999999996447 ) ) ;
#9557=CARTESIAN_POINT ( 'NONE',  ( -35.55580436395489130, 218.5000000000000000, 0.1155267958017064944 ) ) ;
#9561=CARTESIAN_POINT ( 'NONE',  ( -61.87127896937851546, 218.5309553116392465, 2.162041339862725842 ) ) ;
#9573=CARTESIAN_POINT ( 'NONE',  ( -33.77455436395490551, 205.1570982666397356, 4.673758765035198159 ) ) ;
#9601=CARTESIAN_POINT ( 'NONE',  ( -64.64211230271182274, 205.5309553116392465, 1.321298161741817356 ) ) ;
#9605=CARTESIAN_POINT ( 'NONE',  ( -60.29538769728823411, 211.8571965466039444, -6.469044688360768625 ) ) ;
#9606=CARTESIAN_POINT ( 'NONE',  ( -68.60788769728823411, 218.4690446883607535, 2.393094931466250408 ) ) ;
#9612=CARTESIAN_POINT ( 'NONE',  ( -59.69419563604516554, 203.5000000000000000, 0.1155267958017914542 ) ) ;
#9622=CARTESIAN_POINT ( 'NONE',  ( -32.98288769728823411, 201.5309553116392181, -2.393094931466246855 ) ) ;
#9696=CARTESIAN_POINT ( 'NONE',  ( -58.11086230271183695, 214.1499508600178387, -7.418979330068641964 ) ) ;
#9700=CARTESIAN_POINT ( 'NONE',  ( -40.89211230271183695, 205.5309553116392465, 1.321298161741817356 ) ) ;
#9701=CARTESIAN_POINT ( 'NONE',  ( -33.57663769728823411, 204.3130714775002730, 3.149950860017883603 ) ) ;
#9707=CARTESIAN_POINT ( 'NONE',  ( -49.60788769728823411, 218.4690446883607535, 2.393094931466250408 ) ) ;
#9714=UNCERTAINTY_MEASURE_WITH_UNIT (LENGTH_MEASURE( 1.000000000000000082E-05 ), #28, 'distance_accuracy_value', 'NONE');
#9742=CARTESIAN_POINT ( 'NONE',  ( -35.15252896937850124, 206.6499508600178387, -5.571401726697954970 ) ) ;
#9743=CARTESIAN_POINT ( 'NONE',  ( -60.09002896937850124, 204.4285982733020433, 3.350049139982171020 ) ) ;
#9746=CARTESIAN_POINT ( 'NONE',  ( -43.47247103062156981, 207.6499508600178387, 3.839350919129076445 ) ) ;
#9747=CARTESIAN_POINT ( 'NONE',  ( -36.94122103062156981, 207.8379586601371329, -8.530955311639223382 ) ) ;
#9751=CARTESIAN_POINT ( 'NONE',  ( -39.70461230271183695, 207.6069050685336492, -8.469044688360751749 ) ) ;
#9761=CARTESIAN_POINT ( 'NONE',  ( -35.35788769728823411, 216.4690446883607535, 1.857196546604031662 ) ) ;
#9786=CARTESIAN_POINT ( 'NONE',  ( -62.06919563604516554, 214.5000000000000284, -0.1155267958017627827 ) ) ;
#9790=CARTESIAN_POINT ( 'NONE',  ( -47.43080436395489841, 203.5000000000000000, -0.1155267958017335561 ) ) ;
#9791=CARTESIAN_POINT ( 'NONE',  ( -65.44122103062156270, 207.8379586601371329, -8.530955311639223382 ) ) ;
#9795=CARTESIAN_POINT ( 'NONE',  ( -39.70461230271183695, 208.1428034533959135, -6.469044688360754414 ) ) ;
#9803=CARTESIAN_POINT ( 'NONE',  ( -50.59747103062156270, 213.3500491399821328, -5.571401726697985168 ) ) ;
#9807=CARTESIAN_POINT ( 'NONE',  ( -37.93080436395490551, 201.5000000000000000, -0.1155267958017054536 ) ) ;
#9880=CARTESIAN_POINT ( 'NONE',  ( -52.56919563604517265, 218.5000000000000000, -0.1155267958018185298 ) ) ;
#9883=CARTESIAN_POINT ( 'NONE',  ( -43.86086230271183695, 212.1499508600178387, -3.954877714930852495 ) ) ;
#9889=CARTESIAN_POINT ( 'NONE',  ( -44.06622103062156270, 212.1620413398628671, 8.530955311639223382 ) ) ;
#9919=CARTESIAN_POINT ( 'NONE',  ( -38.12127896937849414, 216.5309553116392181, 1.626142955000506429 ) ) ;
#9920=CARTESIAN_POINT ( 'NONE',  ( -58.30877896937847993, 211.6261429550004607, -6.530955311639245586 ) ) ;
#9924=CARTESIAN_POINT ( 'NONE',  ( -43.07663769728824121, 206.0451222850691408, 2.149950860017832532 ) ) ;
#9926=CARTESIAN_POINT ( 'NONE',  ( -57.92038769728821990, 208.1428034533959703, 6.469044688360770401 ) ) ;
#9931=CARTESIAN_POINT ( 'NONE',  ( -46.63169563604517265, 210.1155267958018271, 8.500000000000003553 ) ) ;
#9943=CARTESIAN_POINT ( 'NONE',  ( -40.10788769728823411, 216.4690446883607535, 1.857196546604031662 ) ) ;
#9970=CARTESIAN_POINT ( 'NONE',  ( -49.60044563604517265, 206.6211998817775566, -3.209657149897419348 ) ) ;
#9974=CARTESIAN_POINT ( 'NONE',  ( -51.19122103062155560, 208.3738570449993404, -6.530955311639226935 ) ) ;
#9975=CARTESIAN_POINT ( 'NONE',  ( -34.55877896937850124, 212.1620413398627534, -8.530955311639255356 ) ) ;
#9980=CARTESIAN_POINT ( 'NONE',  ( -51.57961230271182274, 211.8571965466040297, 6.469044688360755302 ) ) ;
#9987=CARTESIAN_POINT ( 'NONE',  ( -59.70163769728823411, 215.6869285224996986, -3.149950860017881382 ) ) ;
#9991=CARTESIAN_POINT ( 'NONE',  ( -41.69122103062156270, 207.8379586601371329, -8.530955311639223382 ) ) ;
#10001=CARTESIAN_POINT ( 'NONE',  ( -62.67038769728823411, 208.1428034533959703, 6.469044688360770401 ) ) ;
#10016=CARTESIAN_POINT ( 'NONE',  ( -53.36830436395490551, 209.8844732041982297, 4.499999999999996447 ) ) ;
#10068=CARTESIAN_POINT ( 'NONE',  ( -58.70461230271184405, 207.6069050685336492, -8.469044688360751749 ) ) ;
#10073=CARTESIAN_POINT ( 'NONE',  ( -49.20461230271185116, 208.6787018382582346, -4.469044688360757966 ) ) ;
#10080=CARTESIAN_POINT ( 'NONE',  ( -53.96205436395491262, 216.1378603801730094, 6.307003348497944195 ) ) ;
#10087=CARTESIAN_POINT ( 'NONE',  ( -32.98288769728823411, 203.5309553116391896, -1.857196546604028997 ) ) ;
#10110=CARTESIAN_POINT ( 'NONE',  ( -43.86086230271183695, 213.1499508600178387, -5.686928522499747451 ) ) ;
#10111=CARTESIAN_POINT ( 'NONE',  ( -54.94419563604517265, 203.5000000000000000, 0.1155267958017914542 ) ) ;
#10115=CARTESIAN_POINT ( 'NONE',  ( -50.20163769728823411, 213.9548777149308592, -2.149950860017830756 ) ) ;
#10116=CARTESIAN_POINT ( 'NONE',  ( -57.12872103062157692, 203.4690446883607535, 1.626142955000567936 ) ) ;
#10120=CARTESIAN_POINT ( 'NONE',  ( -42.87127896937849414, 218.5309553116392465, 2.162041339862725842 ) ) ;
#10132=CARTESIAN_POINT ( 'NONE',  ( -40.30580436395489841, 216.5000000000000000, 0.1155267958017343610 ) ) ;
#10158=CARTESIAN_POINT ( 'NONE',  ( -49.20461230271185116, 208.6787018382582346, -4.469044688360757966 ) ) ;
#10162=CARTESIAN_POINT ( 'NONE',  ( -46.44122103062156270, 208.3738570449993404, -6.530955311639226935 ) ) ;
#10163=CARTESIAN_POINT ( 'NONE',  ( -61.08705436395490551, 203.8621396198270475, -6.307003348497942419 ) ) ;
#10169=CARTESIAN_POINT ( 'NONE',  ( -46.63169563604516554, 210.1155267958017703, 6.500000000000000888 ) ) ;
#10176=CARTESIAN_POINT ( 'NONE',  ( -58.51413769728823411, 213.1499508600178672, 5.686928522499718142 ) ) ;
#10180=CARTESIAN_POINT ( 'NONE',  ( -32.58705436395489841, 203.8621396198270475, -6.307003348497942419 ) ) ;
#10207=CARTESIAN_POINT ( 'NONE',  ( -53.17038769728823411, 208.6787018382581778, 4.469044688360752637 ) ) ;
#10252=CARTESIAN_POINT ( 'NONE',  ( -50.19419563604517975, 201.5000000000000000, 0.1155267958018195706 ) ) ;
#10255=CARTESIAN_POINT ( 'NONE',  ( -41.48586230271182984, 207.8500491399821613, 3.954877714930852495 ) ) ;
#10294=CARTESIAN_POINT ( 'NONE',  ( -55.73586230271182984, 206.8500491399821328, 5.686928522499748340 ) ) ;
#10297=CARTESIAN_POINT ( 'NONE',  ( -44.06622103062156270, 211.0902445701382533, 4.530955311639240257 ) ) ;
#10298=CARTESIAN_POINT ( 'NONE',  ( -63.85788769728821279, 216.4690446883607535, 1.857196546604031662 ) ) ;
#10303=CARTESIAN_POINT ( 'NONE',  ( -47.42336230271184405, 217.4189793300686233, 4.149950860017807663 ) ) ;
#10315=CARTESIAN_POINT ( 'NONE',  ( -39.90997103062156270, 215.5714017266979852, 3.350049139982118618 ) ) ;
#10345=CARTESIAN_POINT ( 'NONE',  ( -59.69419563604517265, 205.4999999999999716, 0.1155267958017633378 ) ) ;
#10348=CARTESIAN_POINT ( 'NONE',  ( -44.06622103062156981, 211.6261429550005744, 6.530955311639227823 ) ) ;
#10349=CARTESIAN_POINT ( 'NONE',  ( -59.30580436395490551, 218.5000000000000000, 0.1155267958017064944 ) ) ;
#10355=CARTESIAN_POINT ( 'NONE',  ( -43.86086230271183695, 213.1499508600178387, -5.686928522499747451 ) ) ;
#10364=CARTESIAN_POINT ( 'NONE',  ( -59.50372103062156981, 216.5309553116392181, -1.626142955000564383 ) ) ;
#10368=CARTESIAN_POINT ( 'NONE',  ( -42.48288769728823411, 201.5309553116392181, -2.393094931466246855 ) ) ;
#10391=CARTESIAN_POINT ( 'NONE',  ( -58.11830436395491262, 209.8844732041982297, 4.499999999999996447 ) ) ;
#10441=CARTESIAN_POINT ( 'NONE',  ( -58.90252896937851546, 205.6499508600178103, -7.303452534266820173 ) ) ;
#10444=CARTESIAN_POINT ( 'NONE',  ( -31.19419563604517265, 205.4999999999999716, 0.1155267958017633378 ) ) ;
#10476=CARTESIAN_POINT ( 'NONE',  ( -55.14211230271182274, 203.5309553116391612, 1.857196546604092280 ) ) ;
#10479=CARTESIAN_POINT ( 'NONE',  ( -67.41294563604516554, 213.2096571498974527, -3.378800118222469617 ) ) ;
#10481=CARTESIAN_POINT ( 'NONE',  ( -61.28497103062156981, 204.4285982733020148, -3.350049139982115509 ) ) ;
#10485=CARTESIAN_POINT ( 'NONE',  ( -43.86086230271183695, 214.1499508600178387, -7.418979330068641964 ) ) ;
#10526=CARTESIAN_POINT ( 'NONE',  ( -62.26711230271183695, 216.4690446883607535, -1.857196546604089393 ) ) ;
#10529=CARTESIAN_POINT ( 'NONE',  ( -57.91294563604517265, 213.2096571498974527, -3.378800118222469617 ) ) ;
#10533=CARTESIAN_POINT ( 'NONE',  ( -45.84747103062156981, 213.3500491399821328, -5.571401726697985168 ) ) ;
#10534=CARTESIAN_POINT ( 'NONE',  ( -62.67038769728824121, 207.6069050685337913, 8.469044688360781947 ) ) ;
#10538=CARTESIAN_POINT ( 'NONE',  ( -49.00669563604516554, 209.8844732041982013, -6.500000000000000888 ) ) ;
#10549=CARTESIAN_POINT ( 'NONE',  ( -60.09747103062156981, 213.3500491399821328, -5.571401726697985168 ) ) ;
#10553=CARTESIAN_POINT ( 'NONE',  ( -59.50372103062156981, 216.5309553116391612, -1.626142955000564383 ) ) ;
#10577=CARTESIAN_POINT ( 'NONE',  ( -61.28497103062156981, 206.1606490808709111, -2.350049139982163027 ) ) ;
#10624=CARTESIAN_POINT ( 'NONE',  ( -48.21502896937850124, 217.3034525342667962, -4.350049139982195001 ) ) ;
#10627=CARTESIAN_POINT ( 'NONE',  ( -34.95461230271183695, 208.6787018382582346, -4.469044688360757966 ) ) ;
#10664=CARTESIAN_POINT ( 'NONE',  ( -45.24627896937850835, 203.4690446883607535, -1.626142955000504209 ) ) ;
#10668=CARTESIAN_POINT ( 'NONE',  ( -40.30580436395490551, 214.5000000000000284, 0.1155267958017899832 ) ) ;
#10669=CARTESIAN_POINT ( 'NONE',  ( -53.76413769728823411, 213.1499508600178672, 5.686928522499718142 ) ) ;
#10673=CARTESIAN_POINT ( 'NONE',  ( -36.93377896937849414, 207.8379586601372750, 8.530955311639258909 ) ) ;
#10692=CARTESIAN_POINT ( 'NONE',  ( -62.47247103062156981, 206.6499508600178672, 5.571401726697986057 ) ) ;
#10713=CARTESIAN_POINT ( 'NONE',  ( -58.70461230271182984, 208.1428034533958851, -6.469044688360754414 ) ) ;
#10715=CARTESIAN_POINT ( 'NONE',  ( -52.17336230271184405, 213.9548777149308023, 2.149950860017852960 ) ) ;
#10719=CARTESIAN_POINT ( 'NONE',  ( -32.58705436395489841, 205.3262412349647263, -4.842901733360204020 ) ) ;
#10720=CARTESIAN_POINT ( 'NONE',  ( -56.73288769728824832, 201.5309553116392181, -2.393094931466246855 ) ) ;
#10724=CARTESIAN_POINT ( 'NONE',  ( -30.79836230271183695, 204.3130714775002446, -3.149950860017828091 ) ) ;
#10734=CARTESIAN_POINT ( 'NONE',  ( -43.86830436395490551, 209.8844732041982581, 6.500000000000000888 ) ) ;
#10738=CARTESIAN_POINT ( 'NONE',  ( -60.49330436395489841, 210.1155267958017134, -6.500000000000000888 ) ) ;
#10765=CARTESIAN_POINT ( 'NONE',  ( -56.13913769728823411, 207.8500491399821613, -3.954877714930864485 ) ) ;
#10814=CARTESIAN_POINT ( 'NONE',  ( -39.11086230271183695, 214.1499508600178387, -7.418979330068641964 ) ) ;
#10817=CARTESIAN_POINT ( 'NONE',  ( -30.20461230271183339, 208.6787018382582346, -4.469044688360757966 ) ) ;
#10820=CARTESIAN_POINT ( 'NONE',  ( -41.29538769728821990, 211.8571965466039444, -6.469044688360768625 ) ) ;
#10851=CARTESIAN_POINT ( 'NONE',  ( -48.41294563604515133, 214.6737587650350747, -4.842901733360249317 ) ) ;
#10857=CARTESIAN_POINT ( 'NONE',  ( -34.96205436395489841, 213.2096571498974242, 3.378800118222489601 ) ) ;
#10858=CARTESIAN_POINT ( 'NONE',  ( -49.80580436395490551, 216.5000000000000000, 0.1155267958017343610 ) ) ;
#10862=CARTESIAN_POINT ( 'NONE',  ( -67.42038769728826253, 207.6069050685337913, 8.469044688360781947 ) ) ;
#10881=CARTESIAN_POINT ( 'NONE',  ( -66.82663769728823411, 204.3130714775002730, 3.149950860017883603 ) ) ;
#10899=CARTESIAN_POINT ( 'NONE',  ( -61.67336230271183695, 215.6869285224997270, 3.149950860017831200 ) ) ;
#10901=CARTESIAN_POINT ( 'NONE',  ( -45.84002896937850124, 206.1606490808709111, 2.350049139982143931 ) ) ;
#10906=CARTESIAN_POINT ( 'NONE',  ( -39.31622103062156270, 211.6261429550005744, 6.530955311639227823 ) ) ;
#10907=CARTESIAN_POINT ( 'NONE',  ( -40.50372103062156981, 218.5309553116391896, -2.162041339862839084 ) ) ;
#10911=CARTESIAN_POINT ( 'NONE',  ( -31.39211230271182984, 203.5309553116391612, 1.857196546604092280 ) ) ;
#10920=CARTESIAN_POINT ( 'NONE',  ( -46.24330436395489841, 210.1155267958017134, -6.500000000000000888 ) ) ;
#10924=CARTESIAN_POINT ( 'NONE',  ( -61.68080436395489841, 203.5000000000000000, -0.1155267958017335561 ) ) ;
#10950=CARTESIAN_POINT ( 'NONE',  ( -43.27455436395490551, 206.6211998817774997, 3.209657149897401585 ) ) ;
#10998=CARTESIAN_POINT ( 'NONE',  ( -48.01711230271184405, 218.4690446883607535, -2.393094931466363651 ) ) ;
#11002=CARTESIAN_POINT ( 'NONE',  ( -35.54836230271182984, 206.0451222850691977, -2.149950860017851184 ) ) ;
#11005=CARTESIAN_POINT ( 'NONE',  ( -47.82663769728823411, 204.3130714775002730, 3.149950860017883603 ) ) ;
#11038=CARTESIAN_POINT ( 'NONE',  ( -47.02752896937850124, 213.3500491399821613, 5.571401726697954970 ) ) ;
#11041=CARTESIAN_POINT ( 'NONE',  ( -32.98288769728823411, 205.5309553116392465, -1.321298161741839117 ) ) ;
#11042=CARTESIAN_POINT ( 'NONE',  ( -44.26413769728823411, 213.1499508600178672, 5.686928522499718142 ) ) ;
#11047=CARTESIAN_POINT ( 'NONE',  ( -31.78794563604516910, 203.8621396198271043, 6.307003348498029460 ) ) ;
#11088=CARTESIAN_POINT ( 'NONE',  ( -66.81919563604517975, 216.5000000000000000, -0.1155267958017906493 ) ) ;
#11090=CARTESIAN_POINT ( 'NONE',  ( -36.53794563604517265, 206.7903428501025758, 3.378800118222471838 ) ) ;
#11095=CARTESIAN_POINT ( 'NONE',  ( -34.56622103062155560, 211.6261429550005744, 6.530955311639227823 ) ) ;
#11096=CARTESIAN_POINT ( 'NONE',  ( -50.59747103062156981, 214.3500491399821044, -7.303452534266878793 ) ) ;
#11101=CARTESIAN_POINT ( 'NONE',  ( -35.74627896937850124, 203.4690446883607535, -1.626142955000504209 ) ) ;
#11112=CARTESIAN_POINT ( 'NONE',  ( -61.87872103062154849, 203.4690446883607535, 1.626142955000567936 ) ) ;
#11138=CARTESIAN_POINT ( 'NONE',  ( -48.42038769728824832, 208.6787018382581778, 4.469044688360752637 ) ) ;
#11183=CARTESIAN_POINT ( 'NONE',  ( -38.31919563604515844, 218.5000000000000000, -0.1155267958018185298 ) ) ;
#11185=CARTESIAN_POINT ( 'NONE',  ( -37.72544563604516554, 213.3788001182224718, 3.209657149897419348 ) ) ;
#11188=CARTESIAN_POINT ( 'NONE',  ( -49.21205436395490551, 214.6737587650352168, 4.842901733360204908 ) ) ;
#11224=CARTESIAN_POINT ( 'NONE',  ( -38.71502896937850124, 215.5714017266979567, -3.350049139982168800 ) ) ;
#11227=CARTESIAN_POINT ( 'NONE',  ( -33.37872103062156981, 205.4690446883607535, 1.090244570138264368 ) ) ;
#11228=CARTESIAN_POINT ( 'NONE',  ( -50.39955436395490551, 214.8429017333601792, -4.673758765035196383 ) ) ;
#11234=CARTESIAN_POINT ( 'NONE',  ( -37.72544563604516554, 216.3070033484980854, 6.137860380172893926 ) ) ;
#11254=CARTESIAN_POINT ( 'NONE',  ( -69.99330436395490551, 210.1155267958017134, -6.500000000000000888 ) ) ;
#11276=CARTESIAN_POINT ( 'NONE',  ( -64.24627896937849414, 203.4690446883607535, -1.626142955000504209 ) ) ;
#11278=CARTESIAN_POINT ( 'NONE',  ( -44.45461230271183695, 208.6787018382582346, -4.469044688360757966 ) ) ;
#11281=CARTESIAN_POINT ( 'NONE',  ( -33.37872103062156981, 203.4690446883607535, 1.626142955000567936 ) ) ;
#11282=CARTESIAN_POINT ( 'NONE',  ( -48.81622103062156981, 212.1620413398628671, 8.530955311639223382 ) ) ;
#11288=CARTESIAN_POINT ( 'NONE',  ( -35.54836230271183695, 204.3130714775002446, -3.149950860017828091 ) ) ;
#11299=CARTESIAN_POINT ( 'NONE',  ( -57.32663769728823411, 204.3130714775002730, 3.149950860017883603 ) ) ;
#11323=CARTESIAN_POINT ( 'NONE',  ( -43.47247103062156981, 207.6499508600178387, 3.839350919129076445 ) ) ;
#11376=CARTESIAN_POINT ( 'NONE',  ( -39.31622103062156270, 211.6261429550005744, 6.530955311639227823 ) ) ;
#11412=CARTESIAN_POINT ( 'NONE',  ( -37.32961230271182274, 211.8571965466040297, 6.469044688360755302 ) ) ;
#11413=PRESENTATION_STYLE_ASSIGNMENT (( #20138 ) ) ;
#11415=CARTESIAN_POINT ( 'NONE',  ( -57.31919563604516554, 214.5000000000000284, -0.1155267958017627827 ) ) ;
#11416=CARTESIAN_POINT ( 'NONE',  ( -42.87872103062156981, 203.4690446883607535, 1.626142955000567936 ) ) ;
#11423=CARTESIAN_POINT ( 'NONE',  ( -30.99627896937850480, 201.4690446883607251, -2.162041339862721845 ) ) ;
#11439=CARTESIAN_POINT ( 'NONE',  ( -50.20163769728823411, 215.6869285224996986, -3.149950860017881382 ) ) ;
#11458=CARTESIAN_POINT ( 'NONE',  ( -48.21502896937850124, 215.5714017266979567, -3.350049139982168800 ) ) ;
#11460=CARTESIAN_POINT ( 'NONE',  ( -41.28794563604517265, 206.7903428501025758, 3.378800118222471838 ) ) ;
#11464=CARTESIAN_POINT ( 'NONE',  ( -59.10788769728823411, 214.4690446883608104, 1.321298161741840893 ) ) ;
#11465=CARTESIAN_POINT ( 'NONE',  ( -46.04538769728823411, 212.3930949314662371, -8.469044688360781947 ) ) ;
#11469=CARTESIAN_POINT ( 'NONE',  ( -38.51711230271183695, 216.4690446883607535, -1.857196546604089393 ) ) ;
#11481=CARTESIAN_POINT ( 'NONE',  ( -47.62872103062154849, 203.4690446883607535, 1.626142955000567936 ) ) ;
#11506=CARTESIAN_POINT ( 'NONE',  ( -42.68080436395489841, 205.4999999999999716, -0.1155267958017894420 ) ) ;
#11559=CARTESIAN_POINT ( 'NONE',  ( -34.76413769728823411, 213.1499508600178672, 5.686928522499718142 ) ) ;
#11591=CARTESIAN_POINT ( 'NONE',  ( -61.87127896937851546, 218.5309553116392465, 2.162041339862725842 ) ) ;
#11593=FILL_AREA_STYLE_COLOUR ( '', #25636 ) ;
#11595=CARTESIAN_POINT ( 'NONE',  ( -54.94419563604517265, 205.4999999999999716, 0.1155267958017633378 ) ) ;
#11596=CARTESIAN_POINT ( 'NONE',  ( -50.59747103062156270, 213.3500491399821328, -5.571401726697985168 ) ) ;
#11602=CARTESIAN_POINT ( 'NONE',  ( -55.34747103062157692, 214.3500491399821044, -7.303452534266878793 ) ) ;
#11607=CARTESIAN_POINT ( 'NONE',  ( -38.52455436395489841, 205.1570982666397640, 4.673758765035199048 ) ) ;
#11619=CARTESIAN_POINT ( 'NONE',  ( -60.09747103062156981, 213.3500491399821328, -5.571401726697985168 ) ) ;
#11637=CARTESIAN_POINT ( 'NONE',  ( -51.97544563604517265, 214.8429017333602360, 4.673758765035156415 ) ) ;
#11639=CARTESIAN_POINT ( 'NONE',  ( -48.41294563604517265, 213.2096571498974527, -3.378800118222469617 ) ) ;
#11642=CARTESIAN_POINT ( 'NONE',  ( -58.51413769728822700, 212.1499508600178387, 3.954877714930865817 ) ) ;
#11643=CARTESIAN_POINT ( 'NONE',  ( -39.51413769728823411, 214.1499508600179240, 7.418979330068584233 ) ) ;
#11647=CARTESIAN_POINT ( 'NONE',  ( -60.28794563604517975, 203.8621396198271043, 6.307003348498029460 ) ) ;
#11658=CARTESIAN_POINT ( 'NONE',  ( -52.97247103062156981, 206.6499508600178672, 5.571401726697986057 ) ) ;
#11689=CARTESIAN_POINT ( 'NONE',  ( -49.40997103062157692, 213.8393509191290889, 2.350049139982164359 ) ) ;
#11693=CARTESIAN_POINT ( 'NONE',  ( -56.93080436395490551, 203.5000000000000000, -0.1155267958017335561 ) ) ;
#11746=CARTESIAN_POINT ( 'NONE',  ( -37.13913769728823411, 206.8500491399821044, -5.686928522499717253 ) ) ;
#11781=CARTESIAN_POINT ( 'NONE',  ( -62.26711230271183695, 218.4690446883607535, -2.393094931466363651 ) ) ;
#11784=CARTESIAN_POINT ( 'NONE',  ( -58.90252896937851546, 207.6499508600178387, -3.839350919129087547 ) ) ;
#11785=CARTESIAN_POINT ( 'NONE',  ( -37.73288769728821279, 203.5309553116391612, -1.857196546604028775 ) ) ;
#11790=CARTESIAN_POINT ( 'NONE',  ( -64.25372103062157692, 218.5309553116391896, -2.162041339862839084 ) ) ;
#11796=CARTESIAN_POINT ( 'NONE',  ( -36.54538769728823411, 211.8571965466040012, -6.469044688360769513 ) ) ;
#11808=CARTESIAN_POINT ( 'NONE',  ( -55.14955436395487709, 214.8429017333601792, -4.673758765035196383 ) ) ;
#11824=CARTESIAN_POINT ( 'NONE',  ( -53.16294563604516554, 214.6737587650350747, -4.842901733360248429 ) ) ;
#11826=CARTESIAN_POINT ( 'NONE',  ( -35.15252896937850124, 207.6499508600178387, -3.839350919129087547 ) ) ;
#11829=CARTESIAN_POINT ( 'NONE',  ( -62.27455436395490551, 206.6211998817774997, 3.209657149897401585 ) ) ;
#11830=CARTESIAN_POINT ( 'NONE',  ( -66.62872103062152007, 203.4690446883607535, 1.626142955000567936 ) ) ;
#11834=CARTESIAN_POINT ( 'NONE',  ( -62.86086230271182984, 214.1499508600178387, -7.418979330068641964 ) ) ;
#11847=CARTESIAN_POINT ( 'NONE',  ( -47.23288769728823411, 203.5309553116391612, -1.857196546604028775 ) ) ;
#11873=CARTESIAN_POINT ( 'NONE',  ( -61.27752896937849414, 212.3500491399821613, 3.839350919129088435 ) ) ;
#11877=CARTESIAN_POINT ( 'NONE',  ( -65.04538769728824832, 211.8571965466039444, -6.469044688360768625 ) ) ;
#11879=CARTESIAN_POINT ( 'NONE',  ( -43.26711230271184405, 218.4690446883607535, -2.393094931466363651 ) ) ;
#11884=CARTESIAN_POINT ( 'NONE',  ( -52.96502896937850124, 215.5714017266979567, -3.350049139982168800 ) ) ;
#11892=CARTESIAN_POINT ( 'NONE',  ( -67.42038769728823411, 208.1428034533959703, 6.469044688360771289 ) ) ;
#11929=CARTESIAN_POINT ( 'NONE',  ( -67.02455436395489130, 206.6211998817774997, 3.209657149897401585 ) ) ;
#11966=CARTESIAN_POINT ( 'NONE',  ( -34.55877896937847993, 211.6261429550004607, -6.530955311639245586 ) ) ;
#11970=CARTESIAN_POINT ( 'NONE',  ( -51.77752896937850124, 212.3500491399821613, 3.839350919129088435 ) ) ;
#11975=CARTESIAN_POINT ( 'NONE',  ( -55.94122103062156981, 207.8379586601371329, -8.530955311639223382 ) ) ;
#11983=CARTESIAN_POINT ( 'NONE',  ( -40.30580436395489841, 216.5000000000000000, 0.1155267958017343610 ) ) ;
#11996=CARTESIAN_POINT ( 'NONE',  ( -52.37872103062156270, 203.4690446883607535, 1.626142955000567936 ) ) ;
#12011=CARTESIAN_POINT ( 'NONE',  ( -53.36086230271183695, 213.1499508600178387, -5.686928522499747451 ) ) ;
#12013=CARTESIAN_POINT ( 'NONE',  ( -67.41294563604516554, 214.6737587650350747, -4.842901733360249317 ) ) ;
#12018=CARTESIAN_POINT ( 'NONE',  ( -57.52455436395489841, 206.6211998817774997, 3.209657149897401585 ) ) ;
#12019=CARTESIAN_POINT ( 'NONE',  ( -67.02455436395489130, 205.1570982666397356, 4.673758765035198159 ) ) ;
#12024=CARTESIAN_POINT ( 'NONE',  ( -63.05877896937850835, 212.1620413398627534, -8.530955311639255356 ) ) ;
#12035=CARTESIAN_POINT ( 'NONE',  ( -53.56622103062157692, 211.6261429550005744, 6.530955311639227823 ) ) ;
#12060=CARTESIAN_POINT ( 'NONE',  ( -36.54538769728824121, 211.3212981617418222, -4.469044688360751749 ) ) ;
#12064=CARTESIAN_POINT ( 'NONE',  ( -63.46205436395489841, 214.6737587650352168, 4.842901733360204908 ) ) ;
#12065=CARTESIAN_POINT ( 'NONE',  ( -31.19419563604517265, 201.5000000000000000, 0.1155267958018195706 ) ) ;
#12070=CARTESIAN_POINT ( 'NONE',  ( -52.17336230271183695, 215.6869285224997270, 3.149950860017831200 ) ) ;
#12114=CARTESIAN_POINT ( 'NONE',  ( -33.37872103062156981, 203.4690446883607535, 1.626142955000567936 ) ) ;
#12151=CARTESIAN_POINT ( 'NONE',  ( -65.43377896937850835, 207.8379586601372750, 8.530955311639258909 ) ) ;
#12156=CARTESIAN_POINT ( 'NONE',  ( -64.04836230271183695, 206.0451222850691977, -2.149950860017851184 ) ) ;
#12163=CARTESIAN_POINT ( 'NONE',  ( -60.69122103062156981, 207.8379586601371329, -8.530955311639223382 ) ) ;
#12197=CARTESIAN_POINT ( 'NONE',  ( -44.65252896937850835, 206.6499508600178387, -5.571401726697954970 ) ) ;
#12199=CARTESIAN_POINT ( 'NONE',  ( -34.75669563604515844, 209.8844732041982297, -4.499999999999996447 ) ) ;
#12205=CARTESIAN_POINT ( 'NONE',  ( -59.50372103062157692, 214.5309553116392749, -1.090244570138262148 ) ) ;
#12206=CARTESIAN_POINT ( 'NONE',  ( -31.99330436395490196, 210.1155267958016850, -8.500000000000003553 ) ) ;
#12210=CARTESIAN_POINT ( 'NONE',  ( -56.92336230271183695, 217.4189793300686233, 4.149950860017807663 ) ) ;
#12222=CARTESIAN_POINT ( 'NONE',  ( -54.75372103062154849, 216.5309553116391612, -1.626142955000564383 ) ) ;
#12250=CARTESIAN_POINT ( 'NONE',  ( -34.96205436395489841, 213.2096571498974242, 3.378800118222489601 ) ) ;
#12254=CARTESIAN_POINT ( 'NONE',  ( -63.65997103062156981, 215.5714017266979852, 3.350049139982118618 ) ) ;
#12256=CARTESIAN_POINT ( 'NONE',  ( -65.24330436395489130, 210.1155267958016850, -8.500000000000003553 ) ) ;
#12261=CARTESIAN_POINT ( 'NONE',  ( -56.72544563604517265, 214.8429017333602360, 4.673758765035156415 ) ) ;
#12269=CARTESIAN_POINT ( 'NONE',  ( -64.25372103062156270, 216.5309553116392181, -1.626142955000564383 ) ) ;
#12307=CARTESIAN_POINT ( 'NONE',  ( -33.77455436395490551, 205.1570982666397356, 4.673758765035198159 ) ) ;
#12330=ORIENTED_EDGE ( 'NONE', *, *, #24996, .T. ) ;
#12344=CARTESIAN_POINT ( 'NONE',  ( -62.86086230271182984, 214.1499508600178387, -7.418979330068641964 ) ) ;
#12348=CARTESIAN_POINT ( 'NONE',  ( -39.90252896937850124, 207.6499508600178387, -3.839350919129087547 ) ) ;
#12356=CARTESIAN_POINT ( 'NONE',  ( -64.84747103062156270, 214.3500491399821044, -7.303452534266878793 ) ) ;
#12391=CARTESIAN_POINT ( 'NONE',  ( -38.71502896937850124, 215.5714017266979567, -3.350049139982168800 ) ) ;
#12392=CARTESIAN_POINT ( 'NONE',  ( -63.05877896937850835, 211.6261429550004607, -6.530955311639245586 ) ) ;
#12395=CARTESIAN_POINT ( 'NONE',  ( -52.97247103062156270, 207.6499508600178387, 3.839350919129076445 ) ) ;
#12396=CARTESIAN_POINT ( 'NONE',  ( -35.15997103062156270, 217.3034525342668815, 4.350049139982096413 ) ) ;
#12400=CARTESIAN_POINT ( 'NONE',  ( -62.46502896937850124, 217.3034525342667962, -4.350049139982195001 ) ) ;
#12413=CARTESIAN_POINT ( 'NONE',  ( -40.70163769728823411, 215.6869285224996986, -3.149950860017881382 ) ) ;
#12442=CARTESIAN_POINT ( 'NONE',  ( -65.23586230271183695, 207.8500491399821613, 3.954877714930852495 ) ) ;
#12447=CARTESIAN_POINT ( 'NONE',  ( -53.96205436395489130, 214.6737587650352168, 4.842901733360204908 ) ) ;
#12448=CARTESIAN_POINT ( 'NONE',  ( -69.39955436395489130, 216.3070033484980002, -6.137860380172975638 ) ) ;
#12452=CARTESIAN_POINT ( 'NONE',  ( -63.25669563604516554, 209.8844732041982013, -6.500000000000000888 ) ) ;
#12460=CARTESIAN_POINT ( 'NONE',  ( -62.07663769728823411, 204.3130714775002730, 3.149950860017883603 ) ) ;
#12464=CARTESIAN_POINT ( 'NONE',  ( -69.20163769728823411, 215.6869285224996986, -3.149950860017881382 ) ) ;
#12485=( BOUNDED_CURVE ( )  B_SPLINE_CURVE ( 2, ( #35380, #327, #3734, #1078, #20444, #35574, #34824, #15307, #8867, #29131, #21195, #29513, #6397, #11892, #6015, #3554, #15116, #32170, #6770, #26859, #23460, #15496, #29893, #9057, #26667, #26478, #6208, #14931, #697, #12269, #23840, #29700, #9430, #17780, #21008, #29323, #32542, #888, #3923, #6584, #12460, #27052, #21381, #24400, #27613, #18542, #24583, #36135, #30272, #32921, #10549, #27420, #9987, #10364, #18916, #15877, #33113, #33484, #10176, #7712, #21938, #7157, #19294, #21751, #33303, #7528, #24213, #1453, #6973, #21568, #19102, #16435, #7342, #30467, #18731, #30653, #4115, #2013, #30833, #4488, #30080, #16251, #4668, #16065, #4857, #27982, #4298, #12833, #1644, #36504, #27801, #13216, #24765, #13027, #1828, #35758, #36316, #13397, #9803, #24947, #22124, #33672, #15687, #27239, #1262, #35948, #17685, #29418, #17873, #14645, #13777, #36874, #2885, #28166, #29222, #13588, #26382, #35099, #8773, #2197, #10920, #14458, #22495, #25140, #3265, #23365, #19474, #34729, #26195, #31020, #20531, #36694, #10734, #14837, #22307, #32073, #33859, #7901, #417, #20345, #26013, #5042, #34915, #16624, #9148, #3076, #25325, #34042, #8087, #32258, #11983, #19661, #42, #5729, #31702, #6102, #17310, #28851, #23555, #11607, #20715, #23182, #6302, #31887, #5917, #17496, #29032, #8960, #233, #11796, #29988, #3643, #3450, #600, #21657, #15784, #18824, #29796, #32639, #23743, #21101, #32826, #35281, #4019, #15213, #6870, #24311, #10087, #7250, #793, #12934, #6680, #3828 ),
 .UNSPECIFIED., .F., .F. ) 
 B_SPLINE_CURVE_WITH_KNOTS ( ( 3, 2, 2, 2, 2, 2, 2, 2, 2, 2, 2, 2, 2, 2, 2, 2, 2, 2, 2, 2, 2, 2, 2, 2, 2, 2, 2, 2, 2, 2, 2, 2, 2, 2, 2, 2, 2, 2, 2, 2, 2, 2, 2, 2, 2, 2, 2, 2, 2, 2, 2, 2, 2, 2, 2, 2, 2, 2, 2, 2, 2, 2, 2, 2, 2, 2, 2, 2, 2, 2, 2, 2, 2, 2, 2, 2, 2, 2, 2, 2, 2, 2, 2, 2, 2, 2, 2, 2, 2, 2, 2, 2, 2, 2, 2, 2, 3 ),
 ( 0.000000000000000000, 0.01041666666666666609, 0.02083333333333333218, 0.03125000000000000000, 0.04166666666666666435, 0.05208333333333333565, 0.06250000000000000000, 0.07291666666666667129, 0.08333333333333332871, 0.09375000000000000000, 0.1041666666666666713, 0.1145833333333333287, 0.1250000000000000000, 0.1354166666666666574, 0.1458333333333333426, 0.1562500000000000000, 0.1666666666666666574, 0.1770833333333333426, 0.1875000000000000000, 0.1979166666666666574, 0.2083333333333333426, 0.2187500000000000000, 0.2291666666666666574, 0.2395833333333333426, 0.2500000000000000000, 0.2604166666666666852, 0.2708333333333333148, 0.2812500000000000000, 0.2916666666666666852, 0.3020833333333333148, 0.3125000000000000000, 0.3229166666666666852, 0.3333333333333333148, 0.3437500000000000000, 0.3541666666666666852, 0.3645833333333333148, 0.3750000000000000000, 0.3854166666666666852, 0.3958333333333333148, 0.4062500000000000000, 0.4166666666666666852, 0.4270833333333333148, 0.4375000000000000000, 0.4479166666666666852, 0.4583333333333333148, 0.4687500000000000000, 0.4791666666666666852, 0.4895833333333333148, 0.5000000000000000000, 0.5104166666666666297, 0.5208333333333333703, 0.5312500000000000000, 0.5416666666666666297, 0.5520833333333333703, 0.5625000000000000000, 0.5729166666666666297, 0.5833333333333333703, 0.5937500000000000000, 0.6041666666666666297, 0.6145833333333333703, 0.6250000000000000000, 0.6354166666666666297, 0.6458333333333333703, 0.6562500000000000000, 0.6666666666666666297, 0.6770833333333333703, 0.6875000000000000000, 0.6979166666666666297, 0.7083333333333333703, 0.7187500000000000000, 0.7291666666666666297, 0.7395833333333333703, 0.7500000000000000000, 0.7604166666666666297, 0.7708333333333333703, 0.7812500000000000000, 0.7916666666666666297, 0.8020833333333333703, 0.8125000000000000000, 0.8229166666666666297, 0.8333333333333333703, 0.8437500000000000000, 0.8541666666666666297, 0.8645833333333333703, 0.8750000000000000000, 0.8854166666666666297, 0.8958333333333333703, 0.9062500000000000000, 0.9166666666666666297, 0.9270833333333333703, 0.9375000000000000000, 0.9479166666666666297, 0.9583333333333333703, 0.9687500000000000000, 0.9791666666666666297, 0.9895833333333333703, 1.000000000000000000 ),
 .UNSPECIFIED. ) 
 CURVE ( )  GEOMETRIC_REPRESENTATION_ITEM ( )  RATIONAL_B_SPLINE_CURVE ( ( 1.000000000000000000, 0.9659258262890683122, 1.000000000000000000, 0.9659258262890683122, 1.000000000000000000, 0.9659258262890683122, 1.000000000000000000, 0.9659258262890683122, 1.000000000000000000, 0.9659258262890683122, 1.000000000000000000, 0.9659258262890683122, 1.000000000000000000, 0.9659258262890683122, 1.000000000000000000, 0.9659258262890683122, 1.000000000000000000, 0.9659258262890683122, 1.000000000000000000, 0.9659258262890683122, 1.000000000000000000, 0.9659258262890683122, 1.000000000000000000, 0.9659258262890683122, 1.000000000000000000, 0.9659258262890683122, 1.000000000000000000, 0.9659258262890683122, 1.000000000000000000, 0.9659258262890683122, 1.000000000000000000, 0.9659258262890683122, 1.000000000000000000, 0.9659258262890683122, 1.000000000000000000, 0.9659258262890683122, 1.000000000000000000, 0.9659258262890683122, 1.000000000000000000, 0.9659258262890683122, 1.000000000000000000, 0.9659258262890683122, 1.000000000000000000, 0.9659258262890683122, 1.000000000000000000, 0.9659258262890683122, 1.000000000000000000, 0.9659258262890683122, 1.000000000000000000, 0.9659258262890683122, 1.000000000000000000, 0.9659258262890683122, 1.000000000000000000, 0.9659258262890683122, 1.000000000000000000, 0.9659258262890683122, 1.000000000000000000, 0.9659258262890683122, 1.000000000000000000, 0.9659258262890683122, 1.000000000000000000, 0.9659258262890683122, 1.000000000000000000, 0.9659258262890683122, 1.000000000000000000, 0.9659258262890683122, 1.000000000000000000, 0.9659258262890683122, 1.000000000000000000, 0.9659258262890683122, 1.000000000000000000, 0.9659258262890683122, 1.000000000000000000, 0.9659258262890683122, 1.000000000000000000, 0.9659258262890683122, 1.000000000000000000, 0.9659258262890683122, 1.000000000000000000, 0.9659258262890683122, 1.000000000000000000, 0.9659258262890683122, 1.000000000000000000, 0.9659258262890683122, 1.000000000000000000, 0.9659258262890683122, 1.000000000000000000, 0.9659258262890683122, 1.000000000000000000, 0.9659258262890683122, 1.000000000000000000, 0.9659258262890683122, 1.000000000000000000, 0.9659258262890683122, 1.000000000000000000, 0.9659258262890683122, 1.000000000000000000, 0.9659258262890683122, 1.000000000000000000, 0.9659258262890683122, 1.000000000000000000, 0.9659258262890683122, 1.000000000000000000, 0.9659258262890683122, 1.000000000000000000, 0.9659258262890683122, 1.000000000000000000, 0.9659258262890683122, 1.000000000000000000, 0.9659258262890683122, 1.000000000000000000, 0.9659258262890683122, 1.000000000000000000, 0.9659258262890683122, 1.000000000000000000, 0.9659258262890683122, 1.000000000000000000, 0.9659258262890683122, 1.000000000000000000, 0.9659258262890683122, 1.000000000000000000, 0.9659258262890683122, 1.000000000000000000, 0.9659258262890683122, 1.000000000000000000, 0.9659258262890683122, 1.000000000000000000, 0.9659258262890683122, 1.000000000000000000, 0.9659258262890683122, 1.000000000000000000, 0.9659258262890683122, 1.000000000000000000, 0.9659258262890683122, 1.000000000000000000, 0.9659258262890683122, 1.000000000000000000, 0.9659258262890683122, 1.000000000000000000, 0.9659258262890683122, 1.000000000000000000, 0.9659258262890683122, 1.000000000000000000, 0.9659258262890683122, 1.000000000000000000, 0.9659258262890683122, 1.000000000000000000, 0.9659258262890683122, 1.000000000000000000, 0.9659258262890683122, 1.000000000000000000, 0.9659258262890683122, 1.000000000000000000, 0.9659258262890683122, 1.000000000000000000, 0.9659258262890683122, 1.000000000000000000, 0.9659258262890683122, 1.000000000000000000, 0.9659258262890683122, 1.000000000000000000, 0.9659258262890683122, 1.000000000000000000, 0.9659258262890683122, 1.000000000000000000, 0.9659258262890683122, 1.000000000000000000, 0.9659258262890683122, 1.000000000000000000, 0.9659258262890683122, 1.000000000000000000, 0.9659258262890683122, 1.000000000000000000, 0.9659258262890683122, 1.000000000000000000, 0.9659258262890683122, 1.000000000000000000, 0.9659258262890683122, 1.000000000000000000, 0.9659258262890683122, 1.000000000000000000, 0.9659258262890683122, 1.000000000000000000, 0.9659258262890683122, 1.000000000000000000, 0.9659258262890683122, 1.000000000000000000, 0.9659258262890683122, 1.000000000000000000, 0.9659258262890683122, 1.000000000000000000, 0.9659258262890683122, 1.000000000000000000 ) ) 
 REPRESENTATION_ITEM ( '' )  );
#12521=DIRECTION ( 'NONE',  ( 0.9933043639548628789, -0.1155267958017759528, 0.000000000000000000 ) ) ;
#12541=CARTESIAN_POINT ( 'NONE',  ( -52.17336230271184405, 217.4189793300686233, 4.149950860017807663 ) ) ;
#12545=CARTESIAN_POINT ( 'NONE',  ( -45.44419563604516554, 205.4999999999999716, 0.1155267958017633378 ) ) ;
#12546=CARTESIAN_POINT ( 'NONE',  ( -32.98288769728824121, 203.5309553116391612, -1.857196546604028775 ) ) ;
#12551=CARTESIAN_POINT ( 'NONE',  ( -45.64955436395490551, 216.3070033484980002, -6.137860380172975638 ) ) ;
#12580=CARTESIAN_POINT ( 'NONE',  ( -43.46502896937849414, 215.5714017266979567, -3.350049139982168800 ) ) ;
#12581=CARTESIAN_POINT ( 'NONE',  ( -61.47544563604515133, 214.8429017333602360, 4.673758765035156415 ) ) ;
#12585=CARTESIAN_POINT ( 'NONE',  ( -45.64955436395490551, 213.3788001182225003, -3.209657149897400252 ) ) ;
#12586=CARTESIAN_POINT ( 'NONE',  ( -69.39955436395486288, 214.8429017333601792, -4.673758765035196383 ) ) ;
#12590=CARTESIAN_POINT ( 'NONE',  ( -48.41294563604517265, 216.1378603801729241, -6.307003348498026796 ) ) ;
#12603=CARTESIAN_POINT ( 'NONE',  ( -41.29538769728821990, 211.8571965466039444, -6.469044688360768625 ) ) ;
#12630=CARTESIAN_POINT ( 'NONE',  ( -62.26711230271183695, 214.4690446883608104, -1.321298161741814914 ) ) ;
#12634=CARTESIAN_POINT ( 'NONE',  ( -51.38913769728823411, 206.8500491399821044, -5.686928522499717253 ) ) ;
#12635=CARTESIAN_POINT ( 'NONE',  ( -30.79836230271183339, 202.5810206699313767, -4.149950860017804111 ) ) ;
#12640=CARTESIAN_POINT ( 'NONE',  ( -47.62127896937847993, 216.5309553116391612, 1.626142955000506873 ) ) ;
#12652=CARTESIAN_POINT ( 'NONE',  ( -36.14955436395489841, 216.3070033484980002, -6.137860380172975638 ) ) ;
#12727=CARTESIAN_POINT ( 'NONE',  ( -51.18377896937850835, 207.8379586601372750, 8.530955311639258909 ) ) ;
#12731=CARTESIAN_POINT ( 'NONE',  ( -46.82961230271182984, 211.3212981617417938, 4.469044688360757966 ) ) ;
#12737=CARTESIAN_POINT ( 'NONE',  ( -50.79538769728824121, 212.3930949314662371, -8.469044688360781947 ) ) ;
#12767=CARTESIAN_POINT ( 'NONE',  ( -42.07961230271182984, 211.8571965466040581, 6.469044688360755302 ) ) ;
#12768=CARTESIAN_POINT ( 'NONE',  ( -58.11086230271183695, 213.1499508600178387, -5.686928522499747451 ) ) ;
#12771=CARTESIAN_POINT ( 'NONE',  ( -42.48288769728823411, 205.5309553116392465, -1.321298161741839117 ) ) ;
#12772=CARTESIAN_POINT ( 'NONE',  ( -51.58705436395488420, 205.3262412349647263, -4.842901733360204020 ) ) ;
#12776=CARTESIAN_POINT ( 'NONE',  ( -48.21502896937850124, 217.3034525342667962, -4.350049139982195001 ) ) ;
#12814=CARTESIAN_POINT ( 'NONE',  ( -50.39211230271182984, 205.5309553116392465, 1.321298161741817356 ) ) ;
#12818=CARTESIAN_POINT ( 'NONE',  ( -44.46205436395488420, 214.6737587650352168, 4.842901733360204908 ) ) ;
#12819=CARTESIAN_POINT ( 'NONE',  ( -68.40997103062156270, 217.3034525342668815, 4.350049139982096413 ) ) ;
#12824=CARTESIAN_POINT ( 'NONE',  ( -46.03794563604517265, 205.3262412349647832, 4.842901733360250205 ) ) ;
#12833=CARTESIAN_POINT ( 'NONE',  ( -52.77455436395490551, 205.1570982666397640, 4.673758765035199048 ) ) ;
#12837=CARTESIAN_POINT ( 'NONE',  ( -42.68080436395489841, 201.5000000000000000, -0.1155267958017054536 ) ) ;
#12916=CARTESIAN_POINT ( 'NONE',  ( -56.72544563604517265, 216.3070033484980854, 6.137860380172893926 ) ) ;
#12920=CARTESIAN_POINT ( 'NONE',  ( -44.05877896937850124, 211.0902445701383101, -4.530955311639234040 ) ) ;
#12926=CARTESIAN_POINT ( 'NONE',  ( -50.99330436395489841, 210.1155267958016850, -8.500000000000003553 ) ) ;
#12934=CARTESIAN_POINT ( 'NONE',  ( -32.38913769728823411, 206.8500491399821044, -5.686928522499717253 ) ) ;
#12957=CARTESIAN_POINT ( 'NONE',  ( -37.52752896937850124, 213.3500491399821613, 5.571401726697954970 ) ) ;
#12958=CARTESIAN_POINT ( 'NONE',  ( -61.07961230271182274, 211.8571965466040297, 6.469044688360755302 ) ) ;
#12963=CARTESIAN_POINT ( 'NONE',  ( -40.89955436395489841, 213.3788001182225003, -3.209657149897400252 ) ) ;
#12965=CARTESIAN_POINT ( 'NONE',  ( -61.68080436395489841, 203.5000000000000000, -0.1155267958017335561 ) ) ;
#12970=CARTESIAN_POINT ( 'NONE',  ( -43.66294563604516554, 216.1378603801729241, -6.307003348498026796 ) ) ;
#12982=CARTESIAN_POINT ( 'NONE',  ( -42.87872103062156981, 203.4690446883607535, 1.626142955000567936 ) ) ;
#13010=CARTESIAN_POINT ( 'NONE',  ( -56.32961230271183695, 211.3212981617417938, 4.469044688360757966 ) ) ;
#13014=CARTESIAN_POINT ( 'NONE',  ( -51.58705436395488420, 205.3262412349647263, -4.842901733360204020 ) ) ;
#13015=CARTESIAN_POINT ( 'NONE',  ( -52.77455436395490551, 203.6929966515020283, 6.137860380172978303 ) ) ;
#13020=CARTESIAN_POINT ( 'NONE',  ( -50.98586230271183695, 206.8500491399821328, 5.686928522499748340 ) ) ;
#13027=CARTESIAN_POINT ( 'NONE',  ( -51.58705436395489130, 205.3262412349647548, -4.842901733360204908 ) ) ;
#13031=CARTESIAN_POINT ( 'NONE',  ( -42.28497103062156270, 202.6965474657331185, -4.350049139982091084 ) ) ;
#13042=CARTESIAN_POINT ( 'NONE',  ( -67.81622103062156270, 211.6261429550005744, 6.530955311639227823 ) ) ;
#13057=CARTESIAN_POINT ( 'NONE',  ( -58.51413769728822700, 212.1499508600178387, 3.954877714930865817 ) ) ;
#13103=CARTESIAN_POINT ( 'NONE',  ( -51.97544563604517265, 216.3070033484980854, 6.137860380172893926 ) ) ;
#13106=CARTESIAN_POINT ( 'NONE',  ( -47.02752896937850835, 212.3500491399821613, 3.839350919129088435 ) ) ;
#13112=CARTESIAN_POINT ( 'NONE',  ( -51.98288769728823411, 201.5309553116392181, -2.393094931466246855 ) ) ;
#13144=CARTESIAN_POINT ( 'NONE',  ( -55.93377896937850124, 208.3738570449995109, 6.530955311639247363 ) ) ;
#13148=CARTESIAN_POINT ( 'NONE',  ( -49.01413769728823411, 212.1499508600178387, 3.954877714930865817 ) ) ;
#13150=CARTESIAN_POINT ( 'NONE',  ( -56.93080436395490551, 203.5000000000000000, -0.1155267958017335561 ) ) ;
#13153=CARTESIAN_POINT ( 'NONE',  ( -40.89211230271183695, 201.5309553116392181, 2.393094931466368980 ) ) ;
#13164=CARTESIAN_POINT ( 'NONE',  ( -43.27455436395490551, 205.1570982666397356, 4.673758765035198159 ) ) ;
#13195=CARTESIAN_POINT ( 'NONE',  ( -52.56919563604517265, 214.5000000000000284, -0.1155267958017627827 ) ) ;
#13200=CARTESIAN_POINT ( 'NONE',  ( -53.17038769728823411, 208.1428034533959703, 6.469044688360770401 ) ) ;
#13201=CARTESIAN_POINT ( 'NONE',  ( -51.38913769728824121, 205.8500491399820760, -7.418979330068584233 ) ) ;
#13207=CARTESIAN_POINT ( 'NONE',  ( -44.85044563604515133, 205.1570982666397072, -4.673758765035155527 ) ) ;
#13216=CARTESIAN_POINT ( 'NONE',  ( -51.98288769728822700, 203.5309553116391896, -1.857196546604028997 ) ) ;
#13220=CARTESIAN_POINT ( 'NONE',  ( -33.97247103062156270, 205.6499508600178956, 7.303452534266880569 ) ) ;
#13246=CARTESIAN_POINT ( 'NONE',  ( -60.09747103062157692, 212.3500491399821613, -3.839350919129076445 ) ) ;
#13288=CARTESIAN_POINT ( 'NONE',  ( -49.00669563604517265, 209.8844732041981729, -8.500000000000003553 ) ) ;
#13292=CARTESIAN_POINT ( 'NONE',  ( -33.17336230271183695, 213.9548777149308023, 2.149950860017852960 ) ) ;
#13326=CARTESIAN_POINT ( 'NONE',  ( -30.20461230271182984, 208.1428034533958851, -6.469044688360754414 ) ) ;
#13328=CARTESIAN_POINT ( 'NONE',  ( -52.17336230271183695, 215.6869285224997270, 3.149950860017831200 ) ) ;
#13332=CARTESIAN_POINT ( 'NONE',  ( -34.36830436395490551, 209.8844732041982297, 4.499999999999996447 ) ) ;
#13333=CARTESIAN_POINT ( 'NONE',  ( -55.94122103062156270, 208.3738570449993404, -6.530955311639226935 ) ) ;
#13337=CARTESIAN_POINT ( 'NONE',  ( -50.19419563604517975, 201.5000000000000000, 0.1155267958018195706 ) ) ;
#13378=CARTESIAN_POINT ( 'NONE',  ( -58.50669563604516554, 209.8844732041982297, -4.499999999999996447 ) ) ;
#13382=CARTESIAN_POINT ( 'NONE',  ( -45.25372103062155560, 216.5309553116391612, -1.626142955000564383 ) ) ;
#13383=CARTESIAN_POINT ( 'NONE',  ( -63.06622103062156270, 212.1620413398628671, 8.530955311639223382 ) ) ;
#13388=CARTESIAN_POINT ( 'NONE',  ( -43.26711230271183695, 216.4690446883607535, -1.857196546604089393 ) ) ;
#13397=CARTESIAN_POINT ( 'NONE',  ( -50.79538769728823411, 211.8571965466040012, -6.469044688360769513 ) ) ;
#13402=CARTESIAN_POINT ( 'NONE',  ( -66.43080436395490551, 203.5000000000000000, -0.1155267958017335561 ) ) ;
#13426=CARTESIAN_POINT ( 'NONE',  ( -60.49330436395489130, 210.1155267958017703, -4.499999999999996447 ) ) ;
#13474=CARTESIAN_POINT ( 'NONE',  ( -37.92336230271182984, 217.4189793300686233, 4.149950860017807663 ) ) ;
#13477=CARTESIAN_POINT ( 'NONE',  ( -65.23586230271183695, 206.8500491399821328, 5.686928522499748340 ) ) ;
#13513=CARTESIAN_POINT ( 'NONE',  ( -54.74627896937848703, 203.4690446883607535, -1.626142955000504209 ) ) ;
#13517=CARTESIAN_POINT ( 'NONE',  ( -66.81919563604516554, 214.5000000000000284, -0.1155267958017627827 ) ) ;
#13518=CARTESIAN_POINT ( 'NONE',  ( -62.67038769728823411, 208.1428034533959703, 6.469044688360770401 ) ) ;
#13522=CARTESIAN_POINT ( 'NONE',  ( -34.95461230271183695, 207.6069050685336492, -8.469044688360751749 ) ) ;
#13565=CARTESIAN_POINT ( 'NONE',  ( -60.88169563604516554, 210.1155267958017703, 6.500000000000000888 ) ) ;
#13567=CARTESIAN_POINT ( 'NONE',  ( -59.89211230271182274, 205.5309553116392465, 1.321298161741817356 ) ) ;
#13572=CARTESIAN_POINT ( 'NONE',  ( -38.32663769728824121, 204.3130714775002730, 3.149950860017883603 ) ) ;
#13573=CARTESIAN_POINT ( 'NONE',  ( -57.92038769728823411, 207.6069050685337913, 8.469044688360781947 ) ) ;
#13577=CARTESIAN_POINT ( 'NONE',  ( -67.80877896937849414, 212.1620413398627534, -8.530955311639255356 ) ) ;
#13588=CARTESIAN_POINT ( 'NONE',  ( -47.23288769728823411, 203.5309553116391896, -1.857196546604028997 ) ) ;
#13594=CARTESIAN_POINT ( 'NONE',  ( -64.64955436395490551, 214.8429017333601792, -4.673758765035196383 ) ) ;
#13621=CARTESIAN_POINT ( 'NONE',  ( -54.75372103062156270, 214.5309553116392749, -1.090244570138262148 ) ) ;
#13670=CARTESIAN_POINT ( 'NONE',  ( -39.70461230271183695, 207.6069050685336492, -8.469044688360751749 ) ) ;
#13675=CARTESIAN_POINT ( 'NONE',  ( -31.98586230271182984, 207.8500491399821613, 3.954877714930852495 ) ) ;
#13679=CARTESIAN_POINT ( 'NONE',  ( -37.53497103062156981, 204.4285982733020148, -3.350049139982115509 ) ) ;
#13708=CARTESIAN_POINT ( 'NONE',  ( -42.07961230271182984, 211.8571965466040297, 6.469044688360755302 ) ) ;
#13714=CARTESIAN_POINT ( 'NONE',  ( -64.44419563604517975, 205.4999999999999716, 0.1155267958017633378 ) ) ;
#13715=CARTESIAN_POINT ( 'NONE',  ( -42.28497103062156270, 204.4285982733020148, -3.350049139982115509 ) ) ;
#13716=ADVANCED_FACE ( 'NONE', ( #5001 ), #14813, .T. ) ;
#13720=CARTESIAN_POINT ( 'NONE',  ( -34.75669563604515844, 209.8844732041981729, -8.500000000000003553 ) ) ;
#13733=CARTESIAN_POINT ( 'NONE',  ( -69.00000000000002842, 209.9999999999999716, -6.500000000000000888 ) ) ;
#13739=CARTESIAN_POINT ( 'NONE',  ( -69.39955436395486288, 214.8429017333601792, -4.673758765035196383 ) ) ;
#13759=CARTESIAN_POINT ( 'NONE',  ( -47.02752896937850835, 212.3500491399821613, 3.839350919129088435 ) ) ;
#13763=CARTESIAN_POINT ( 'NONE',  ( -35.75372103062156981, 216.5309553116391612, -1.626142955000564383 ) ) ;
#13764=CARTESIAN_POINT ( 'NONE',  ( -54.55580436395489841, 218.5000000000000000, 0.1155267958017064944 ) ) ;
#13768=CARTESIAN_POINT ( 'NONE',  ( -39.11086230271183695, 213.1499508600178387, -5.686928522499747451 ) ) ;
#13777=CARTESIAN_POINT ( 'NONE',  ( -48.22247103062156270, 206.6499508600178672, 5.571401726697986057 ) ) ;
#13781=CARTESIAN_POINT ( 'NONE',  ( -64.45163769728823411, 215.6869285224996986, -3.149950860017881382 ) ) ;
#13808=CARTESIAN_POINT ( 'NONE',  ( -52.57663769728824832, 206.0451222850691408, 2.149950860017832532 ) ) ;
#13854=CARTESIAN_POINT ( 'NONE',  ( -36.73586230271183695, 205.8500491399821613, 7.418979330068642852 ) ) ;
#13857=CARTESIAN_POINT ( 'NONE',  ( -33.56919563604517265, 214.5000000000000284, -0.1155267958017627827 ) ) ;
#13860=CARTESIAN_POINT ( 'NONE',  ( -40.89955436395488420, 214.8429017333601792, -4.673758765035196383 ) ) ;
#13893=CARTESIAN_POINT ( 'NONE',  ( -42.87127896937850124, 216.5309553116391612, 1.626142955000506873 ) ) ;
#13897=CARTESIAN_POINT ( 'NONE',  ( -36.74330436395489130, 210.1155267958017703, -4.499999999999996447 ) ) ;
#13898=CARTESIAN_POINT ( 'NONE',  ( -42.48288769728824121, 203.5309553116391612, -1.857196546604028775 ) ) ;
#13903=CARTESIAN_POINT ( 'NONE',  ( -38.91294563604516554, 216.1378603801729241, -6.307003348498026796 ) ) ;
#13922=CARTESIAN_POINT ( 'NONE',  ( -69.79538769728823411, 211.8571965466039444, -6.469044688360768625 ) ) ;
#13939=CARTESIAN_POINT ( 'NONE',  ( -63.65252896937849414, 206.6499508600178387, -5.571401726697954970 ) ) ;
#13941=CARTESIAN_POINT ( 'NONE',  ( -37.92336230271182984, 213.9548777149308023, 2.149950860017852960 ) ) ;
#13946=CARTESIAN_POINT ( 'NONE',  ( -37.53497103062156981, 204.4285982733020148, -3.350049139982115509 ) ) ;
#13947=CARTESIAN_POINT ( 'NONE',  ( -49.60788769728823411, 218.4690446883607535, 2.393094931466250408 ) ) ;
#13952=CARTESIAN_POINT ( 'NONE',  ( -37.72544563604515844, 214.8429017333602360, 4.673758765035156415 ) ) ;
#13963=CARTESIAN_POINT ( 'NONE',  ( -63.85788769728821279, 216.4690446883607535, 1.857196546604031662 ) ) ;
#13987=CARTESIAN_POINT ( 'NONE',  ( -47.62872103062157692, 205.4690446883607535, 1.090244570138264368 ) ) ;
#14035=CARTESIAN_POINT ( 'NONE',  ( -38.91294563604516554, 216.1378603801729241, -6.307003348498026796 ) ) ;
#14039=CARTESIAN_POINT ( 'NONE',  ( -67.41294563604516554, 214.6737587650350747, -4.842901733360249317 ) ) ;
#14042=CARTESIAN_POINT ( 'NONE',  ( -49.60788769728823411, 216.4690446883607535, 1.857196546604031662 ) ) ;
#14074=CARTESIAN_POINT ( 'NONE',  ( -39.11086230271183695, 213.1499508600178387, -5.686928522499747451 ) ) ;
#14078=CARTESIAN_POINT ( 'NONE',  ( -32.19122103062156270, 208.9097554298617752, -4.530955311639240257 ) ) ;
#14079=CARTESIAN_POINT ( 'NONE',  ( -48.42038769728821990, 208.1428034533959703, 6.469044688360770401 ) ) ;
#14085=CARTESIAN_POINT ( 'NONE',  ( -31.98586230271182984, 205.8500491399821613, 7.418979330068642852 ) ) ;
#14102=CARTESIAN_POINT ( 'NONE',  ( -64.64955436395490551, 214.8429017333601792, -4.673758765035196383 ) ) ;
#14121=CARTESIAN_POINT ( 'NONE',  ( -60.28794563604516554, 205.3262412349648116, 4.842901733360249317 ) ) ;
#14123=CARTESIAN_POINT ( 'NONE',  ( -39.70461230271183695, 208.6787018382582346, -4.469044688360757966 ) ) ;
#14127=CARTESIAN_POINT ( 'NONE',  ( -40.30580436395489841, 216.5000000000000000, 0.1155267958017343610 ) ) ;
#14128=CARTESIAN_POINT ( 'NONE',  ( -44.46205436395490551, 216.1378603801730094, 6.307003348497944195 ) ) ;
#14133=CARTESIAN_POINT ( 'NONE',  ( -34.55877896937847993, 211.6261429550004607, -6.530955311639245586 ) ) ;
#14146=CARTESIAN_POINT ( 'NONE',  ( -57.72247103062156270, 206.6499508600178672, 5.571401726697986057 ) ) ;
#14170=CARTESIAN_POINT ( 'NONE',  ( -46.63913769728824121, 207.8500491399821613, -3.954877714930864485 ) ) ;
#14178=CARTESIAN_POINT ( 'NONE',  ( -45.64955436395490551, 214.8429017333601792, -4.673758765035196383 ) ) ;
#14221=CARTESIAN_POINT ( 'NONE',  ( -53.95461230271181563, 208.1428034533959135, -6.469044688360754414 ) ) ;
#14225=CARTESIAN_POINT ( 'NONE',  ( -42.87872103062156981, 203.4690446883607535, 1.626142955000567936 ) ) ;
#14261=CARTESIAN_POINT ( 'NONE',  ( -37.72544563604515844, 214.8429017333602360, 4.673758765035156415 ) ) ;
#14265=CARTESIAN_POINT ( 'NONE',  ( -55.93377896937850124, 208.9097554298617183, 4.530955311639234040 ) ) ;
#14266=CARTESIAN_POINT ( 'NONE',  ( -41.49330436395490551, 210.1155267958017134, -6.500000000000000888 ) ) ;
#14272=CARTESIAN_POINT ( 'NONE',  ( -33.17336230271183695, 217.4189793300686233, 4.149950860017807663 ) ) ;
#14288=CARTESIAN_POINT ( 'NONE',  ( -62.27455436395490551, 205.1570982666397356, 4.673758765035198159 ) ) ;
#14307=CARTESIAN_POINT ( 'NONE',  ( -51.77752896937849414, 213.3500491399821613, 5.571401726697954970 ) ) ;
#14309=CARTESIAN_POINT ( 'NONE',  ( -45.44419563604516554, 205.4999999999999716, 0.1155267958017633378 ) ) ;
#14312=CARTESIAN_POINT ( 'NONE',  ( -32.78497103062156981, 204.4285982733020148, -3.350049139982115509 ) ) ;
#14313=CARTESIAN_POINT ( 'NONE',  ( -47.82663769728823411, 202.5810206699313767, 4.149950860017909804 ) ) ;
#14318=CARTESIAN_POINT ( 'NONE',  ( -30.20461230271182274, 208.1428034533959135, -6.469044688360754414 ) ) ;
#14329=CARTESIAN_POINT ( 'NONE',  ( -54.15997103062156981, 215.5714017266979852, 3.350049139982118618 ) ) ;
#14356=CARTESIAN_POINT ( 'NONE',  ( -45.45163769728823411, 213.9548777149308592, -2.149950860017830756 ) ) ;
#14361=CARTESIAN_POINT ( 'NONE',  ( -66.43080436395490551, 203.5000000000000000, -0.1155267958017335561 ) ) ;
#14407=CARTESIAN_POINT ( 'NONE',  ( -38.92038769728823411, 208.1428034533959703, 6.469044688360770401 ) ) ;
#14441=CARTESIAN_POINT ( 'NONE',  ( -45.44419563604516554, 203.5000000000000000, 0.1155267958017914542 ) ) ;
#14445=CARTESIAN_POINT ( 'NONE',  ( -54.35044563604515844, 206.6211998817775566, -3.209657149897419348 ) ) ;
#14446=CARTESIAN_POINT ( 'NONE',  ( -38.72247103062156981, 206.6499508600178672, 5.571401726697986057 ) ) ;
#14452=CARTESIAN_POINT ( 'NONE',  ( -55.54538769728824832, 212.3930949314662371, -8.469044688360781947 ) ) ;
#14458=CARTESIAN_POINT ( 'NONE',  ( -46.04538769728823411, 211.8571965466040012, -6.469044688360769513 ) ) ;
#14470=CARTESIAN_POINT ( 'NONE',  ( -58.31622103062155560, 211.6261429550005744, 6.530955311639227823 ) ) ;
#14488=CARTESIAN_POINT ( 'NONE',  ( -55.14211230271182984, 203.5309553116391896, 1.857196546604092724 ) ) ;
#14490=CARTESIAN_POINT ( 'NONE',  ( -45.04836230271183695, 206.0451222850691977, -2.149950860017851184 ) ) ;
#14493=CARTESIAN_POINT ( 'NONE',  ( -54.35788769728822700, 214.4690446883608104, 1.321298161741840893 ) ) ;
#14494=CARTESIAN_POINT ( 'NONE',  ( -40.30580436395490551, 218.5000000000000000, 0.1155267958017064944 ) ) ;
#14498=CARTESIAN_POINT ( 'NONE',  ( -55.73586230271182984, 205.8500491399821613, 7.418979330068642852 ) ) ;
#14512=CARTESIAN_POINT ( 'NONE',  ( -44.46205436395488420, 214.6737587650352168, 4.842901733360204908 ) ) ;
#14539=CARTESIAN_POINT ( 'NONE',  ( -39.11830436395489841, 209.8844732041982297, 4.499999999999996447 ) ) ;
#14543=CARTESIAN_POINT ( 'NONE',  ( -57.72247103062156270, 206.6499508600178672, 5.571401726697986057 ) ) ;
#14550=VERTEX_POINT ( 'NONE', #32266 ) ;
#14595=CARTESIAN_POINT ( 'NONE',  ( -32.38913769728823411, 206.8500491399821044, -5.686928522499717253 ) ) ;
#14629=CARTESIAN_POINT ( 'NONE',  ( -61.67336230271184405, 217.4189793300686233, 4.149950860017807663 ) ) ;
#14632=CARTESIAN_POINT ( 'NONE',  ( -57.51711230271184405, 214.4690446883608104, -1.321298161741814914 ) ) ;
#14633=CARTESIAN_POINT ( 'NONE',  ( -33.77455436395490551, 205.1570982666397356, 4.673758765035198159 ) ) ;
#14638=CARTESIAN_POINT ( 'NONE',  ( -66.03497103062157692, 202.6965474657331185, -4.350049139982091084 ) ) ;
#14645=CARTESIAN_POINT ( 'NONE',  ( -48.42038769728822700, 208.1428034533959703, 6.469044688360771289 ) ) ;
#14656=CARTESIAN_POINT ( 'NONE',  ( -59.50372103062156981, 216.5309553116391612, -1.626142955000564383 ) ) ;
#14673=CARTESIAN_POINT ( 'NONE',  ( -55.34002896937850124, 204.4285982733020433, 3.350049139982171020 ) ) ;
#14675=CARTESIAN_POINT ( 'NONE',  ( -32.57961230271184405, 211.3212981617417938, 4.469044688360757966 ) ) ;
#14678=CARTESIAN_POINT ( 'NONE',  ( -60.49330436395489130, 210.1155267958017703, -4.499999999999996447 ) ) ;
#14679=CARTESIAN_POINT ( 'NONE',  ( -38.72247103062156981, 205.6499508600178956, 7.303452534266880569 ) ) ;
#14684=CARTESIAN_POINT ( 'NONE',  ( -57.51711230271184405, 218.4690446883607535, -2.393094931466363651 ) ) ;
#14696=CARTESIAN_POINT ( 'NONE',  ( -45.45163769728822700, 215.6869285224996986, -3.149950860017881382 ) ) ;
#14726=CARTESIAN_POINT ( 'NONE',  ( -63.25669563604515844, 209.8844732041982297, -4.499999999999996447 ) ) ;
#14731=CARTESIAN_POINT ( 'NONE',  ( -53.36830436395489841, 209.8844732041982581, 6.500000000000000888 ) ) ;
#14732=CARTESIAN_POINT ( 'NONE',  ( -42.67336230271183695, 217.4189793300686233, 4.149950860017807663 ) ) ;
#14785=CARTESIAN_POINT ( 'NONE',  ( -69.99330436395489130, 210.1155267958017703, -4.499999999999996447 ) ) ;
#14813=( BOUNDED_SURFACE ( )  B_SPLINE_SURFACE ( 3, 2, ( 
 ( #11254, #13922, #34189, #13739, #8234, #21582, #19434, #16764, #25287, #31167, #34374, #13042, #31344, #36838, #22454, #5190, #10881, #24597, #5371, #16950, #28312, #28493, #2536, #8416, #2350, #30287, #35963, #14102, #16583, #8045, #25654, #19621, #19985, #31528, #5553, #36655, #17138, #10001, #10692, #14288, #7172, #18745, #4312, #22270, #15891, #33823, #27436, #5929, #6314, #29431, #11619, #26207, #34927, #14656, #31899, #20166, #23194, #32271, #430, #14470, #2898, #20543, #26024, #23378, #3276, #17886, #28863, #8972, #34742, #17508, #29043, #20357, #53, #8595, #3465, #11808, #8785, #32086, #6117, #9160, #26397, #34556, #3088, #244, #17696, #29236, #23006, #14849, #37388, #11996, #23567, #35112, #20727, #31714, #15036, #26584, #5741, #17321, #613, #25839, #11439, #31466, #30919, #14042, #22949, #11188, #22763, #31650, #22578, #2468, #34123, #36960, #11005, #5313, #36775, #20102, #33760, #22393, #16707, #5489, #16891, #8173, #25226, #14178, #19556, #28254, #19748, #5677, #28799, #5126, #28429, #25591, #31286, #37147, #28066, #2284, #8535, #14225, #33941, #7984, #34311, #31107, #8356, #17072, #17258, #10820, #19928, #13860, #25408, #28611, #2648, #25776, #16518, #2835, #37326, #11376, #34494, #14407, #25963, #22210, #4936, #7800, #19376, #2100, #13679, #20292, #11746, #34675, #9283, #365, #35233, #17635, #31833, #20480, #9095, #28983, #5866, #23687, #11559, #26900, #20857, #17444, #3401, #12307, #548, #12114, #21045, #6436, #32396, #14969, #14595, #29361, #180 ),
 ( #14785, #23133, #29739, #23315, #29553, #26517, #18009, #26705, #3772, #736, #26329, #15346, #32210, #6248, #6623, #11929, #3024, #32583, #26147, #6049, #23881, #34863, #23499, #8903, #15156, #8720, #3592, #35420, #32018, #29168, #9470, #3212, #35047, #18199, #20664, #17826, #15906, #22336, #33331, #24974, #1482, #24796, #7740, #30302, #10577, #4886, #16653, #36724, #13426, #36534, #13246, #22156, #21596, #7371, #16280, #36347, #30680, #33888, #13057, #19324, #10391, #21967, #4700, #33514, #24612, #33702, #16466, #27827, #30861, #28010, #10765, #1857, #7557, #2043, #7931, #27455, #19133, #13621, #25172, #19505, #31051, #5073, #36161, #28198, #10016, #10207, #30496, #2227, #13808, #35979, #21781, #33146, #18943, #4518, #7190, #18759, #4327, #16092, #27644, #1672, #22894, #2598, #31231, #19873, #11689, #17393, #37090, #25538, #25911, #11138, #17204, #8665, #34806, #13987, #2783, #31416, #28557, #25724, #14170, #22715, #19691, #23262, #5620, #5435, #14356, #37456, #26094, #31777, #8120, #37277, #34258, #17018, #8301, #34070, #11323, #10950, #23075, #34441, #11506, #8481, #5259, #20051, #31597, #16838, #28377, #34620, #25356, #3156, #20234, #2414, #28743, #124, #5812, #28934, #8851, #2969, #14539, #20424, #31969, #5999, #17579, #36902, #29112, #22524, #20989, #35362, #3534, #17762, #30062, #12060, #20796, #15099, #24195, #21363, #35177, #9413, #18141, #12250, #29495, #20610, #9223, #1056, #6754, #26460, #14911, #15288, #494, #6567, #35556, #35740, #3342, #29683, #32339 ),
 ( #32523, #6377, #3717, #26841, #15478, #21175, #34995, #26649, #23634, #17952, #680, #23441, #23820, #307, #12442, #871, #24012, #9601, #9038, #32714, #18328, #32150, #6190, #29873, #14726, #26274, #3906, #29303, #27033, #12630, #9786, #32902, #6955, #18523, #11873, #33466, #7140, #21916, #30253, #19456, #4650, #13567, #10345, #27963, #1434, #30634, #18714, #30448, #13378, #35928, #16231, #10529, #22289, #4838, #19082, #27783, #18896, #1809, #27219, #13010, #7508, #4467, #36297, #1994, #4280, #24932, #16046, #27594, #36485, #1624, #15856, #22105, #33654, #7693, #19274, #30815, #16416, #25121, #13195, #36677, #10715, #21549, #24748, #33843, #7881, #4097, #15668, #1244, #27402, #12814, #24383, #24565, #36118, #9970, #33284, #10158, #33097, #21733, #7322, #11639, #8435, #31186, #25679, #31549, #19644, #34576, #13759, #22475, #5573, #16604, #34210, #37230, #10901, #20186, #14309, #31004, #14490, #8805, #26047, #11278, #36857, #22847, #25305, #8254, #5209, #34023, #34396, #8067, #20004, #28512, #17158, #19828, #5024, #23214, #16786, #11460, #28700, #2737, #8617, #34763, #31736, #31366, #28147, #14123, #25861, #74, #5390, #28331, #2921, #2368, #25490, #5763, #13941, #16970, #37042, #17343, #2178, #37410, #23028, #11090, #22666, #28886, #2555, #20560, #35312, #32103, #11826, #15053, #12199, #35691, #23773, #35506, #31920, #29636, #6135, #3857, #29063, #17713, #20378, #14675, #5950, #32290, #17903, #26225, #3672, #262, #20746, #6332, #15242, #17529, #3107, #29448, #3483 ),
 ( #9367, #14866, #23585, #12013, #23397, #24148, #21128, #34945, #26982, #823, #8990, #29252, #20941, #3294, #26601, #632, #26412, #447, #32474, #35127, #6521, #9177, #18096, #26792, #1008, #12392, #23963, #9553, #32666, #6707, #18279, #29823, #15433, #12581, #32851, #12958, #15998, #27170, #36434, #30588, #9743, #30767, #25068, #4790, #4417, #15616, #27546, #4044, #24518, #9920, #12768, #1572, #1194, #24698, #7274, #36250, #36068, #21314, #27913, #35878, #27732, #13144, #10294, #24886, #1942, #10476, #10111, #13513, #30393, #21866, #16366, #21682, #24337, #19223, #21504, #4230, #22053, #33047, #33234, #7095, #13328, #6898, #4603, #33418, #18663, #18473, #7457, #27356, #30203, #19033, #15806, #1387, #16182, #1762, #30014, #33608, #7646, #18848, #8389, #10851, #20136, #7831, #22424, #36625, #30954, #22244, #11038, #34159, #4972, #19958, #16553, #36994, #22612, #31500, #14441, #10664, #8204, #19781, #33792, #25441, #28283, #19406, #28097, #36809, #25625, #31138, #2322, #13893, #2130, #2869, #37358, #13708, #5712, #17107, #25260, #33974, #2500, #8014, #31317, #5345, #5157, #19590, #16923, #16736, #22794, #28464, #14074, #37181, #11224, #5523, #34345, #28649, #2685, #14261, #25811, #11412, #22980, #34530, #8569, #31683, #17293, #28833, #20699, #26366, #32243, #23918, #5901, #400, #6283, #11966, #3247, #14821, #9134, #3059, #35460, #26, #26179, #20517, #35265, #17859, #23538, #29014, #3809, #23349, #32057, #35082, #9510, #32623, #8942, #29402, #3434, #15003, #26554 ),
 ( #6086, #29206, #17670, #23167, #29779, #26743, #17482, #6661, #6476, #34709, #216, #583, #20328, #12151, #23728, #9321, #8755, #20890, #31869, #32433, #18048, #29590, #3626, #34899, #15196, #777, #12344, #18235, #21085, #11781, #25997, #11591, #14629, #18991, #35651, #6851, #15954, #965, #18620, #21640, #32810, #4564, #36208, #15387, #36395, #30728, #10441, #10068, #21273, #33192, #9696, #30162, #15573, #18427, #7235, #29970, #30353, #12916, #4376, #4191, #26935, #33568, #4000, #33382, #18809, #27507, #30547, #7604, #16140, #15766, #19181, #36025, #1529, #22015, #27317, #27129, #24844, #1155, #9880, #27690, #12541, #13103, #1344, #24658, #21460, #12727, #24295, #24479, #35838, #33001, #10252, #24106, #21828, #1719, #7421, #7052, #13288, #20615, #312, #36952, #10624, #10998, #36584, #7977, #4930, #7791, #22571, #22203, #19741, #2277, #31279, #19550, #16325, #23447, #30911, #22756, #8167, #5308, #20430, #35000, #31974, #31099, #9043, #25402, #34117, #11879, #5120, #33752, #14732, #19369, #36770, #6004, #16512, #16699, #28059, #8856, #4752, #37140, #16885, #2094, #1904, #28421, #22385, #13670, #2462, #25220, #10814, #14035, #25585, #27873, #11183, #17585, #13474, #34812, #33935, #26280, #25026, #28248, #13854, #29117, #3161, #6572, #29688, #26466, #15483, #499, #32529, #18147, #27038, #9975, #32155, #3722, #15294, #6195, #20994, #23825, #14917, #17767, #32345, #21180, #26654, #35367, #9419, #29309, #35933, #32907, #12065, #1249, #12635, #3348, #6382, #35562, #23639 ),
 ( #18333, #26846, #876, #12448, #3540, #3911, #6759, #9606, #12819, #32720, #29878, #6961, #1062, #35182, #24017, #17957, #685, #29500, #9228, #15104, #20802, #24200, #35745, #9791, #12256, #21368, #18529, #30067, #4102, #15674, #27224, #24388, #24936, #30819, #30259, #13383, #22294, #10534, #22110, #31009, #16422, #19279, #36491, #24569, #1815, #10163, #36862, #33659, #5030, #27788, #7887, #18902, #7699, #36123, #10349, #4843, #15862, #27969, #2000, #2182, #33847, #13573, #25125, #36302, #36682, #7145, #30454, #10720, #21922, #16237, #19460, #21738, #16609, #33471, #7514, #28152, #19087, #33289, #13764, #25310, #21555, #33102, #18719, #4285, #27407, #30638, #1439, #13015, #7328, #4655, #4472, #16051, #27598, #1629, #13201, #24753, #8810, #22481, #11096, #5394, #20191, #31554, #37234, #13947, #26229, #8259, #16974, #11282, #20382, #17534, #31371, #5578, #14313, #8439, #25684, #16791, #28516, #34768, #2925, #22670, #34214, #11465, #19832, #2741, #31741, #31924, #37048, #25866, #2559, #14128, #22852, #34402, #20008, #5214, #5955, #28704, #17164, #19649, #37415, #34028, #8622, #23034, #34581, #5768, #31191, #17348, #28891, #28336, #8074, #10907, #14494, #26051, #78, #2373, #11643, #23219, #29069, #3113, #14679, #25496, #35511, #29641, #3298, #18100, #26417, #15621, #829, #9747, #6526, #24152, #35131, #26797, #14870, #26607, #9557, #32107, #12396, #6713, #18479, #1012, #15246, #23968, #15058, #21133, #23401, #9182, #3677, #636, #32479, #35695, #451, #32670, #12206 ),
 ( #18284, #29827, #3864, #12586, #15437, #23779, #26986, #21320, #17718, #35317, #32857, #9371, #20946, #6907, #30019, #12019, #4049, #11830, #23589, #32297, #267, #34949, #8995, #20751, #20565, #6336, #17908, #6141, #29258, #29452, #3487, #10298, #30592, #24703, #4422, #33052, #21687, #13518, #19228, #1391, #27361, #27736, #12965, #19041, #10481, #36629, #15812, #4607, #33239, #30399, #27551, #16004, #24523, #21508, #25075, #7461, #7278, #16187, #1767, #27917, #33612, #9926, #1578, #36072, #18852, #10116, #13150, #36255, #35883, #21870, #24342, #13333, #33423, #24891, #36441, #22060, #7651, #30772, #4794, #7837, #16372, #1947, #10669, #22248, #33799, #19409, #7099, #18667, #30959, #4977, #27175, #30208, #1199, #12772, #4235, #16558, #31, #31876, #11596, #11228, #22431, #22799, #10858, #19785, #16741, #19595, #34350, #33979, #31505, #14079, #5527, #31322, #28105, #34715, #5163, #34534, #19962, #17114, #31688, #8760, #5717, #5350, #20334, #37185, #8393, #23171, #16927, #8020, #26002, #31143, #11042, #17298, #28288, #28469, #2326, #20142, #2136, #11416, #28653, #13898, #13715, #2690, #34165, #25446, #14266, #36999, #22618, #25817, #37363, #25264, #22984, #28839, #36815, #8573, #8209, #2508, #25629, #2873, #14446, #221, #29018, #17863, #3439, #11785, #26750, #23353, #6287, #29408, #781, #21278, #5906, #15008, #26560, #17486, #32247, #35088, #26183, #3064, #6090, #32437, #404, #9138, #20703, #14633, #9701, #6665, #34905, #12546, #23923, #8949, #17674, #9325, #20522 ) ),
 .UNSPECIFIED., .T., .F., .F. ) 
 B_SPLINE_SURFACE_WITH_KNOTS ( ( 4, 3, 4 ),
 ( 3, 2, 2, 2, 2, 2, 2, 2, 2, 2, 2, 2, 2, 2, 2, 2, 2, 2, 2, 2, 2, 2, 2, 2, 2, 2, 2, 2, 2, 2, 2, 2, 2, 2, 2, 2, 2, 2, 2, 2, 2, 2, 2, 2, 2, 2, 2, 2, 2, 2, 2, 2, 2, 2, 2, 2, 2, 2, 2, 2, 2, 2, 2, 2, 2, 2, 2, 2, 2, 2, 2, 2, 2, 2, 2, 2, 2, 2, 2, 2, 2, 2, 2, 2, 2, 2, 2, 2, 2, 2, 2, 2, 2, 2, 2, 2, 3 ),
 ( 0.000000000000000000, 0.5000000000000000000, 1.000000000000000000 ),
 ( 0.000000000000000000, 0.01041666666666666609, 0.02083333333333333218, 0.03125000000000000000, 0.04166666666666666435, 0.05208333333333333565, 0.06250000000000000000, 0.07291666666666667129, 0.08333333333333332871, 0.09375000000000000000, 0.1041666666666666713, 0.1145833333333333287, 0.1250000000000000000, 0.1354166666666666574, 0.1458333333333333426, 0.1562500000000000000, 0.1666666666666666574, 0.1770833333333333426, 0.1875000000000000000, 0.1979166666666666574, 0.2083333333333333426, 0.2187500000000000000, 0.2291666666666666574, 0.2395833333333333426, 0.2500000000000000000, 0.2604166666666666852, 0.2708333333333333148, 0.2812500000000000000, 0.2916666666666666852, 0.3020833333333333148, 0.3125000000000000000, 0.3229166666666666852, 0.3333333333333333148, 0.3437500000000000000, 0.3541666666666666852, 0.3645833333333333148, 0.3750000000000000000, 0.3854166666666666852, 0.3958333333333333148, 0.4062500000000000000, 0.4166666666666666852, 0.4270833333333333148, 0.4375000000000000000, 0.4479166666666666852, 0.4583333333333333148, 0.4687500000000000000, 0.4791666666666666852, 0.4895833333333333148, 0.5000000000000000000, 0.5104166666666666297, 0.5208333333333333703, 0.5312500000000000000, 0.5416666666666666297, 0.5520833333333333703, 0.5625000000000000000, 0.5729166666666666297, 0.5833333333333333703, 0.5937500000000000000, 0.6041666666666666297, 0.6145833333333333703, 0.6250000000000000000, 0.6354166666666666297, 0.6458333333333333703, 0.6562500000000000000, 0.6666666666666666297, 0.6770833333333333703, 0.6875000000000000000, 0.6979166666666666297, 0.7083333333333333703, 0.7187500000000000000, 0.7291666666666666297, 0.7395833333333333703, 0.7500000000000000000, 0.7604166666666666297, 0.7708333333333333703, 0.7812500000000000000, 0.7916666666666666297, 0.8020833333333333703, 0.8125000000000000000, 0.8229166666666666297, 0.8333333333333333703, 0.8437500000000000000, 0.8541666666666666297, 0.8645833333333333703, 0.8750000000000000000, 0.8854166666666666297, 0.8958333333333333703, 0.9062500000000000000, 0.9166666666666666297, 0.9270833333333333703, 0.9375000000000000000, 0.9479166666666666297, 0.9583333333333333703, 0.9687500000000000000, 0.9791666666666666297, 0.9895833333333333703, 1.000000000000000000 ),
 .UNSPECIFIED. ) 
 GEOMETRIC_REPRESENTATION_ITEM ( )  RATIONAL_B_SPLINE_SURFACE ( (
 ( 1.000000000000000000, 0.9659258262890683122, 1.000000000000000000, 0.9659258262890683122, 1.000000000000000000, 0.9659258262890683122, 1.000000000000000000, 0.9659258262890683122, 1.000000000000000000, 0.9659258262890683122, 1.000000000000000000, 0.9659258262890683122, 1.000000000000000000, 0.9659258262890683122, 1.000000000000000000, 0.9659258262890683122, 1.000000000000000000, 0.9659258262890683122, 1.000000000000000000, 0.9659258262890683122, 1.000000000000000000, 0.9659258262890683122, 1.000000000000000000, 0.9659258262890683122, 1.000000000000000000, 0.9659258262890683122, 1.000000000000000000, 0.9659258262890683122, 1.000000000000000000, 0.9659258262890683122, 1.000000000000000000, 0.9659258262890683122, 1.000000000000000000, 0.9659258262890683122, 1.000000000000000000, 0.9659258262890683122, 1.000000000000000000, 0.9659258262890683122, 1.000000000000000000, 0.9659258262890683122, 1.000000000000000000, 0.9659258262890683122, 1.000000000000000000, 0.9659258262890683122, 1.000000000000000000, 0.9659258262890683122, 1.000000000000000000, 0.9659258262890683122, 1.000000000000000000, 0.9659258262890683122, 1.000000000000000000, 0.9659258262890683122, 1.000000000000000000, 0.9659258262890683122, 1.000000000000000000, 0.9659258262890683122, 1.000000000000000000, 0.9659258262890683122, 1.000000000000000000, 0.9659258262890683122, 1.000000000000000000, 0.9659258262890683122, 1.000000000000000000, 0.9659258262890683122, 1.000000000000000000, 0.9659258262890683122, 1.000000000000000000, 0.9659258262890683122, 1.000000000000000000, 0.9659258262890683122, 1.000000000000000000, 0.9659258262890683122, 1.000000000000000000, 0.9659258262890683122, 1.000000000000000000, 0.9659258262890683122, 1.000000000000000000, 0.9659258262890683122, 1.000000000000000000, 0.9659258262890683122, 1.000000000000000000, 0.9659258262890683122, 1.000000000000000000, 0.9659258262890683122, 1.000000000000000000, 0.9659258262890683122, 1.000000000000000000, 0.9659258262890683122, 1.000000000000000000, 0.9659258262890683122, 1.000000000000000000, 0.9659258262890683122, 1.000000000000000000, 0.9659258262890683122, 1.000000000000000000, 0.9659258262890683122, 1.000000000000000000, 0.9659258262890683122, 1.000000000000000000, 0.9659258262890683122, 1.000000000000000000, 0.9659258262890683122, 1.000000000000000000, 0.9659258262890683122, 1.000000000000000000, 0.9659258262890683122, 1.000000000000000000, 0.9659258262890683122, 1.000000000000000000, 0.9659258262890683122, 1.000000000000000000, 0.9659258262890683122, 1.000000000000000000, 0.9659258262890683122, 1.000000000000000000, 0.9659258262890683122, 1.000000000000000000, 0.9659258262890683122, 1.000000000000000000, 0.9659258262890683122, 1.000000000000000000, 0.9659258262890683122, 1.000000000000000000, 0.9659258262890683122, 1.000000000000000000, 0.9659258262890683122, 1.000000000000000000, 0.9659258262890683122, 1.000000000000000000, 0.9659258262890683122, 1.000000000000000000, 0.9659258262890683122, 1.000000000000000000, 0.9659258262890683122, 1.000000000000000000, 0.9659258262890683122, 1.000000000000000000, 0.9659258262890683122, 1.000000000000000000, 0.9659258262890683122, 1.000000000000000000, 0.9659258262890683122, 1.000000000000000000, 0.9659258262890683122, 1.000000000000000000, 0.9659258262890683122, 1.000000000000000000, 0.9659258262890683122, 1.000000000000000000, 0.9659258262890683122, 1.000000000000000000, 0.9659258262890683122, 1.000000000000000000, 0.9659258262890683122, 1.000000000000000000, 0.9659258262890683122, 1.000000000000000000, 0.9659258262890683122, 1.000000000000000000, 0.9659258262890683122, 1.000000000000000000, 0.9659258262890683122, 1.000000000000000000, 0.9659258262890683122, 1.000000000000000000, 0.9659258262890683122, 1.000000000000000000, 0.9659258262890683122, 1.000000000000000000, 0.9659258262890683122, 1.000000000000000000, 0.9659258262890683122, 1.000000000000000000, 0.9659258262890683122, 1.000000000000000000, 0.9659258262890683122, 1.000000000000000000, 0.9659258262890683122, 1.000000000000000000, 0.9659258262890683122, 1.000000000000000000, 0.9659258262890683122, 1.000000000000000000, 0.9659258262890683122, 1.000000000000000000, 0.9659258262890683122, 1.000000000000000000, 0.9659258262890683122, 1.000000000000000000, 0.9659258262890683122, 1.000000000000000000, 0.9659258262890683122, 1.000000000000000000),
 ( 0.3333333333333333703, 0.3219752754296894559, 0.3333333333333333703, 0.3219752754296894559, 0.3333333333333333703, 0.3219752754296894559, 0.3333333333333333703, 0.3219752754296894559, 0.3333333333333333703, 0.3219752754296894559, 0.3333333333333333703, 0.3219752754296894559, 0.3333333333333333703, 0.3219752754296894559, 0.3333333333333333703, 0.3219752754296894559, 0.3333333333333333703, 0.3219752754296894559, 0.3333333333333333703, 0.3219752754296894559, 0.3333333333333333703, 0.3219752754296894559, 0.3333333333333333703, 0.3219752754296894559, 0.3333333333333333703, 0.3219752754296894559, 0.3333333333333333703, 0.3219752754296894559, 0.3333333333333333703, 0.3219752754296894559, 0.3333333333333333703, 0.3219752754296894559, 0.3333333333333333703, 0.3219752754296894559, 0.3333333333333333703, 0.3219752754296894559, 0.3333333333333333703, 0.3219752754296894559, 0.3333333333333333703, 0.3219752754296894559, 0.3333333333333333703, 0.3219752754296894559, 0.3333333333333333703, 0.3219752754296894559, 0.3333333333333333703, 0.3219752754296894559, 0.3333333333333333703, 0.3219752754296894559, 0.3333333333333333703, 0.3219752754296894559, 0.3333333333333333703, 0.3219752754296894559, 0.3333333333333333703, 0.3219752754296894559, 0.3333333333333333703, 0.3219752754296894559, 0.3333333333333333703, 0.3219752754296894559, 0.3333333333333333703, 0.3219752754296894559, 0.3333333333333333703, 0.3219752754296894559, 0.3333333333333333703, 0.3219752754296894559, 0.3333333333333333703, 0.3219752754296894559, 0.3333333333333333703, 0.3219752754296894559, 0.3333333333333333703, 0.3219752754296894559, 0.3333333333333333703, 0.3219752754296894559, 0.3333333333333333703, 0.3219752754296894559, 0.3333333333333333703, 0.3219752754296894559, 0.3333333333333333703, 0.3219752754296894559, 0.3333333333333333703, 0.3219752754296894559, 0.3333333333333333703, 0.3219752754296894559, 0.3333333333333333703, 0.3219752754296894559, 0.3333333333333333703, 0.3219752754296894559, 0.3333333333333333703, 0.3219752754296894559, 0.3333333333333333703, 0.3219752754296894559, 0.3333333333333333703, 0.3219752754296894559, 0.3333333333333333703, 0.3219752754296894559, 0.3333333333333333703, 0.3219752754296894559, 0.3333333333333333703, 0.3219752754296894559, 0.3333333333333333703, 0.3219752754296894559, 0.3333333333333333703, 0.3219752754296894559, 0.3333333333333333703, 0.3219752754296894559, 0.3333333333333333703, 0.3219752754296894559, 0.3333333333333333703, 0.3219752754296894559, 0.3333333333333333703, 0.3219752754296894559, 0.3333333333333333703, 0.3219752754296894559, 0.3333333333333333703, 0.3219752754296894559, 0.3333333333333333703, 0.3219752754296894559, 0.3333333333333333703, 0.3219752754296894559, 0.3333333333333333703, 0.3219752754296894559, 0.3333333333333333703, 0.3219752754296894559, 0.3333333333333333703, 0.3219752754296894559, 0.3333333333333333703, 0.3219752754296894559, 0.3333333333333333703, 0.3219752754296894559, 0.3333333333333333703, 0.3219752754296894559, 0.3333333333333333703, 0.3219752754296894559, 0.3333333333333333703, 0.3219752754296894559, 0.3333333333333333703, 0.3219752754296894559, 0.3333333333333333703, 0.3219752754296894559, 0.3333333333333333703, 0.3219752754296894559, 0.3333333333333333703, 0.3219752754296894559, 0.3333333333333333703, 0.3219752754296894559, 0.3333333333333333703, 0.3219752754296894559, 0.3333333333333333703, 0.3219752754296894559, 0.3333333333333333703, 0.3219752754296894559, 0.3333333333333333703, 0.3219752754296894559, 0.3333333333333333703, 0.3219752754296894559, 0.3333333333333333703, 0.3219752754296894559, 0.3333333333333333703, 0.3219752754296894559, 0.3333333333333333703, 0.3219752754296894559, 0.3333333333333333703, 0.3219752754296894559, 0.3333333333333333703, 0.3219752754296894559, 0.3333333333333333703, 0.3219752754296894559, 0.3333333333333333703, 0.3219752754296894559, 0.3333333333333333703, 0.3219752754296894559, 0.3333333333333333703, 0.3219752754296894559, 0.3333333333333333703, 0.3219752754296894559, 0.3333333333333333703, 0.3219752754296894559, 0.3333333333333333703, 0.3219752754296894559, 0.3333333333333333703, 0.3219752754296894559, 0.3333333333333333703, 0.3219752754296894559, 0.3333333333333333703, 0.3219752754296894559, 0.3333333333333333703, 0.3219752754296894559, 0.3333333333333333703, 0.3219752754296894559, 0.3333333333333333703, 0.3219752754296894559, 0.3333333333333333703, 0.3219752754296894559, 0.3333333333333333703),
 ( 0.3333333333333333703, 0.3219752754296894559, 0.3333333333333333703, 0.3219752754296894559, 0.3333333333333333703, 0.3219752754296894559, 0.3333333333333333703, 0.3219752754296894559, 0.3333333333333333703, 0.3219752754296894559, 0.3333333333333333703, 0.3219752754296894559, 0.3333333333333333703, 0.3219752754296894559, 0.3333333333333333703, 0.3219752754296894559, 0.3333333333333333703, 0.3219752754296894559, 0.3333333333333333703, 0.3219752754296894559, 0.3333333333333333703, 0.3219752754296894559, 0.3333333333333333703, 0.3219752754296894559, 0.3333333333333333703, 0.3219752754296894559, 0.3333333333333333703, 0.3219752754296894559, 0.3333333333333333703, 0.3219752754296894559, 0.3333333333333333703, 0.3219752754296894559, 0.3333333333333333703, 0.3219752754296894559, 0.3333333333333333703, 0.3219752754296894559, 0.3333333333333333703, 0.3219752754296894559, 0.3333333333333333703, 0.3219752754296894559, 0.3333333333333333703, 0.3219752754296894559, 0.3333333333333333703, 0.3219752754296894559, 0.3333333333333333703, 0.3219752754296894559, 0.3333333333333333703, 0.3219752754296894559, 0.3333333333333333703, 0.3219752754296894559, 0.3333333333333333703, 0.3219752754296894559, 0.3333333333333333703, 0.3219752754296894559, 0.3333333333333333703, 0.3219752754296894559, 0.3333333333333333703, 0.3219752754296894559, 0.3333333333333333703, 0.3219752754296894559, 0.3333333333333333703, 0.3219752754296894559, 0.3333333333333333703, 0.3219752754296894559, 0.3333333333333333703, 0.3219752754296894559, 0.3333333333333333703, 0.3219752754296894559, 0.3333333333333333703, 0.3219752754296894559, 0.3333333333333333703, 0.3219752754296894559, 0.3333333333333333703, 0.3219752754296894559, 0.3333333333333333703, 0.3219752754296894559, 0.3333333333333333703, 0.3219752754296894559, 0.3333333333333333703, 0.3219752754296894559, 0.3333333333333333703, 0.3219752754296894559, 0.3333333333333333703, 0.3219752754296894559, 0.3333333333333333703, 0.3219752754296894559, 0.3333333333333333703, 0.3219752754296894559, 0.3333333333333333703, 0.3219752754296894559, 0.3333333333333333703, 0.3219752754296894559, 0.3333333333333333703, 0.3219752754296894559, 0.3333333333333333703, 0.3219752754296894559, 0.3333333333333333703, 0.3219752754296894559, 0.3333333333333333703, 0.3219752754296894559, 0.3333333333333333703, 0.3219752754296894559, 0.3333333333333333703, 0.3219752754296894559, 0.3333333333333333703, 0.3219752754296894559, 0.3333333333333333703, 0.3219752754296894559, 0.3333333333333333703, 0.3219752754296894559, 0.3333333333333333703, 0.3219752754296894559, 0.3333333333333333703, 0.3219752754296894559, 0.3333333333333333703, 0.3219752754296894559, 0.3333333333333333703, 0.3219752754296894559, 0.3333333333333333703, 0.3219752754296894559, 0.3333333333333333703, 0.3219752754296894559, 0.3333333333333333703, 0.3219752754296894559, 0.3333333333333333703, 0.3219752754296894559, 0.3333333333333333703, 0.3219752754296894559, 0.3333333333333333703, 0.3219752754296894559, 0.3333333333333333703, 0.3219752754296894559, 0.3333333333333333703, 0.3219752754296894559, 0.3333333333333333703, 0.3219752754296894559, 0.3333333333333333703, 0.3219752754296894559, 0.3333333333333333703, 0.3219752754296894559, 0.3333333333333333703, 0.3219752754296894559, 0.3333333333333333703, 0.3219752754296894559, 0.3333333333333333703, 0.3219752754296894559, 0.3333333333333333703, 0.3219752754296894559, 0.3333333333333333703, 0.3219752754296894559, 0.3333333333333333703, 0.3219752754296894559, 0.3333333333333333703, 0.3219752754296894559, 0.3333333333333333703, 0.3219752754296894559, 0.3333333333333333703, 0.3219752754296894559, 0.3333333333333333703, 0.3219752754296894559, 0.3333333333333333703, 0.3219752754296894559, 0.3333333333333333703, 0.3219752754296894559, 0.3333333333333333703, 0.3219752754296894559, 0.3333333333333333703, 0.3219752754296894559, 0.3333333333333333703, 0.3219752754296894559, 0.3333333333333333703, 0.3219752754296894559, 0.3333333333333333703, 0.3219752754296894559, 0.3333333333333333703, 0.3219752754296894559, 0.3333333333333333703, 0.3219752754296894559, 0.3333333333333333703, 0.3219752754296894559, 0.3333333333333333703, 0.3219752754296894559, 0.3333333333333333703, 0.3219752754296894559, 0.3333333333333333703, 0.3219752754296894559, 0.3333333333333333703, 0.3219752754296894559, 0.3333333333333333703, 0.3219752754296894559, 0.3333333333333333703, 0.3219752754296894559, 0.3333333333333333703),
 ( 1.000000000000000000, 0.9659258262890683122, 1.000000000000000000, 0.9659258262890683122, 1.000000000000000000, 0.9659258262890683122, 1.000000000000000000, 0.9659258262890683122, 1.000000000000000000, 0.9659258262890683122, 1.000000000000000000, 0.9659258262890683122, 1.000000000000000000, 0.9659258262890683122, 1.000000000000000000, 0.9659258262890683122, 1.000000000000000000, 0.9659258262890683122, 1.000000000000000000, 0.9659258262890683122, 1.000000000000000000, 0.9659258262890683122, 1.000000000000000000, 0.9659258262890683122, 1.000000000000000000, 0.9659258262890683122, 1.000000000000000000, 0.9659258262890683122, 1.000000000000000000, 0.9659258262890683122, 1.000000000000000000, 0.9659258262890683122, 1.000000000000000000, 0.9659258262890683122, 1.000000000000000000, 0.9659258262890683122, 1.000000000000000000, 0.9659258262890683122, 1.000000000000000000, 0.9659258262890683122, 1.000000000000000000, 0.9659258262890683122, 1.000000000000000000, 0.9659258262890683122, 1.000000000000000000, 0.9659258262890683122, 1.000000000000000000, 0.9659258262890683122, 1.000000000000000000, 0.9659258262890683122, 1.000000000000000000, 0.9659258262890683122, 1.000000000000000000, 0.9659258262890683122, 1.000000000000000000, 0.9659258262890683122, 1.000000000000000000, 0.9659258262890683122, 1.000000000000000000, 0.9659258262890683122, 1.000000000000000000, 0.9659258262890683122, 1.000000000000000000, 0.9659258262890683122, 1.000000000000000000, 0.9659258262890683122, 1.000000000000000000, 0.9659258262890683122, 1.000000000000000000, 0.9659258262890683122, 1.000000000000000000, 0.9659258262890683122, 1.000000000000000000, 0.9659258262890683122, 1.000000000000000000, 0.9659258262890683122, 1.000000000000000000, 0.9659258262890683122, 1.000000000000000000, 0.9659258262890683122, 1.000000000000000000, 0.9659258262890683122, 1.000000000000000000, 0.9659258262890683122, 1.000000000000000000, 0.9659258262890683122, 1.000000000000000000, 0.9659258262890683122, 1.000000000000000000, 0.9659258262890683122, 1.000000000000000000, 0.9659258262890683122, 1.000000000000000000, 0.9659258262890683122, 1.000000000000000000, 0.9659258262890683122, 1.000000000000000000, 0.9659258262890683122, 1.000000000000000000, 0.9659258262890683122, 1.000000000000000000, 0.9659258262890683122, 1.000000000000000000, 0.9659258262890683122, 1.000000000000000000, 0.9659258262890683122, 1.000000000000000000, 0.9659258262890683122, 1.000000000000000000, 0.9659258262890683122, 1.000000000000000000, 0.9659258262890683122, 1.000000000000000000, 0.9659258262890683122, 1.000000000000000000, 0.9659258262890683122, 1.000000000000000000, 0.9659258262890683122, 1.000000000000000000, 0.9659258262890683122, 1.000000000000000000, 0.9659258262890683122, 1.000000000000000000, 0.9659258262890683122, 1.000000000000000000, 0.9659258262890683122, 1.000000000000000000, 0.9659258262890683122, 1.000000000000000000, 0.9659258262890683122, 1.000000000000000000, 0.9659258262890683122, 1.000000000000000000, 0.9659258262890683122, 1.000000000000000000, 0.9659258262890683122, 1.000000000000000000, 0.9659258262890683122, 1.000000000000000000, 0.9659258262890683122, 1.000000000000000000, 0.9659258262890683122, 1.000000000000000000, 0.9659258262890683122, 1.000000000000000000, 0.9659258262890683122, 1.000000000000000000, 0.9659258262890683122, 1.000000000000000000, 0.9659258262890683122, 1.000000000000000000, 0.9659258262890683122, 1.000000000000000000, 0.9659258262890683122, 1.000000000000000000, 0.9659258262890683122, 1.000000000000000000, 0.9659258262890683122, 1.000000000000000000, 0.9659258262890683122, 1.000000000000000000, 0.9659258262890683122, 1.000000000000000000, 0.9659258262890683122, 1.000000000000000000, 0.9659258262890683122, 1.000000000000000000, 0.9659258262890683122, 1.000000000000000000, 0.9659258262890683122, 1.000000000000000000, 0.9659258262890683122, 1.000000000000000000, 0.9659258262890683122, 1.000000000000000000, 0.9659258262890683122, 1.000000000000000000, 0.9659258262890683122, 1.000000000000000000, 0.9659258262890683122, 1.000000000000000000, 0.9659258262890683122, 1.000000000000000000, 0.9659258262890683122, 1.000000000000000000, 0.9659258262890683122, 1.000000000000000000, 0.9659258262890683122, 1.000000000000000000, 0.9659258262890683122, 1.000000000000000000, 0.9659258262890683122, 1.000000000000000000),
 ( 0.3333333333333333703, 0.3219752754296894559, 0.3333333333333333703, 0.3219752754296894559, 0.3333333333333333703, 0.3219752754296894559, 0.3333333333333333703, 0.3219752754296894559, 0.3333333333333333703, 0.3219752754296894559, 0.3333333333333333703, 0.3219752754296894559, 0.3333333333333333703, 0.3219752754296894559, 0.3333333333333333703, 0.3219752754296894559, 0.3333333333333333703, 0.3219752754296894559, 0.3333333333333333703, 0.3219752754296894559, 0.3333333333333333703, 0.3219752754296894559, 0.3333333333333333703, 0.3219752754296894559, 0.3333333333333333703, 0.3219752754296894559, 0.3333333333333333703, 0.3219752754296894559, 0.3333333333333333703, 0.3219752754296894559, 0.3333333333333333703, 0.3219752754296894559, 0.3333333333333333703, 0.3219752754296894559, 0.3333333333333333703, 0.3219752754296894559, 0.3333333333333333703, 0.3219752754296894559, 0.3333333333333333703, 0.3219752754296894559, 0.3333333333333333703, 0.3219752754296894559, 0.3333333333333333703, 0.3219752754296894559, 0.3333333333333333703, 0.3219752754296894559, 0.3333333333333333703, 0.3219752754296894559, 0.3333333333333333703, 0.3219752754296894559, 0.3333333333333333703, 0.3219752754296894559, 0.3333333333333333703, 0.3219752754296894559, 0.3333333333333333703, 0.3219752754296894559, 0.3333333333333333703, 0.3219752754296894559, 0.3333333333333333703, 0.3219752754296894559, 0.3333333333333333703, 0.3219752754296894559, 0.3333333333333333703, 0.3219752754296894559, 0.3333333333333333703, 0.3219752754296894559, 0.3333333333333333703, 0.3219752754296894559, 0.3333333333333333703, 0.3219752754296894559, 0.3333333333333333703, 0.3219752754296894559, 0.3333333333333333703, 0.3219752754296894559, 0.3333333333333333703, 0.3219752754296894559, 0.3333333333333333703, 0.3219752754296894559, 0.3333333333333333703, 0.3219752754296894559, 0.3333333333333333703, 0.3219752754296894559, 0.3333333333333333703, 0.3219752754296894559, 0.3333333333333333703, 0.3219752754296894559, 0.3333333333333333703, 0.3219752754296894559, 0.3333333333333333703, 0.3219752754296894559, 0.3333333333333333703, 0.3219752754296894559, 0.3333333333333333703, 0.3219752754296894559, 0.3333333333333333703, 0.3219752754296894559, 0.3333333333333333703, 0.3219752754296894559, 0.3333333333333333703, 0.3219752754296894559, 0.3333333333333333703, 0.3219752754296894559, 0.3333333333333333703, 0.3219752754296894559, 0.3333333333333333703, 0.3219752754296894559, 0.3333333333333333703, 0.3219752754296894559, 0.3333333333333333703, 0.3219752754296894559, 0.3333333333333333703, 0.3219752754296894559, 0.3333333333333333703, 0.3219752754296894559, 0.3333333333333333703, 0.3219752754296894559, 0.3333333333333333703, 0.3219752754296894559, 0.3333333333333333703, 0.3219752754296894559, 0.3333333333333333703, 0.3219752754296894559, 0.3333333333333333703, 0.3219752754296894559, 0.3333333333333333703, 0.3219752754296894559, 0.3333333333333333703, 0.3219752754296894559, 0.3333333333333333703, 0.3219752754296894559, 0.3333333333333333703, 0.3219752754296894559, 0.3333333333333333703, 0.3219752754296894559, 0.3333333333333333703, 0.3219752754296894559, 0.3333333333333333703, 0.3219752754296894559, 0.3333333333333333703, 0.3219752754296894559, 0.3333333333333333703, 0.3219752754296894559, 0.3333333333333333703, 0.3219752754296894559, 0.3333333333333333703, 0.3219752754296894559, 0.3333333333333333703, 0.3219752754296894559, 0.3333333333333333703, 0.3219752754296894559, 0.3333333333333333703, 0.3219752754296894559, 0.3333333333333333703, 0.3219752754296894559, 0.3333333333333333703, 0.3219752754296894559, 0.3333333333333333703, 0.3219752754296894559, 0.3333333333333333703, 0.3219752754296894559, 0.3333333333333333703, 0.3219752754296894559, 0.3333333333333333703, 0.3219752754296894559, 0.3333333333333333703, 0.3219752754296894559, 0.3333333333333333703, 0.3219752754296894559, 0.3333333333333333703, 0.3219752754296894559, 0.3333333333333333703, 0.3219752754296894559, 0.3333333333333333703, 0.3219752754296894559, 0.3333333333333333703, 0.3219752754296894559, 0.3333333333333333703, 0.3219752754296894559, 0.3333333333333333703, 0.3219752754296894559, 0.3333333333333333703, 0.3219752754296894559, 0.3333333333333333703, 0.3219752754296894559, 0.3333333333333333703, 0.3219752754296894559, 0.3333333333333333703, 0.3219752754296894559, 0.3333333333333333703, 0.3219752754296894559, 0.3333333333333333703, 0.3219752754296894559, 0.3333333333333333703),
 ( 0.3333333333333333703, 0.3219752754296894559, 0.3333333333333333703, 0.3219752754296894559, 0.3333333333333333703, 0.3219752754296894559, 0.3333333333333333703, 0.3219752754296894559, 0.3333333333333333703, 0.3219752754296894559, 0.3333333333333333703, 0.3219752754296894559, 0.3333333333333333703, 0.3219752754296894559, 0.3333333333333333703, 0.3219752754296894559, 0.3333333333333333703, 0.3219752754296894559, 0.3333333333333333703, 0.3219752754296894559, 0.3333333333333333703, 0.3219752754296894559, 0.3333333333333333703, 0.3219752754296894559, 0.3333333333333333703, 0.3219752754296894559, 0.3333333333333333703, 0.3219752754296894559, 0.3333333333333333703, 0.3219752754296894559, 0.3333333333333333703, 0.3219752754296894559, 0.3333333333333333703, 0.3219752754296894559, 0.3333333333333333703, 0.3219752754296894559, 0.3333333333333333703, 0.3219752754296894559, 0.3333333333333333703, 0.3219752754296894559, 0.3333333333333333703, 0.3219752754296894559, 0.3333333333333333703, 0.3219752754296894559, 0.3333333333333333703, 0.3219752754296894559, 0.3333333333333333703, 0.3219752754296894559, 0.3333333333333333703, 0.3219752754296894559, 0.3333333333333333703, 0.3219752754296894559, 0.3333333333333333703, 0.3219752754296894559, 0.3333333333333333703, 0.3219752754296894559, 0.3333333333333333703, 0.3219752754296894559, 0.3333333333333333703, 0.3219752754296894559, 0.3333333333333333703, 0.3219752754296894559, 0.3333333333333333703, 0.3219752754296894559, 0.3333333333333333703, 0.3219752754296894559, 0.3333333333333333703, 0.3219752754296894559, 0.3333333333333333703, 0.3219752754296894559, 0.3333333333333333703, 0.3219752754296894559, 0.3333333333333333703, 0.3219752754296894559, 0.3333333333333333703, 0.3219752754296894559, 0.3333333333333333703, 0.3219752754296894559, 0.3333333333333333703, 0.3219752754296894559, 0.3333333333333333703, 0.3219752754296894559, 0.3333333333333333703, 0.3219752754296894559, 0.3333333333333333703, 0.3219752754296894559, 0.3333333333333333703, 0.3219752754296894559, 0.3333333333333333703, 0.3219752754296894559, 0.3333333333333333703, 0.3219752754296894559, 0.3333333333333333703, 0.3219752754296894559, 0.3333333333333333703, 0.3219752754296894559, 0.3333333333333333703, 0.3219752754296894559, 0.3333333333333333703, 0.3219752754296894559, 0.3333333333333333703, 0.3219752754296894559, 0.3333333333333333703, 0.3219752754296894559, 0.3333333333333333703, 0.3219752754296894559, 0.3333333333333333703, 0.3219752754296894559, 0.3333333333333333703, 0.3219752754296894559, 0.3333333333333333703, 0.3219752754296894559, 0.3333333333333333703, 0.3219752754296894559, 0.3333333333333333703, 0.3219752754296894559, 0.3333333333333333703, 0.3219752754296894559, 0.3333333333333333703, 0.3219752754296894559, 0.3333333333333333703, 0.3219752754296894559, 0.3333333333333333703, 0.3219752754296894559, 0.3333333333333333703, 0.3219752754296894559, 0.3333333333333333703, 0.3219752754296894559, 0.3333333333333333703, 0.3219752754296894559, 0.3333333333333333703, 0.3219752754296894559, 0.3333333333333333703, 0.3219752754296894559, 0.3333333333333333703, 0.3219752754296894559, 0.3333333333333333703, 0.3219752754296894559, 0.3333333333333333703, 0.3219752754296894559, 0.3333333333333333703, 0.3219752754296894559, 0.3333333333333333703, 0.3219752754296894559, 0.3333333333333333703, 0.3219752754296894559, 0.3333333333333333703, 0.3219752754296894559, 0.3333333333333333703, 0.3219752754296894559, 0.3333333333333333703, 0.3219752754296894559, 0.3333333333333333703, 0.3219752754296894559, 0.3333333333333333703, 0.3219752754296894559, 0.3333333333333333703, 0.3219752754296894559, 0.3333333333333333703, 0.3219752754296894559, 0.3333333333333333703, 0.3219752754296894559, 0.3333333333333333703, 0.3219752754296894559, 0.3333333333333333703, 0.3219752754296894559, 0.3333333333333333703, 0.3219752754296894559, 0.3333333333333333703, 0.3219752754296894559, 0.3333333333333333703, 0.3219752754296894559, 0.3333333333333333703, 0.3219752754296894559, 0.3333333333333333703, 0.3219752754296894559, 0.3333333333333333703, 0.3219752754296894559, 0.3333333333333333703, 0.3219752754296894559, 0.3333333333333333703, 0.3219752754296894559, 0.3333333333333333703, 0.3219752754296894559, 0.3333333333333333703, 0.3219752754296894559, 0.3333333333333333703, 0.3219752754296894559, 0.3333333333333333703, 0.3219752754296894559, 0.3333333333333333703, 0.3219752754296894559, 0.3333333333333333703),
 ( 1.000000000000000000, 0.9659258262890683122, 1.000000000000000000, 0.9659258262890683122, 1.000000000000000000, 0.9659258262890683122, 1.000000000000000000, 0.9659258262890683122, 1.000000000000000000, 0.9659258262890683122, 1.000000000000000000, 0.9659258262890683122, 1.000000000000000000, 0.9659258262890683122, 1.000000000000000000, 0.9659258262890683122, 1.000000000000000000, 0.9659258262890683122, 1.000000000000000000, 0.9659258262890683122, 1.000000000000000000, 0.9659258262890683122, 1.000000000000000000, 0.9659258262890683122, 1.000000000000000000, 0.9659258262890683122, 1.000000000000000000, 0.9659258262890683122, 1.000000000000000000, 0.9659258262890683122, 1.000000000000000000, 0.9659258262890683122, 1.000000000000000000, 0.9659258262890683122, 1.000000000000000000, 0.9659258262890683122, 1.000000000000000000, 0.9659258262890683122, 1.000000000000000000, 0.9659258262890683122, 1.000000000000000000, 0.9659258262890683122, 1.000000000000000000, 0.9659258262890683122, 1.000000000000000000, 0.9659258262890683122, 1.000000000000000000, 0.9659258262890683122, 1.000000000000000000, 0.9659258262890683122, 1.000000000000000000, 0.9659258262890683122, 1.000000000000000000, 0.9659258262890683122, 1.000000000000000000, 0.9659258262890683122, 1.000000000000000000, 0.9659258262890683122, 1.000000000000000000, 0.9659258262890683122, 1.000000000000000000, 0.9659258262890683122, 1.000000000000000000, 0.9659258262890683122, 1.000000000000000000, 0.9659258262890683122, 1.000000000000000000, 0.9659258262890683122, 1.000000000000000000, 0.9659258262890683122, 1.000000000000000000, 0.9659258262890683122, 1.000000000000000000, 0.9659258262890683122, 1.000000000000000000, 0.9659258262890683122, 1.000000000000000000, 0.9659258262890683122, 1.000000000000000000, 0.9659258262890683122, 1.000000000000000000, 0.9659258262890683122, 1.000000000000000000, 0.9659258262890683122, 1.000000000000000000, 0.9659258262890683122, 1.000000000000000000, 0.9659258262890683122, 1.000000000000000000, 0.9659258262890683122, 1.000000000000000000, 0.9659258262890683122, 1.000000000000000000, 0.9659258262890683122, 1.000000000000000000, 0.9659258262890683122, 1.000000000000000000, 0.9659258262890683122, 1.000000000000000000, 0.9659258262890683122, 1.000000000000000000, 0.9659258262890683122, 1.000000000000000000, 0.9659258262890683122, 1.000000000000000000, 0.9659258262890683122, 1.000000000000000000, 0.9659258262890683122, 1.000000000000000000, 0.9659258262890683122, 1.000000000000000000, 0.9659258262890683122, 1.000000000000000000, 0.9659258262890683122, 1.000000000000000000, 0.9659258262890683122, 1.000000000000000000, 0.9659258262890683122, 1.000000000000000000, 0.9659258262890683122, 1.000000000000000000, 0.9659258262890683122, 1.000000000000000000, 0.9659258262890683122, 1.000000000000000000, 0.9659258262890683122, 1.000000000000000000, 0.9659258262890683122, 1.000000000000000000, 0.9659258262890683122, 1.000000000000000000, 0.9659258262890683122, 1.000000000000000000, 0.9659258262890683122, 1.000000000000000000, 0.9659258262890683122, 1.000000000000000000, 0.9659258262890683122, 1.000000000000000000, 0.9659258262890683122, 1.000000000000000000, 0.9659258262890683122, 1.000000000000000000, 0.9659258262890683122, 1.000000000000000000, 0.9659258262890683122, 1.000000000000000000, 0.9659258262890683122, 1.000000000000000000, 0.9659258262890683122, 1.000000000000000000, 0.9659258262890683122, 1.000000000000000000, 0.9659258262890683122, 1.000000000000000000, 0.9659258262890683122, 1.000000000000000000, 0.9659258262890683122, 1.000000000000000000, 0.9659258262890683122, 1.000000000000000000, 0.9659258262890683122, 1.000000000000000000, 0.9659258262890683122, 1.000000000000000000, 0.9659258262890683122, 1.000000000000000000, 0.9659258262890683122, 1.000000000000000000, 0.9659258262890683122, 1.000000000000000000, 0.9659258262890683122, 1.000000000000000000, 0.9659258262890683122, 1.000000000000000000, 0.9659258262890683122, 1.000000000000000000, 0.9659258262890683122, 1.000000000000000000, 0.9659258262890683122, 1.000000000000000000, 0.9659258262890683122, 1.000000000000000000, 0.9659258262890683122, 1.000000000000000000, 0.9659258262890683122, 1.000000000000000000, 0.9659258262890683122, 1.000000000000000000, 0.9659258262890683122, 1.000000000000000000, 0.9659258262890683122, 1.000000000000000000) ) ) 
 REPRESENTATION_ITEM ( '' )  SURFACE ( )  );
#14821=CARTESIAN_POINT ( 'NONE',  ( -34.16294563604515133, 214.6737587650350747, -4.842901733360249317 ) ) ;
#14825=CARTESIAN_POINT ( 'NONE',  ( -57.71502896937850835, 213.8393509191290889, -2.350049139982142155 ) ) ;
#14832=CARTESIAN_POINT ( 'NONE',  ( -58.31622103062156981, 212.1620413398628671, 8.530955311639223382 ) ) ;
#14837=CARTESIAN_POINT ( 'NONE',  ( -43.67038769728823411, 208.1428034533959703, 6.469044688360771289 ) ) ;
#14849=CARTESIAN_POINT ( 'NONE',  ( -52.77455436395490551, 205.1570982666397356, 4.673758765035198159 ) ) ;
#14864=CARTESIAN_POINT ( 'NONE',  ( -56.52752896937850124, 213.3500491399821613, 5.571401726697954970 ) ) ;
#14866=CARTESIAN_POINT ( 'NONE',  ( -67.80877896937850835, 211.6261429550004607, -6.530955311639245586 ) ) ;
#14869=CARTESIAN_POINT ( 'NONE',  ( -62.86830436395490551, 209.8844732041982297, 4.499999999999996447 ) ) ;
#14870=CARTESIAN_POINT ( 'NONE',  ( -35.95163769728824121, 217.4189793300686233, -4.149950860017907139 ) ) ;
#14873=CARTESIAN_POINT ( 'NONE',  ( -55.93377896937850124, 207.8379586601372750, 8.530955311639258909 ) ) ;
#14886=CARTESIAN_POINT ( 'NONE',  ( -56.33705436395489841, 205.3262412349647263, -4.842901733360204020 ) ) ;
#14911=CARTESIAN_POINT ( 'NONE',  ( -33.57663769728823411, 206.0451222850691408, 2.149950860017832532 ) ) ;
#14915=CARTESIAN_POINT ( 'NONE',  ( -64.05580436395490551, 216.5000000000000000, 0.1155267958017343610 ) ) ;
#14917=CARTESIAN_POINT ( 'NONE',  ( -33.17336230271183695, 217.4189793300686233, 4.149950860017807663 ) ) ;
#14922=CARTESIAN_POINT ( 'NONE',  ( -64.24627896937849414, 203.4690446883607535, -1.626142955000504209 ) ) ;
#14931=CARTESIAN_POINT ( 'NONE',  ( -64.64955436395490551, 214.8429017333601792, -4.673758765035197271 ) ) ;
#14969=CARTESIAN_POINT ( 'NONE',  ( -32.58705436395489841, 205.3262412349647263, -4.842901733360204020 ) ) ;
#14986=PLANE ( 'NONE',  #2153 ) ;
#15003=CARTESIAN_POINT ( 'NONE',  ( -30.20461230271182274, 208.1428034533959135, -6.469044688360754414 ) ) ;
#15007=CARTESIAN_POINT ( 'NONE',  ( -58.50669563604516554, 209.8844732041982297, -4.499999999999996447 ) ) ;
#15008=CARTESIAN_POINT ( 'NONE',  ( -36.14955436395490551, 214.8429017333601792, -4.673758765035196383 ) ) ;
#15013=CARTESIAN_POINT ( 'NONE',  ( -62.07663769728824121, 202.5810206699313767, 4.149950860017909804 ) ) ;
#15036=CARTESIAN_POINT ( 'NONE',  ( -51.38913769728823411, 206.8500491399821044, -5.686928522499717253 ) ) ;
#15050=CARTESIAN_POINT ( 'NONE',  ( -45.04836230271183695, 204.3130714775002446, -3.149950860017828091 ) ) ;
#15053=CARTESIAN_POINT ( 'NONE',  ( -34.95461230271183695, 208.6787018382582346, -4.469044688360757966 ) ) ;
#15056=CARTESIAN_POINT ( 'NONE',  ( -61.08705436395490551, 206.7903428501026042, -3.378800118222489157 ) ) ;
#15058=CARTESIAN_POINT ( 'NONE',  ( -33.97247103062156270, 205.6499508600178956, 7.303452534266880569 ) ) ;
#15062=CARTESIAN_POINT ( 'NONE',  ( -55.53794563604517975, 203.8621396198271043, 6.307003348498029460 ) ) ;
#15072=CARTESIAN_POINT ( 'NONE',  ( -48.22247103062156270, 206.6499508600178672, 5.571401726697986057 ) ) ;
#15099=CARTESIAN_POINT ( 'NONE',  ( -36.14955436395489841, 213.3788001182225003, -3.209657149897400252 ) ) ;
#15103=CARTESIAN_POINT ( 'NONE',  ( -56.13913769728823411, 206.8500491399821044, -5.686928522499717253 ) ) ;
#15104=CARTESIAN_POINT ( 'NONE',  ( -66.23288769728823411, 201.5309553116392181, -2.393094931466246855 ) ) ;
#15109=CARTESIAN_POINT ( 'NONE',  ( -62.26711230271183695, 216.4690446883607535, -1.857196546604089393 ) ) ;
#15116=CARTESIAN_POINT ( 'NONE',  ( -66.82663769728823411, 204.3130714775002730, 3.149950860017883603 ) ) ;
#15156=CARTESIAN_POINT ( 'NONE',  ( -65.24330436395489130, 210.1155267958017703, -4.499999999999996447 ) ) ;
#15196=CARTESIAN_POINT ( 'NONE',  ( -63.25669563604515844, 209.8844732041981729, -8.500000000000003553 ) ) ;
#15200=CARTESIAN_POINT ( 'NONE',  ( -40.69419563604516554, 205.4999999999999716, 0.1155267958017633378 ) ) ;
#15206=CARTESIAN_POINT ( 'NONE',  ( -66.43080436395490551, 201.5000000000000000, -0.1155267958017054536 ) ) ;
#15213=CARTESIAN_POINT ( 'NONE',  ( -33.57663769728823411, 204.3130714775002730, 3.149950860017883603 ) ) ;
#15240=CARTESIAN_POINT ( 'NONE',  ( -40.10044563604516554, 205.1570982666397072, -4.673758765035155527 ) ) ;
#15242=CARTESIAN_POINT ( 'NONE',  ( -30.79836230271183339, 206.0451222850691977, -2.149950860017851184 ) ) ;
#15245=CARTESIAN_POINT ( 'NONE',  ( -60.29538769728823411, 211.3212981617418222, -4.469044688360751749 ) ) ;
#15246=CARTESIAN_POINT ( 'NONE',  ( -34.36830436395490551, 209.8844732041983150, 8.500000000000003553 ) ) ;
#15250=CARTESIAN_POINT ( 'NONE',  ( -57.71502896937850835, 217.3034525342667962, -4.350049139982195001 ) ) ;
#15260=CARTESIAN_POINT ( 'NONE',  ( -35.15997103062156270, 215.5714017266979852, 3.350049139982118618 ) ) ;
#15288=CARTESIAN_POINT ( 'NONE',  ( -33.37872103062156981, 205.4690446883607535, 1.090244570138264368 ) ) ;
#15293=CARTESIAN_POINT ( 'NONE',  ( -58.90997103062156270, 215.5714017266979852, 3.350049139982118618 ) ) ;
#15294=CARTESIAN_POINT ( 'NONE',  ( -33.96502896937850124, 217.3034525342667962, -4.350049139982195001 ) ) ;
#15299=CARTESIAN_POINT ( 'NONE',  ( -57.12127896937847993, 216.5309553116391612, 1.626142955000506873 ) ) ;
#15307=CARTESIAN_POINT ( 'NONE',  ( -68.60788769728824832, 216.4690446883607535, 1.857196546604031662 ) ) ;
#15346=CARTESIAN_POINT ( 'NONE',  ( -67.81622103062157692, 211.0902445701382533, 4.530955311639240257 ) ) ;
#15387=CARTESIAN_POINT ( 'NONE',  ( -59.49627896937850835, 201.4690446883607251, -2.162041339862721845 ) ) ;
#15391=CARTESIAN_POINT ( 'NONE',  ( -41.28794563604517265, 206.7903428501025758, 3.378800118222471838 ) ) ;
#15398=CARTESIAN_POINT ( 'NONE',  ( -47.23288769728824121, 201.5309553116392181, -2.393094931466246855 ) ) ;
#15431=CARTESIAN_POINT ( 'NONE',  ( -31.59002896937850124, 204.4285982733020433, 3.350049139982171020 ) ) ;
#15433=CARTESIAN_POINT ( 'NONE',  ( -61.67336230271183695, 215.6869285224997270, 3.149950860017831200 ) ) ;
#15436=CARTESIAN_POINT ( 'NONE',  ( -45.05580436395490551, 214.5000000000000284, 0.1155267958017899832 ) ) ;
#15437=CARTESIAN_POINT ( 'NONE',  ( -69.20163769728823411, 215.6869285224996986, -3.149950860017881382 ) ) ;
#15439=CARTESIAN_POINT ( 'NONE',  ( -68.00669563604516554, 209.8844732041982013, -6.500000000000000888 ) ) ;
#15441=CARTESIAN_POINT ( 'NONE',  ( -49.99627896937850835, 201.4690446883607251, -2.162041339862721845 ) ) ;
#15452=CARTESIAN_POINT ( 'NONE',  ( -37.53497103062156981, 204.4285982733020148, -3.350049139982115509 ) ) ;
#15478=CARTESIAN_POINT ( 'NONE',  ( -67.21502896937850835, 213.8393509191290889, -2.350049139982142155 ) ) ;
#15482=CARTESIAN_POINT ( 'NONE',  ( -50.99330436395489841, 210.1155267958017134, -6.500000000000000888 ) ) ;
#15483=CARTESIAN_POINT ( 'NONE',  ( -35.54836230271182984, 202.5810206699313767, -4.149950860017804111 ) ) ;
#15489=CARTESIAN_POINT ( 'NONE',  ( -59.10044563604516554, 205.1570982666397072, -4.673758765035155527 ) ) ;
#15496=CARTESIAN_POINT ( 'NONE',  ( -65.83705436395489130, 205.3262412349647548, -4.842901733360204908 ) ) ;
#15501=CARTESIAN_POINT ( 'NONE',  ( -34.76413769728823411, 214.1499508600179240, 7.418979330068584233 ) ) ;
#15569=ORIENTED_EDGE ( 'NONE', *, *, #19616, .F. ) ;
#15573=CARTESIAN_POINT ( 'NONE',  ( -57.71502896937850835, 217.3034525342667962, -4.350049139982195001 ) ) ;
#15578=CARTESIAN_POINT ( 'NONE',  ( -44.45461230271183695, 208.6787018382582346, -4.469044688360757966 ) ) ;
#15584=CARTESIAN_POINT ( 'NONE',  ( -47.43080436395489841, 201.5000000000000000, -0.1155267958017054536 ) ) ;
#15615=CARTESIAN_POINT ( 'NONE',  ( -42.47544563604516554, 214.8429017333602360, 4.673758765035156415 ) ) ;
#15616=CARTESIAN_POINT ( 'NONE',  ( -59.10044563604516554, 205.1570982666397072, -4.673758765035155527 ) ) ;
#15620=CARTESIAN_POINT ( 'NONE',  ( -46.04538769728823411, 211.3212981617418222, -4.469044688360751749 ) ) ;
#15621=CARTESIAN_POINT ( 'NONE',  ( -37.33705436395491262, 203.8621396198270475, -6.307003348497942419 ) ) ;
#15626=CARTESIAN_POINT ( 'NONE',  ( -46.43377896937850835, 207.8379586601372750, 8.530955311639258909 ) ) ;
#15640=CARTESIAN_POINT ( 'NONE',  ( -38.72247103062156981, 206.6499508600178672, 5.571401726697986057 ) ) ;
#15668=CARTESIAN_POINT ( 'NONE',  ( -50.98586230271183695, 207.8500491399821613, 3.954877714930852495 ) ) ;
#15673=CARTESIAN_POINT ( 'NONE',  ( -45.45163769728822700, 215.6869285224996986, -3.149950860017881382 ) ) ;
#15674=CARTESIAN_POINT ( 'NONE',  ( -64.25372103062157692, 218.5309553116391896, -2.162041339862839084 ) ) ;
#15679=CARTESIAN_POINT ( 'NONE',  ( -42.07961230271182984, 211.8571965466040297, 6.469044688360755302 ) ) ;
#15687=CARTESIAN_POINT ( 'NONE',  ( -49.80580436395490551, 216.5000000000000000, 0.1155267958017343610 ) ) ;
#15692=CARTESIAN_POINT ( 'NONE',  ( -37.73288769728823411, 201.5309553116392181, -2.393094931466246855 ) ) ;
#15766=CARTESIAN_POINT ( 'NONE',  ( -54.35044563604515844, 203.6929966515019430, -6.137860380172892150 ) ) ;
#15770=CARTESIAN_POINT ( 'NONE',  ( -46.43377896937850835, 208.9097554298617183, 4.530955311639234040 ) ) ;
#15777=CARTESIAN_POINT ( 'NONE',  ( -49.01413769728823411, 214.1499508600179240, 7.418979330068584233 ) ) ;
#15784=CARTESIAN_POINT ( 'NONE',  ( -35.35788769728823411, 216.4690446883607535, 1.857196546604031662 ) ) ;
#15805=CARTESIAN_POINT ( 'NONE',  ( -35.74627896937850124, 203.4690446883607535, -1.626142955000504209 ) ) ;
#15806=CARTESIAN_POINT ( 'NONE',  ( -50.19419563604517265, 203.5000000000000000, 0.1155267958017914542 ) ) ;
#15810=CARTESIAN_POINT ( 'NONE',  ( -49.80580436395490551, 214.5000000000000284, 0.1155267958017899832 ) ) ;
#15812=CARTESIAN_POINT ( 'NONE',  ( -60.88913769728823411, 206.8500491399821044, -5.686928522499717253 ) ) ;
#15815=CARTESIAN_POINT ( 'NONE',  ( -49.79836230271183695, 202.5810206699313767, -4.149950860017804111 ) ) ;
#15826=CARTESIAN_POINT ( 'NONE',  ( -34.76413769728823411, 213.1499508600178672, 5.686928522499718142 ) ) ;
#15856=CARTESIAN_POINT ( 'NONE',  ( -54.15252896937849414, 207.6499508600178387, -3.839350919129087547 ) ) ;
#15861=CARTESIAN_POINT ( 'NONE',  ( -42.08705436395489841, 205.3262412349647263, -4.842901733360204020 ) ) ;
#15862=CARTESIAN_POINT ( 'NONE',  ( -58.90997103062156981, 217.3034525342668815, 4.350049139982096413 ) ) ;
#15865=SHAPE_DEFINITION_REPRESENTATION ( #26507, #6520 ) ;
#15869=CARTESIAN_POINT ( 'NONE',  ( -39.90252896937850124, 206.6499508600178387, -5.571401726697954970 ) ) ;
#15877=CARTESIAN_POINT ( 'NONE',  ( -59.10788769728823411, 216.4690446883607535, 1.857196546604031662 ) ) ;
#15881=CARTESIAN_POINT ( 'NONE',  ( -39.11830436395489841, 209.8844732041983150, 8.500000000000003553 ) ) ;
#15891=CARTESIAN_POINT ( 'NONE',  ( -61.28497103062156981, 204.4285982733020148, -3.350049139982115509 ) ) ;
#15906=CARTESIAN_POINT ( 'NONE',  ( -62.86830436395490551, 209.8844732041982297, 4.499999999999996447 ) ) ;
#15916=EDGE_CURVE ( 'NONE', #29947, #14550, #71, .T. ) ;
#15954=CARTESIAN_POINT ( 'NONE',  ( -60.88169563604516554, 210.1155267958018271, 8.500000000000003553 ) ) ;
#15957=CARTESIAN_POINT ( 'NONE',  ( -47.81919563604517265, 214.5000000000000284, -0.1155267958017627827 ) ) ;
#15964=CARTESIAN_POINT ( 'NONE',  ( -49.21205436395490551, 216.1378603801730094, 6.307003348497944195 ) ) ;
#15997=CARTESIAN_POINT ( 'NONE',  ( -37.72544563604516554, 214.8429017333602360, 4.673758765035156415 ) ) ;
#15998=CARTESIAN_POINT ( 'NONE',  ( -60.88169563604516554, 210.1155267958017703, 6.500000000000000888 ) ) ;
#16002=CARTESIAN_POINT ( 'NONE',  ( -43.67038769728823411, 208.6787018382581778, 4.469044688360752637 ) ) ;
#16004=CARTESIAN_POINT ( 'NONE',  ( -59.89955436395490551, 214.8429017333601792, -4.673758765035196383 ) ) ;
#16008=CARTESIAN_POINT ( 'NONE',  ( -45.44419563604516554, 201.5000000000000000, 0.1155267958018195706 ) ) ;
#16019=CARTESIAN_POINT ( 'NONE',  ( -37.13913769728823411, 206.8500491399821044, -5.686928522499717253 ) ) ;
#16046=CARTESIAN_POINT ( 'NONE',  ( -54.94419563604517265, 205.4999999999999716, 0.1155267958017633378 ) ) ;
#16047=CARTESIAN_POINT ( 'NONE',  ( 0.000000000000000000, 0.000000000000000000, 0.000000000000000000 ) ) ;
#16050=CARTESIAN_POINT ( 'NONE',  ( -46.83705436395489841, 205.3262412349647263, -4.842901733360204020 ) ) ;
#16051=CARTESIAN_POINT ( 'NONE',  ( -51.98288769728823411, 201.5309553116392181, -2.393094931466246855 ) ) ;
#16056=CARTESIAN_POINT ( 'NONE',  ( -51.18377896937847993, 208.3738570449995109, 6.530955311639247363 ) ) ;
#16065=CARTESIAN_POINT ( 'NONE',  ( -53.56622103062156981, 211.6261429550005744, 6.530955311639228711 ) ) ;
#16069=CARTESIAN_POINT ( 'NONE',  ( -38.12872103062156270, 201.4690446883607819, 2.162041339862843525 ) ) ;
#16092=CARTESIAN_POINT ( 'NONE',  ( -50.79538769728824121, 211.3212981617418222, -4.469044688360751749 ) ) ;
#16114=VERTEX_POINT ( 'NONE', #34348 ) ;
#16140=CARTESIAN_POINT ( 'NONE',  ( -54.54836230271183695, 202.5810206699313767, -4.149950860017804111 ) ) ;
#16144=CARTESIAN_POINT ( 'NONE',  ( -34.75669563604515844, 209.8844732041982297, -4.499999999999996447 ) ) ;
#16182=CARTESIAN_POINT ( 'NONE',  ( -49.79836230271183695, 204.3130714775002446, -3.149950860017828091 ) ) ;
#16186=CARTESIAN_POINT ( 'NONE',  ( -49.21205436395490551, 213.2096571498974242, 3.378800118222489601 ) ) ;
#16187=CARTESIAN_POINT ( 'NONE',  ( -58.71205436395488420, 214.6737587650352168, 4.842901733360204908 ) ) ;
#16192=CARTESIAN_POINT ( 'NONE',  ( -49.20461230271185116, 207.6069050685336492, -8.469044688360751749 ) ) ;
#16229=CARTESIAN_POINT ( 'NONE',  ( -61.27752896937850124, 213.3500491399821613, 5.571401726697954970 ) ) ;
#16231=CARTESIAN_POINT ( 'NONE',  ( -58.11086230271183695, 212.1499508600178387, -3.954877714930852495 ) ) ;
#16236=CARTESIAN_POINT ( 'NONE',  ( -50.20163769728823411, 215.6869285224996986, -3.149950860017881382 ) ) ;
#16237=CARTESIAN_POINT ( 'NONE',  ( -56.33705436395490551, 203.8621396198270475, -6.307003348497942419 ) ) ;
#16243=CARTESIAN_POINT ( 'NONE',  ( -42.87127896937850124, 216.5309553116391612, 1.626142955000506873 ) ) ;
#16251=CARTESIAN_POINT ( 'NONE',  ( -53.96205436395489130, 214.6737587650351884, 4.842901733360205796 ) ) ;
#16255=CARTESIAN_POINT ( 'NONE',  ( -62.86830436395490551, 209.8844732041982581, 6.500000000000000888 ) ) ;
#16280=CARTESIAN_POINT ( 'NONE',  ( -59.30580436395490551, 214.5000000000000284, 0.1155267958017899832 ) ) ;
#16325=CARTESIAN_POINT ( 'NONE',  ( -45.84002896937850124, 202.6965474657332038, 4.350049139982197666 ) ) ;
#16328=CARTESIAN_POINT ( 'NONE',  ( -37.13169563604516554, 210.1155267958017703, 4.499999999999996447 ) ) ;
#16364=CARTESIAN_POINT ( 'NONE',  ( -31.39211230271182629, 203.5309553116391896, 1.857196546604092724 ) ) ;
#16366=CARTESIAN_POINT ( 'NONE',  ( -54.15252896937850124, 206.6499508600178387, -5.571401726697954970 ) ) ;
#16371=CARTESIAN_POINT ( 'NONE',  ( -38.32663769728823411, 206.0451222850691408, 2.149950860017832532 ) ) ;
#16372=CARTESIAN_POINT ( 'NONE',  ( -54.15997103062156981, 215.5714017266979852, 3.350049139982118618 ) ) ;
#16376=CARTESIAN_POINT ( 'NONE',  ( -30.00669563604516554, 209.8844732041981729, -8.500000000000003553 ) ) ;
#16414=CARTESIAN_POINT ( 'NONE',  ( -65.43377896937850835, 208.3738570449995109, 6.530955311639247363 ) ) ;
#16416=CARTESIAN_POINT ( 'NONE',  ( -52.96502896937850124, 213.8393509191290889, -2.350049139982142155 ) ) ;
#16421=CARTESIAN_POINT ( 'NONE',  ( -39.51413769728823411, 213.1499508600178672, 5.686928522499718142 ) ) ;
#16422=CARTESIAN_POINT ( 'NONE',  ( -62.07663769728824121, 202.5810206699313767, 4.149950860017909804 ) ) ;
#16427=CARTESIAN_POINT ( 'NONE',  ( -41.28794563604515133, 205.3262412349647832, 4.842901733360250205 ) ) ;
#16435=CARTESIAN_POINT ( 'NONE',  ( -55.94122103062156981, 208.3738570449994256, -6.530955311639227823 ) ) ;
#16441=CARTESIAN_POINT ( 'NONE',  ( -62.27455436395490551, 205.1570982666397356, 4.673758765035198159 ) ) ;
#16466=CARTESIAN_POINT ( 'NONE',  ( -56.93080436395490551, 205.4999999999999716, -0.1155267958017894420 ) ) ;
#16469=CARTESIAN_POINT ( 'NONE',  ( -66.82663769728823411, 204.3130714775002730, 3.149950860017883603 ) ) ;
#16512=CARTESIAN_POINT ( 'NONE',  ( -41.88169563604517265, 210.1155267958018271, 8.500000000000003553 ) ) ;
#16515=CARTESIAN_POINT ( 'NONE',  ( -66.22544563604516554, 214.8429017333602360, 4.673758765035156415 ) ) ;
#16518=CARTESIAN_POINT ( 'NONE',  ( -39.90997103062156270, 215.5714017266979852, 3.350049139982118618 ) ) ;
#16553=CARTESIAN_POINT ( 'NONE',  ( -46.23586230271182984, 206.8500491399821328, 5.686928522499748340 ) ) ;
#16557=CARTESIAN_POINT ( 'NONE',  ( -39.31622103062156981, 211.0902445701382533, 4.530955311639240257 ) ) ;
#16558=CARTESIAN_POINT ( 'NONE',  ( -51.19122103062155560, 208.3738570449993404, -6.530955311639226935 ) ) ;
#16563=CARTESIAN_POINT ( 'NONE',  ( -68.60788769728823411, 218.4690446883607535, 2.393094931466250408 ) ) ;
#16583=CARTESIAN_POINT ( 'NONE',  ( -64.45163769728823411, 215.6869285224996986, -3.149950860017881382 ) ) ;
#16602=CARTESIAN_POINT ( 'NONE',  ( -63.45461230271182274, 208.1428034533958851, -6.469044688360754414 ) ) ;
#16604=CARTESIAN_POINT ( 'NONE',  ( -46.43377896937850835, 208.9097554298617183, 4.530955311639234040 ) ) ;
#16608=CARTESIAN_POINT ( 'NONE',  ( -37.13913769728823411, 206.8500491399821044, -5.686928522499717253 ) ) ;
#16609=CARTESIAN_POINT ( 'NONE',  ( -55.74330436395489841, 210.1155267958016850, -8.500000000000003553 ) ) ;
#16614=CARTESIAN_POINT ( 'NONE',  ( -65.82961230271185116, 212.3930949314663792, 8.469044688360751749 ) ) ;
#16624=CARTESIAN_POINT ( 'NONE',  ( -41.69122103062156270, 208.3738570449994256, -6.530955311639227823 ) ) ;
#16629=CARTESIAN_POINT ( 'NONE',  ( -56.93080436395490551, 203.5000000000000000, -0.1155267958017335561 ) ) ;
#16653=CARTESIAN_POINT ( 'NONE',  ( -60.88913769728824121, 207.8500491399821613, -3.954877714930864485 ) ) ;
#16699=CARTESIAN_POINT ( 'NONE',  ( -41.68377896937850124, 207.8379586601372750, 8.530955311639258909 ) ) ;
#16703=CARTESIAN_POINT ( 'NONE',  ( -66.81919563604517975, 216.5000000000000000, -0.1155267958017906493 ) ) ;
#16707=CARTESIAN_POINT ( 'NONE',  ( -46.63913769728824121, 206.8500491399821044, -5.686928522499717253 ) ) ;
#16736=CARTESIAN_POINT ( 'NONE',  ( -39.70461230271183695, 208.1428034533959135, -6.469044688360754414 ) ) ;
#16740=CARTESIAN_POINT ( 'NONE',  ( -34.56622103062156981, 211.0902445701382533, 4.530955311639240257 ) ) ;
#16741=CARTESIAN_POINT ( 'NONE',  ( -49.40997103062156981, 215.5714017266979852, 3.350049139982118618 ) ) ;
#16746=CARTESIAN_POINT ( 'NONE',  ( -31.59002896937850124, 202.6965474657332038, 4.350049139982197666 ) ) ;
#16764=CARTESIAN_POINT ( 'NONE',  ( -68.60788769728823411, 216.4690446883607535, 1.857196546604031662 ) ) ;
#16783=CARTESIAN_POINT ( 'NONE',  ( -57.91294563604515844, 214.6737587650350747, -4.842901733360248429 ) ) ;
#16786=CARTESIAN_POINT ( 'NONE',  ( -41.48586230271182984, 207.8500491399821613, 3.954877714930852495 ) ) ;
#16790=CARTESIAN_POINT ( 'NONE',  ( -36.74330436395489841, 210.1155267958017134, -6.500000000000000888 ) ) ;
#16791=CARTESIAN_POINT ( 'NONE',  ( -47.23288769728824121, 201.5309553116392181, -2.393094931466246855 ) ) ;
#16796=CARTESIAN_POINT ( 'NONE',  ( -64.84002896937849414, 202.6965474657332038, 4.350049139982197666 ) ) ;
#16811=CARTESIAN_POINT ( 'NONE',  ( -61.28497103062156981, 204.4285982733020148, -3.350049139982115509 ) ) ;
#16838=CARTESIAN_POINT ( 'NONE',  ( -41.69122103062156270, 208.9097554298617752, -4.530955311639240257 ) ) ;
#16843=CARTESIAN_POINT ( 'NONE',  ( -67.22247103062156270, 206.6499508600178672, 5.571401726697986057 ) ) ;
#16885=CARTESIAN_POINT ( 'NONE',  ( -40.69419563604516554, 201.5000000000000000, 0.1155267958018195706 ) ) ;
#16888=CARTESIAN_POINT ( 'NONE',  ( -33.96502896937850124, 213.8393509191290889, -2.350049139982142155 ) ) ;
#16891=CARTESIAN_POINT ( 'NONE',  ( -46.24330436395489841, 210.1155267958017134, -6.500000000000000888 ) ) ;
#16923=CARTESIAN_POINT ( 'NONE',  ( -39.90252896937850124, 206.6499508600178387, -5.571401726697954970 ) ) ;
#16926=CARTESIAN_POINT ( 'NONE',  ( -35.35788769728823411, 214.4690446883608104, 1.321298161741840893 ) ) ;
#16927=CARTESIAN_POINT ( 'NONE',  ( -45.05580436395489841, 216.5000000000000000, 0.1155267958017343610 ) ) ;
#16933=CARTESIAN_POINT ( 'NONE',  ( -68.40997103062156270, 217.3034525342668815, 4.350049139982096413 ) ) ;
#16940=DIRECTION ( 'NONE',  ( -0.9933043639548644332, 0.1155267958017622554, 0.000000000000000000 ) ) ;
#16943=CARTESIAN_POINT ( 'NONE',  ( -31.99330436395490196, 210.1155267958017134, -6.500000000000000888 ) ) ;
#16950=CARTESIAN_POINT ( 'NONE',  ( -66.23288769728823411, 203.5309553116391612, -1.857196546604028775 ) ) ;
#16967=CARTESIAN_POINT ( 'NONE',  ( -62.86086230271182984, 213.1499508600178387, -5.686928522499747451 ) ) ;
#16970=CARTESIAN_POINT ( 'NONE',  ( -37.72544563604516554, 213.3788001182224718, 3.209657149897419348 ) ) ;
#16973=CARTESIAN_POINT ( 'NONE',  ( -68.80580436395490551, 214.5000000000000284, 0.1155267958017899832 ) ) ;
#16974=CARTESIAN_POINT ( 'NONE',  ( -49.01413769728823411, 214.1499508600179240, 7.418979330068584233 ) ) ;
#16978=CARTESIAN_POINT ( 'NONE',  ( -38.71502896937850124, 215.5714017266979567, -3.350049139982168800 ) ) ;
#16992=CARTESIAN_POINT ( 'NONE',  ( -59.30580436395489841, 216.5000000000000000, 0.1155267958017343610 ) ) ;
#17018=CARTESIAN_POINT ( 'NONE',  ( -44.06622103062156270, 211.0902445701382533, 4.530955311639240257 ) ) ;
#17068=CARTESIAN_POINT ( 'NONE',  ( -55.93377896937850124, 208.3738570449995109, 6.530955311639247363 ) ) ;
#17072=CARTESIAN_POINT ( 'NONE',  ( -41.69122103062155560, 208.3738570449993404, -6.530955311639226935 ) ) ;
#17107=CARTESIAN_POINT ( 'NONE',  ( -41.68377896937849414, 208.3738570449995109, 6.530955311639247363 ) ) ;
#17112=CARTESIAN_POINT ( 'NONE',  ( -61.07961230271182984, 211.3212981617417938, 4.469044688360757966 ) ) ;
#17114=CARTESIAN_POINT ( 'NONE',  ( -46.83705436395489841, 205.3262412349647263, -4.842901733360204020 ) ) ;
#17120=CARTESIAN_POINT ( 'NONE',  ( -37.92336230271182984, 217.4189793300686233, 4.149950860017807663 ) ) ;
#17138=CARTESIAN_POINT ( 'NONE',  ( -62.86830436395490551, 209.8844732041982581, 6.500000000000000888 ) ) ;
#17156=CARTESIAN_POINT ( 'NONE',  ( -54.74627896937849414, 203.4690446883607535, -1.626142955000504209 ) ) ;
#17158=CARTESIAN_POINT ( 'NONE',  ( -42.27752896937850835, 212.3500491399821613, 3.839350919129088435 ) ) ;
#17163=CARTESIAN_POINT ( 'NONE',  ( -38.12872103062154849, 203.4690446883607535, 1.626142955000567936 ) ) ;
#17164=CARTESIAN_POINT ( 'NONE',  ( -43.07663769728824121, 202.5810206699313767, 4.149950860017909804 ) ) ;
#17168=CARTESIAN_POINT ( 'NONE',  ( -38.91294563604516554, 214.6737587650350747, -4.842901733360249317 ) ) ;
#17179=CARTESIAN_POINT ( 'NONE',  ( -52.77455436395490551, 205.1570982666397356, 4.673758765035198159 ) ) ;
#17204=CARTESIAN_POINT ( 'NONE',  ( -48.22247103062156981, 207.6499508600178387, 3.839350919129076445 ) ) ;
#17208=CARTESIAN_POINT ( 'NONE',  ( -69.99330436395490551, 210.1155267958017134, -6.500000000000000888 ) ) ;
#17215=AXIS2_PLACEMENT_3D ( 'NONE', #16047, #4651, #19645 ) ;
#17258=CARTESIAN_POINT ( 'NONE',  ( -41.49330436395490551, 210.1155267958017134, -6.500000000000000888 ) ) ;
#17293=CARTESIAN_POINT ( 'NONE',  ( -36.34002896937850124, 204.4285982733020433, 3.350049139982171020 ) ) ;
#17297=CARTESIAN_POINT ( 'NONE',  ( -52.76711230271184405, 214.4690446883608104, -1.321298161741814914 ) ) ;
#17298=CARTESIAN_POINT ( 'NONE',  ( -44.06622103062156981, 211.6261429550005744, 6.530955311639227823 ) ) ;
#17304=CARTESIAN_POINT ( 'NONE',  ( -63.26413769728823411, 214.1499508600179240, 7.418979330068584233 ) ) ;
#17310=CARTESIAN_POINT ( 'NONE',  ( -39.11830436395489841, 209.8844732041982581, 6.500000000000000888 ) ) ;
#17321=CARTESIAN_POINT ( 'NONE',  ( -50.79538769728821990, 211.8571965466039444, -6.469044688360768625 ) ) ;
#17341=CARTESIAN_POINT ( 'NONE',  ( -48.41294563604515844, 214.6737587650350747, -4.842901733360248429 ) ) ;
#17343=CARTESIAN_POINT ( 'NONE',  ( -37.32961230271184405, 211.3212981617417938, 4.469044688360757966 ) ) ;
#17347=CARTESIAN_POINT ( 'NONE',  ( -56.93080436395490551, 205.4999999999999716, -0.1155267958017894420 ) ) ;
#17348=CARTESIAN_POINT ( 'NONE',  ( -41.29538769728824121, 212.3930949314662371, -8.469044688360781947 ) ) ;
#17353=CARTESIAN_POINT ( 'NONE',  ( -30.40252896937849769, 206.6499508600178387, -5.571401726697954970 ) ) ;
#17365=CARTESIAN_POINT ( 'NONE',  ( -51.78497103062156981, 204.4285982733020148, -3.350049139982115509 ) ) ;
#17393=CARTESIAN_POINT ( 'NONE',  ( -49.21205436395490551, 213.2096571498974242, 3.378800118222489601 ) ) ;
#17398=CARTESIAN_POINT ( 'NONE',  ( -63.85788769728821279, 216.4690446883607535, 1.857196546604031662 ) ) ;
#17435=PRODUCT ( 'pusher spring', 'pusher spring', '', ( #17768 ) ) ;
#17444=CARTESIAN_POINT ( 'NONE',  ( -34.17038769728823411, 208.1428034533959703, 6.469044688360770401 ) ) ;
#17482=CARTESIAN_POINT ( 'NONE',  ( -66.81919563604516554, 218.5000000000000000, -0.1155267958018185298 ) ) ;
#17485=CARTESIAN_POINT ( 'NONE',  ( -57.12127896937850124, 214.5309553116392749, 1.090244570138288127 ) ) ;
#17486=CARTESIAN_POINT ( 'NONE',  ( -35.75372103062156981, 216.5309553116391612, -1.626142955000564383 ) ) ;
#17491=CARTESIAN_POINT ( 'NONE',  ( -58.51413769728822700, 214.1499508600179240, 7.418979330068584233 ) ) ;
#17496=CARTESIAN_POINT ( 'NONE',  ( -37.33705436395490551, 205.3262412349647548, -4.842901733360204908 ) ) ;
#17508=CARTESIAN_POINT ( 'NONE',  ( -56.33705436395489841, 205.3262412349647263, -4.842901733360204020 ) ) ;
#17527=CARTESIAN_POINT ( 'NONE',  ( -48.80877896937850835, 211.6261429550004891, -6.530955311639245586 ) ) ;
#17529=CARTESIAN_POINT ( 'NONE',  ( -30.60044563604516199, 206.6211998817775566, -3.209657149897419348 ) ) ;
#17533=CARTESIAN_POINT ( 'NONE',  ( -53.56622103062157692, 211.0902445701382533, 4.530955311639240257 ) ) ;
#17534=CARTESIAN_POINT ( 'NONE',  ( -48.42038769728824832, 207.6069050685337913, 8.469044688360781947 ) ) ;
#17539=CARTESIAN_POINT ( 'NONE',  ( -62.06919563604516554, 218.5000000000000000, -0.1155267958018185298 ) ) ;
#17551=CARTESIAN_POINT ( 'NONE',  ( -48.02455436395488420, 205.1570982666397356, 4.673758765035198159 ) ) ;
#17579=CARTESIAN_POINT ( 'NONE',  ( -38.32663769728823411, 206.0451222850691408, 2.149950860017832532 ) ) ;
#17583=CARTESIAN_POINT ( 'NONE',  ( -65.24330436395489130, 210.1155267958017134, -6.500000000000000888 ) ) ;
#17585=CARTESIAN_POINT ( 'NONE',  ( -38.12127896937850835, 218.5309553116392465, 2.162041339862725842 ) ) ;
#17635=CARTESIAN_POINT ( 'NONE',  ( -36.14955436395490551, 214.8429017333601792, -4.673758765035196383 ) ) ;
#17670=CARTESIAN_POINT ( 'NONE',  ( -67.61086230271183695, 214.1499508600178387, -7.418979330068641964 ) ) ;
#17673=CARTESIAN_POINT ( 'NONE',  ( -52.37127896937850835, 214.5309553116392749, 1.090244570138288127 ) ) ;
#17674=CARTESIAN_POINT ( 'NONE',  ( -32.38913769728823411, 206.8500491399821044, -5.686928522499717253 ) ) ;
#17679=CARTESIAN_POINT ( 'NONE',  ( -55.14955436395491262, 216.3070033484980002, -6.137860380172975638 ) ) ;
#17685=CARTESIAN_POINT ( 'NONE',  ( -49.01413769728823411, 213.1499508600178672, 5.686928522499718142 ) ) ;
#17696=CARTESIAN_POINT ( 'NONE',  ( -53.36830436395489841, 209.8844732041982581, 6.500000000000000888 ) ) ;
#17711=CARTESIAN_POINT ( 'NONE',  ( -49.99627896937850124, 203.4690446883607535, -1.626142955000504209 ) ) ;
#17713=CARTESIAN_POINT ( 'NONE',  ( -32.97544563604516554, 213.3788001182224718, 3.209657149897419348 ) ) ;
#17717=CARTESIAN_POINT ( 'NONE',  ( -63.46205436395489841, 213.2096571498974242, 3.378800118222489601 ) ) ;
#17718=CARTESIAN_POINT ( 'NONE',  ( -68.40997103062156270, 215.5714017266979852, 3.350049139982118618 ) ) ;
#17722=CARTESIAN_POINT ( 'NONE',  ( -59.69419563604517265, 201.5000000000000000, 0.1155267958018195706 ) ) ;
#17734=CARTESIAN_POINT ( 'NONE',  ( -43.86830436395490551, 209.8844732041982581, 6.500000000000000888 ) ) ;
#17762=CARTESIAN_POINT ( 'NONE',  ( -36.94122103062156981, 208.9097554298617752, -4.530955311639240257 ) ) ;
#17766=CARTESIAN_POINT ( 'NONE',  ( -54.55580436395489841, 216.5000000000000000, 0.1155267958017343610 ) ) ;
#17767=CARTESIAN_POINT ( 'NONE',  ( -32.97544563604516554, 216.3070033484980854, 6.137860380172893926 ) ) ;
#17768=PRODUCT_CONTEXT ( 'NONE', #35935, 'mechanical' ) ;
#17772=CARTESIAN_POINT ( 'NONE',  ( -53.36086230271183695, 213.1499508600178387, -5.686928522499747451 ) ) ;
#17780=CARTESIAN_POINT ( 'NONE',  ( -63.46205436395489841, 214.6737587650351884, 4.842901733360205796 ) ) ;
#17826=CARTESIAN_POINT ( 'NONE',  ( -63.06622103062156270, 211.0902445701382533, 4.530955311639240257 ) ) ;
#17859=CARTESIAN_POINT ( 'NONE',  ( -32.57961230271183695, 211.8571965466040297, 6.469044688360755302 ) ) ;
#17862=CARTESIAN_POINT ( 'NONE',  ( -60.28794563604517975, 206.7903428501025758, 3.378800118222471838 ) ) ;
#17863=CARTESIAN_POINT ( 'NONE',  ( -38.12872103062154849, 203.4690446883607535, 1.626142955000567936 ) ) ;
#17868=CARTESIAN_POINT ( 'NONE',  ( -58.90997103062156981, 217.3034525342668815, 4.350049139982096413 ) ) ;
#17873=CARTESIAN_POINT ( 'NONE',  ( -48.61830436395490551, 209.8844732041982581, 6.500000000000000888 ) ) ;
#17886=CARTESIAN_POINT ( 'NONE',  ( -57.12872103062157692, 203.4690446883607535, 1.626142955000567936 ) ) ;
#17901=CARTESIAN_POINT ( 'NONE',  ( -45.24627896937849414, 203.4690446883607535, -1.626142955000504209 ) ) ;
#17903=CARTESIAN_POINT ( 'NONE',  ( -31.98586230271182984, 207.8500491399821613, 3.954877714930852495 ) ) ;
#17907=CARTESIAN_POINT ( 'NONE',  ( -63.65997103062157692, 213.8393509191290889, 2.350049139982164359 ) ) ;
#17908=CARTESIAN_POINT ( 'NONE',  ( -64.84747103062156270, 213.3500491399821328, -5.571401726697985168 ) ) ;
#17911=CARTESIAN_POINT ( 'NONE',  ( -58.90252896937851546, 205.6499508600178103, -7.303452534266820173 ) ) ;
#17923=CARTESIAN_POINT ( 'NONE',  ( -55.14955436395487709, 214.8429017333601792, -4.673758765035196383 ) ) ;
#17952=CARTESIAN_POINT ( 'NONE',  ( -66.22544563604516554, 213.3788001182224718, 3.209657149897419348 ) ) ;
#17956=CARTESIAN_POINT ( 'NONE',  ( -57.12872103062157692, 203.4690446883607535, 1.626142955000567936 ) ) ;
#17957=CARTESIAN_POINT ( 'NONE',  ( -67.02455436395489130, 203.6929966515020283, 6.137860380172978303 ) ) ;
#17963=CARTESIAN_POINT ( 'NONE',  ( -60.88169563604516554, 210.1155267958017703, 6.500000000000000888 ) ) ;
#17984=PRODUCT_DEFINITION_CONTEXT ( 'detailed design', #29401, 'design' ) ;
#18009=CARTESIAN_POINT ( 'NONE',  ( -68.80580436395490551, 214.5000000000000284, 0.1155267958017899832 ) ) ;
#18048=CARTESIAN_POINT ( 'NONE',  ( -64.04836230271183695, 202.5810206699313767, -4.149950860017804111 ) ) ;
#18052=CARTESIAN_POINT ( 'NONE',  ( -50.59002896937850835, 206.1606490808709111, 2.350049139982143931 ) ) ;
#18057=CARTESIAN_POINT ( 'NONE',  ( -63.46205436395489841, 216.1378603801730094, 6.307003348497944195 ) ) ;
#18093=CARTESIAN_POINT ( 'NONE',  ( -33.76711230271184405, 216.4690446883607535, -1.857196546604089393 ) ) ;
#18096=CARTESIAN_POINT ( 'NONE',  ( -63.65252896937849414, 206.6499508600178387, -5.571401726697954970 ) ) ;
#18099=CARTESIAN_POINT ( 'NONE',  ( -54.95163769728822700, 213.9548777149308592, -2.149950860017830756 ) ) ;
#18100=CARTESIAN_POINT ( 'NONE',  ( -37.73288769728823411, 201.5309553116392181, -2.393094931466246855 ) ) ;
#18104=CARTESIAN_POINT ( 'NONE',  ( -58.30877896937849414, 212.1620413398627534, -8.530955311639255356 ) ) ;
#18114=CARTESIAN_POINT ( 'NONE',  ( -38.12872103062154849, 203.4690446883607535, 1.626142955000567936 ) ) ;
#18141=CARTESIAN_POINT ( 'NONE',  ( -35.15997103062156270, 213.8393509191290889, 2.350049139982164359 ) ) ;
#18145=CARTESIAN_POINT ( 'NONE',  ( -55.54538769728823411, 211.8571965466039444, -6.469044688360768625 ) ) ;
#18147=CARTESIAN_POINT ( 'NONE',  ( -34.95461230271183695, 207.6069050685336492, -8.469044688360751749 ) ) ;
#18152=CARTESIAN_POINT ( 'NONE',  ( -64.44419563604516554, 203.5000000000000000, 0.1155267958017914542 ) ) ;
#18199=CARTESIAN_POINT ( 'NONE',  ( -63.46205436395489841, 213.2096571498974242, 3.378800118222489601 ) ) ;
#18235=CARTESIAN_POINT ( 'NONE',  ( -62.66294563604517265, 216.1378603801729241, -6.307003348498026796 ) ) ;
#18239=CARTESIAN_POINT ( 'NONE',  ( -51.38169563604516554, 210.1155267958017703, 4.499999999999996447 ) ) ;
#18245=CARTESIAN_POINT ( 'NONE',  ( -49.80580436395490551, 218.5000000000000000, 0.1155267958017064944 ) ) ;
#18277=CARTESIAN_POINT ( 'NONE',  ( -31.98586230271182984, 206.8500491399821328, 5.686928522499748340 ) ) ;
#18279=CARTESIAN_POINT ( 'NONE',  ( -62.06919563604516554, 216.5000000000000000, -0.1155267958017906493 ) ) ;
#18283=CARTESIAN_POINT ( 'NONE',  ( -51.38913769728824121, 207.8500491399821613, -3.954877714930864485 ) ) ;
#18284=CARTESIAN_POINT ( 'NONE',  ( -69.99330436395490551, 210.1155267958017134, -6.500000000000000888 ) ) ;
#18289=CARTESIAN_POINT ( 'NONE',  ( -42.47544563604517265, 216.3070033484980854, 6.137860380172893926 ) ) ;
#18302=CARTESIAN_POINT ( 'NONE',  ( -32.58705436395489841, 205.3262412349647263, -4.842901733360204020 ) ) ;
#18328=CARTESIAN_POINT ( 'NONE',  ( -64.04836230271183695, 206.0451222850691977, -2.149950860017851184 ) ) ;
#18332=CARTESIAN_POINT ( 'NONE',  ( -49.60788769728823411, 216.4690446883607535, 1.857196546604031662 ) ) ;
#18333=CARTESIAN_POINT ( 'NONE',  ( -69.99330436395489130, 210.1155267958016850, -8.500000000000003553 ) ) ;
#18337=CARTESIAN_POINT ( 'NONE',  ( -60.48586230271183695, 206.8500491399821328, 5.686928522499748340 ) ) ;
#18349=CARTESIAN_POINT ( 'NONE',  ( -32.19122103062156270, 207.8379586601371329, -8.530955311639223382 ) ) ;
#18427=CARTESIAN_POINT ( 'NONE',  ( -57.51711230271184405, 218.4690446883607535, -2.393094931466363651 ) ) ;
#18432=CARTESIAN_POINT ( 'NONE',  ( -42.67336230271183695, 213.9548777149308023, 2.149950860017852960 ) ) ;
#18439=CARTESIAN_POINT ( 'NONE',  ( -44.26413769728823411, 214.1499508600179240, 7.418979330068584233 ) ) ;
#18444=UNCERTAINTY_MEASURE_WITH_UNIT (LENGTH_MEASURE( 1.000000000000000082E-05 ), #20330, 'distance_accuracy_value', 'NONE');
#18463=DIRECTION ( 'NONE',  ( -0.1155267958017757585, -0.9933043639548629899, 1.378486719154166141E-14 ) ) ;
#18472=CARTESIAN_POINT ( 'NONE',  ( -40.29836230271182984, 204.3130714775002446, -3.149950860017828091 ) ) ;
#18473=CARTESIAN_POINT ( 'NONE',  ( -51.18377896937847993, 208.3738570449995109, 6.530955311639247363 ) ) ;
#18477=CARTESIAN_POINT ( 'NONE',  ( -47.82663769728823411, 206.0451222850691408, 2.149950860017832532 ) ) ;
#18479=CARTESIAN_POINT ( 'NONE',  ( -34.76413769728823411, 214.1499508600179240, 7.418979330068584233 ) ) ;
#18483=CARTESIAN_POINT ( 'NONE',  ( -48.01711230271184405, 218.4690446883607535, -2.393094931466363651 ) ) ;
#18494=CARTESIAN_POINT ( 'NONE',  ( -32.19122103062156981, 208.3738570449993404, -6.530955311639226935 ) ) ;
#18523=CARTESIAN_POINT ( 'NONE',  ( -61.47544563604516554, 213.3788001182224718, 3.209657149897419348 ) ) ;
#18528=CARTESIAN_POINT ( 'NONE',  ( -52.37872103062156270, 203.4690446883607535, 1.626142955000567936 ) ) ;
#18529=CARTESIAN_POINT ( 'NONE',  ( -64.84747103062156270, 214.3500491399821044, -7.303452534266878793 ) ) ;
#18534=CARTESIAN_POINT ( 'NONE',  ( -39.50669563604517265, 209.8844732041982013, -6.500000000000000888 ) ) ;
#18542=CARTESIAN_POINT ( 'NONE',  ( -61.08705436395489841, 205.3262412349647548, -4.842901733360204908 ) ) ;
#18547=CARTESIAN_POINT ( 'NONE',  ( -39.51413769728823411, 214.1499508600179240, 7.418979330068584233 ) ) ;
#18620=CARTESIAN_POINT ( 'NONE',  ( -60.48586230271183695, 205.8500491399821613, 7.418979330068642852 ) ) ;
#18625=CARTESIAN_POINT ( 'NONE',  ( -41.09002896937850124, 206.1606490808709111, 2.350049139982143931 ) ) ;
#18632=CARTESIAN_POINT ( 'NONE',  ( -50.39955436395490551, 216.3070033484980002, -6.137860380172975638 ) ) ;
#18662=CARTESIAN_POINT ( 'NONE',  ( -41.48586230271182984, 206.8500491399821328, 5.686928522499748340 ) ) ;
#18663=CARTESIAN_POINT ( 'NONE',  ( -51.38169563604516554, 210.1155267958017703, 6.500000000000000888 ) ) ;
#18666=CARTESIAN_POINT ( 'NONE',  ( -51.58705436395489841, 206.7903428501026042, -3.378800118222489157 ) ) ;
#18667=CARTESIAN_POINT ( 'NONE',  ( -52.77455436395490551, 205.1570982666397356, 4.673758765035198159 ) ) ;
#18672=CARTESIAN_POINT ( 'NONE',  ( -45.84002896937850124, 202.6965474657332038, 4.350049139982197666 ) ) ;
#18685=CARTESIAN_POINT ( 'NONE',  ( -40.50372103062156981, 216.5309553116391612, -1.626142955000564383 ) ) ;
#18714=CARTESIAN_POINT ( 'NONE',  ( -58.90252896937851546, 207.6499508600178387, -3.839350919129087547 ) ) ;
#18718=CARTESIAN_POINT ( 'NONE',  ( -42.68080436395489841, 203.5000000000000000, -0.1155267958017335561 ) ) ;
#18719=CARTESIAN_POINT ( 'NONE',  ( -53.76413769728823411, 214.1499508600179240, 7.418979330068584233 ) ) ;
#18724=CARTESIAN_POINT ( 'NONE',  ( -46.43377896937850835, 208.3738570449995109, 6.530955311639247363 ) ) ;
#18731=CARTESIAN_POINT ( 'NONE',  ( -55.34747103062156981, 213.3500491399821328, -5.571401726697985168 ) ) ;
#18735=CARTESIAN_POINT ( 'NONE',  ( -34.36830436395490551, 209.8844732041983150, 8.500000000000003553 ) ) ;
#18745=CARTESIAN_POINT ( 'NONE',  ( -61.87872103062154849, 203.4690446883607535, 1.626142955000567936 ) ) ;
#18759=CARTESIAN_POINT ( 'NONE',  ( -51.19122103062157692, 208.9097554298617752, -4.530955311639240257 ) ) ;
#18809=CARTESIAN_POINT ( 'NONE',  ( -55.34002896937850124, 202.6965474657332038, 4.350049139982197666 ) ) ;
#18812=CARTESIAN_POINT ( 'NONE',  ( -49.79836230271183695, 206.0451222850691977, -2.149950860017851184 ) ) ;
#18818=CARTESIAN_POINT ( 'NONE',  ( -48.22247103062156981, 205.6499508600178956, 7.303452534266880569 ) ) ;
#18824=CARTESIAN_POINT ( 'NONE',  ( -35.15997103062156270, 215.5714017266979852, 3.350049139982118618 ) ) ;
#18847=CARTESIAN_POINT ( 'NONE',  ( -36.53794563604517265, 205.3262412349648116, 4.842901733360249317 ) ) ;
#18848=CARTESIAN_POINT ( 'NONE',  ( -48.80877896937850835, 211.6261429550004607, -6.530955311639245586 ) ) ;
#18851=CARTESIAN_POINT ( 'NONE',  ( -53.17038769728823411, 208.6787018382581778, 4.469044688360752637 ) ) ;
#18852=CARTESIAN_POINT ( 'NONE',  ( -57.32663769728823411, 204.3130714775002730, 3.149950860017883603 ) ) ;
#18856=CARTESIAN_POINT ( 'NONE',  ( -46.23586230271182984, 205.8500491399821613, 7.418979330068642852 ) ) ;
#18868=CARTESIAN_POINT ( 'NONE',  ( -35.95163769728823411, 215.6869285224996986, -3.149950860017881382 ) ) ;
#18896=CARTESIAN_POINT ( 'NONE',  ( -56.92336230271183695, 213.9548777149308023, 2.149950860017852960 ) ) ;
#18901=CARTESIAN_POINT ( 'NONE',  ( -43.07663769728823411, 204.3130714775002730, 3.149950860017883603 ) ) ;
#18902=CARTESIAN_POINT ( 'NONE',  ( -59.89955436395489841, 216.3070033484980002, -6.137860380172975638 ) ) ;
#18907=CARTESIAN_POINT ( 'NONE',  ( -45.04836230271183695, 204.3130714775002446, -3.149950860017828091 ) ) ;
#18916=CARTESIAN_POINT ( 'NONE',  ( -59.30580436395489841, 216.5000000000000000, 0.1155267958017343610 ) ) ;
#18920=CARTESIAN_POINT ( 'NONE',  ( -43.47247103062156981, 205.6499508600178956, 7.303452534266880569 ) ) ;
#18943=CARTESIAN_POINT ( 'NONE',  ( -51.78497103062156981, 206.1606490808709111, -2.350049139982163027 ) ) ;
#18991=CARTESIAN_POINT ( 'NONE',  ( -61.47544563604516554, 216.3070033484980854, 6.137860380172893926 ) ) ;
#18994=CARTESIAN_POINT ( 'NONE',  ( -33.37127896937850124, 214.5309553116392749, 1.090244570138288127 ) ) ;
#19033=CARTESIAN_POINT ( 'NONE',  ( -50.39211230271182274, 203.5309553116391612, 1.857196546604092280 ) ) ;
#19039=CARTESIAN_POINT ( 'NONE',  ( -48.61830436395490551, 209.8844732041982297, 4.499999999999996447 ) ) ;
#19041=CARTESIAN_POINT ( 'NONE',  ( -61.48288769728821990, 203.5309553116391612, -1.857196546604028775 ) ) ;
#19045=CARTESIAN_POINT ( 'NONE',  ( -49.00669563604517265, 209.8844732041981729, -8.500000000000003553 ) ) ;
#19080=CARTESIAN_POINT ( 'NONE',  ( -64.84002896937850835, 204.4285982733020433, 3.350049139982171020 ) ) ;
#19082=CARTESIAN_POINT ( 'NONE',  ( -57.31919563604516554, 214.5000000000000284, -0.1155267958017627827 ) ) ;
#19086=CARTESIAN_POINT ( 'NONE',  ( -42.48288769728824121, 203.5309553116391612, -1.857196546604028775 ) ) ;
#19087=CARTESIAN_POINT ( 'NONE',  ( -54.95163769728822700, 217.4189793300686233, -4.149950860017907139 ) ) ;
#19091=CARTESIAN_POINT ( 'NONE',  ( -41.09002896937850124, 204.4285982733020433, 3.350049139982171020 ) ) ;
#19102=CARTESIAN_POINT ( 'NONE',  ( -56.13913769728823411, 206.8500491399821044, -5.686928522499717253 ) ) ;
#19106=CARTESIAN_POINT ( 'NONE',  ( -34.56622103062156981, 212.1620413398628671, 8.530955311639223382 ) ) ;
#19133=CARTESIAN_POINT ( 'NONE',  ( -54.95163769728822700, 213.9548777149308592, -2.149950860017830756 ) ) ;
#19181=CARTESIAN_POINT ( 'NONE',  ( -54.15252896937849414, 205.6499508600178103, -7.303452534266820173 ) ) ;
#19184=CARTESIAN_POINT ( 'NONE',  ( -32.77752896937849414, 212.3500491399821613, 3.839350919129088435 ) ) ;
#19223=CARTESIAN_POINT ( 'NONE',  ( -53.55877896937850124, 211.6261429550004607, -6.530955311639245586 ) ) ;
#19224=ADVANCED_BREP_SHAPE_REPRESENTATION ( '', ( #8321, #17215 ), #2050 ) ;
#19227=CARTESIAN_POINT ( 'NONE',  ( -33.57663769728823411, 206.0451222850691408, 2.149950860017832532 ) ) ;
#19228=CARTESIAN_POINT ( 'NONE',  ( -62.47247103062156981, 206.6499508600178672, 5.571401726697986057 ) ) ;
#19232=CARTESIAN_POINT ( 'NONE',  ( -32.18377896937850124, 207.8379586601372750, 8.530955311639258909 ) ) ;
#19272=CARTESIAN_POINT ( 'NONE',  ( -59.49627896937850124, 203.4690446883607535, -1.626142955000504209 ) ) ;
#19274=CARTESIAN_POINT ( 'NONE',  ( -53.36086230271183695, 212.1499508600178387, -3.954877714930852495 ) ) ;
#19278=CARTESIAN_POINT ( 'NONE',  ( -33.97247103062156270, 206.6499508600178672, 5.571401726697986057 ) ) ;
#19279=CARTESIAN_POINT ( 'NONE',  ( -61.87872103062156981, 201.4690446883607819, 2.162041339862843525 ) ) ;
#19286=CARTESIAN_POINT ( 'NONE',  ( -40.29836230271182984, 204.3130714775002446, -3.149950860017828091 ) ) ;
#19294=CARTESIAN_POINT ( 'NONE',  ( -57.72247103062156270, 206.6499508600178672, 5.571401726697986057 ) ) ;
#19298=CARTESIAN_POINT ( 'NONE',  ( -59.10788769728823411, 216.4690446883607535, 1.857196546604031662 ) ) ;
#19324=CARTESIAN_POINT ( 'NONE',  ( -58.31622103062156981, 211.0902445701382533, 4.530955311639240257 ) ) ;
#19369=CARTESIAN_POINT ( 'NONE',  ( -42.47544563604517265, 216.3070033484980854, 6.137860380172893926 ) ) ;
#19372=CARTESIAN_POINT ( 'NONE',  ( -67.61086230271183695, 213.1499508600178387, -5.686928522499747451 ) ) ;
#19376=CARTESIAN_POINT ( 'NONE',  ( -37.93080436395489841, 203.5000000000000000, -0.1155267958017335561 ) ) ;
#19406=CARTESIAN_POINT ( 'NONE',  ( -44.05877896937847993, 211.6261429550004607, -6.530955311639245586 ) ) ;
#19408=CARTESIAN_POINT ( 'NONE',  ( -67.80877896937849414, 211.0902445701383101, -4.530955311639234040 ) ) ;
#19409=CARTESIAN_POINT ( 'NONE',  ( -53.17038769728823411, 208.1428034533959703, 6.469044688360770401 ) ) ;
#19413=CARTESIAN_POINT ( 'NONE',  ( -32.97544563604516554, 216.3070033484980854, 6.137860380172893926 ) ) ;
#19434=CARTESIAN_POINT ( 'NONE',  ( -68.80580436395490551, 216.5000000000000000, 0.1155267958017343610 ) ) ;
#19456=CARTESIAN_POINT ( 'NONE',  ( -60.28794563604517975, 206.7903428501025758, 3.378800118222471838 ) ) ;
#19459=CARTESIAN_POINT ( 'NONE',  ( -32.19122103062156981, 208.3738570449993404, -6.530955311639226935 ) ) ;
#19460=CARTESIAN_POINT ( 'NONE',  ( -56.13913769728823411, 205.8500491399820760, -7.418979330068584233 ) ) ;
#19466=CARTESIAN_POINT ( 'NONE',  ( -67.01711230271185116, 218.4690446883607535, -2.393094931466363651 ) ) ;
#19474=CARTESIAN_POINT ( 'NONE',  ( -45.05580436395489841, 216.5000000000000000, 0.1155267958017343610 ) ) ;
#19478=CARTESIAN_POINT ( 'NONE',  ( -64.25372103062154849, 216.5309553116391612, -1.626142955000564383 ) ) ;
#19505=CARTESIAN_POINT ( 'NONE',  ( -54.35788769728822700, 214.4690446883608104, 1.321298161741840893 ) ) ;
#19508=CARTESIAN_POINT ( 'NONE',  ( -67.61830436395489130, 209.8844732041982581, 6.500000000000000888 ) ) ;
#19550=CARTESIAN_POINT ( 'NONE',  ( -46.03794563604517975, 203.8621396198271043, 6.307003348498029460 ) ) ;
#19553=CARTESIAN_POINT ( 'NONE',  ( -36.34002896937849414, 206.1606490808709111, 2.350049139982143931 ) ) ;
#19556=CARTESIAN_POINT ( 'NONE',  ( -45.45163769728822700, 215.6869285224996986, -3.149950860017881382 ) ) ;
#19590=CARTESIAN_POINT ( 'NONE',  ( -40.10044563604517265, 205.1570982666397072, -4.673758765035155527 ) ) ;
#19594=CARTESIAN_POINT ( 'NONE',  ( -31.99330436395490196, 210.1155267958017703, -4.499999999999996447 ) ) ;
#19595=CARTESIAN_POINT ( 'NONE',  ( -49.21205436395490551, 214.6737587650352168, 4.842901733360204908 ) ) ;
#19599=CARTESIAN_POINT ( 'NONE',  ( -35.94419563604516554, 201.5000000000000000, 0.1155267958018195706 ) ) ;
#19616=EDGE_CURVE ( 'NONE', #29947, #16114, #2, .T. ) ;
#19621=CARTESIAN_POINT ( 'NONE',  ( -63.85788769728821279, 216.4690446883607535, 1.857196546604031662 ) ) ;
#19642=CARTESIAN_POINT ( 'NONE',  ( -59.29836230271183695, 204.3130714775002446, -3.149950860017828091 ) ) ;
#19644=CARTESIAN_POINT ( 'NONE',  ( -47.42336230271184405, 213.9548777149308023, 2.149950860017852960 ) ) ;
#19645=DIRECTION ( 'NONE',  ( 1.000000000000000000, 0.000000000000000000, 0.000000000000000000 ) ) ;
#19648=CARTESIAN_POINT ( 'NONE',  ( -39.71205436395490551, 214.6737587650352168, 4.842901733360204908 ) ) ;
#19649=CARTESIAN_POINT ( 'NONE',  ( -42.87872103062157692, 201.4690446883607819, 2.162041339862843525 ) ) ;
#19653=CARTESIAN_POINT ( 'NONE',  ( -31.19419563604516910, 203.5000000000000000, 0.1155267958017914542 ) ) ;
#19661=CARTESIAN_POINT ( 'NONE',  ( -40.10788769728823411, 216.4690446883607535, 1.857196546604031662 ) ) ;
#19666=CARTESIAN_POINT ( 'NONE',  ( -66.62872103062152007, 203.4690446883607535, 1.626142955000567936 ) ) ;
#19691=CARTESIAN_POINT ( 'NONE',  ( -46.24330436395489841, 210.1155267958017703, -4.499999999999996447 ) ) ;
#19741=CARTESIAN_POINT ( 'NONE',  ( -46.63169563604517265, 210.1155267958018271, 8.500000000000003553 ) ) ;
#19745=CARTESIAN_POINT ( 'NONE',  ( -68.00669563604516554, 209.8844732041982013, -6.500000000000000888 ) ) ;
#19748=CARTESIAN_POINT ( 'NONE',  ( -45.05580436395489841, 216.5000000000000000, 0.1155267958017343610 ) ) ;
#19781=CARTESIAN_POINT ( 'NONE',  ( -44.85044563604515133, 205.1570982666397072, -4.673758765035155527 ) ) ;
#19784=CARTESIAN_POINT ( 'NONE',  ( -38.92038769728823411, 208.6787018382581778, 4.469044688360752637 ) ) ;
#19785=CARTESIAN_POINT ( 'NONE',  ( -49.60788769728823411, 216.4690446883607535, 1.857196546604031662 ) ) ;
#19790=CARTESIAN_POINT ( 'NONE',  ( -69.79538769728823411, 212.3930949314662371, -8.469044688360781947 ) ) ;
#19826=CARTESIAN_POINT ( 'NONE',  ( -56.92336230271182984, 215.6869285224997270, 3.149950860017831200 ) ) ;
#19828=CARTESIAN_POINT ( 'NONE',  ( -42.07961230271182984, 211.3212981617417938, 4.469044688360757966 ) ) ;
#19831=CARTESIAN_POINT ( 'NONE',  ( -68.60788769728823411, 214.4690446883608104, 1.321298161741840893 ) ) ;
#19832=CARTESIAN_POINT ( 'NONE',  ( -45.84747103062156981, 214.3500491399821044, -7.303452534266878793 ) ) ;
#19837=CARTESIAN_POINT ( 'NONE',  ( -35.15252896937850124, 206.6499508600178387, -5.571401726697954970 ) ) ;
#19848=CARTESIAN_POINT ( 'NONE',  ( -64.84747103062156270, 213.3500491399821328, -5.571401726697985168 ) ) ;
#19873=CARTESIAN_POINT ( 'NONE',  ( -49.60788769728823411, 214.4690446883608104, 1.321298161741840893 ) ) ;
#19878=CARTESIAN_POINT ( 'NONE',  ( -69.79538769728823411, 211.8571965466039444, -6.469044688360768625 ) ) ;
#19925=CARTESIAN_POINT ( 'NONE',  ( -59.29836230271183695, 204.3130714775002446, -3.149950860017828091 ) ) ;
#19928=CARTESIAN_POINT ( 'NONE',  ( -41.09747103062156981, 213.3500491399821328, -5.571401726697985168 ) ) ;
#19958=CARTESIAN_POINT ( 'NONE',  ( -46.43377896937850835, 208.3738570449995109, 6.530955311639247363 ) ) ;
#19961=CARTESIAN_POINT ( 'NONE',  ( -38.52455436395490551, 206.6211998817774997, 3.209657149897401585 ) ) ;
#19962=CARTESIAN_POINT ( 'NONE',  ( -47.03497103062156981, 204.4285982733020148, -3.350049139982115509 ) ) ;
#19968=CARTESIAN_POINT ( 'NONE',  ( -33.37127896937850124, 218.5309553116392465, 2.162041339862725842 ) ) ;
#19985=CARTESIAN_POINT ( 'NONE',  ( -63.65997103062156981, 215.5714017266979852, 3.350049139982118618 ) ) ;
#20002=CARTESIAN_POINT ( 'NONE',  ( -44.25669563604516554, 209.8844732041982013, -6.500000000000000888 ) ) ;
#20004=CARTESIAN_POINT ( 'NONE',  ( -42.67336230271183695, 213.9548777149308023, 2.149950860017852960 ) ) ;
#20007=CARTESIAN_POINT ( 'NONE',  ( -67.81622103062157692, 211.0902445701382533, 4.530955311639240257 ) ) ;
#20008=CARTESIAN_POINT ( 'NONE',  ( -43.86830436395490551, 209.8844732041983150, 8.500000000000003553 ) ) ;
#20012=CARTESIAN_POINT ( 'NONE',  ( -32.77752896937850124, 213.3500491399821613, 5.571401726697954970 ) ) ;
#20024=CARTESIAN_POINT ( 'NONE',  ( -64.05580436395490551, 216.5000000000000000, 0.1155267958017343610 ) ) ;
#20051=CARTESIAN_POINT ( 'NONE',  ( -42.08705436395490551, 206.7903428501026042, -3.378800118222489157 ) ) ;
#20056=CARTESIAN_POINT ( 'NONE',  ( -68.80580436395490551, 216.5000000000000000, 0.1155267958017343610 ) ) ;
#20102=CARTESIAN_POINT ( 'NONE',  ( -47.23288769728823411, 203.5309553116391612, -1.857196546604028775 ) ) ;
#20136=CARTESIAN_POINT ( 'NONE',  ( -48.21502896937850124, 215.5714017266979567, -3.350049139982168800 ) ) ;
#20138=SURFACE_STYLE_USAGE ( .BOTH. , #5347 ) ;
#20140=CARTESIAN_POINT ( 'NONE',  ( -56.72544563604517265, 213.3788001182224718, 3.209657149897419348 ) ) ;
#20142=CARTESIAN_POINT ( 'NONE',  ( -43.27455436395490551, 205.1570982666397356, 4.673758765035198159 ) ) ;
#20148=CARTESIAN_POINT ( 'NONE',  ( -59.50372103062157692, 218.5309553116391896, -2.162041339862839084 ) ) ;
#20166=CARTESIAN_POINT ( 'NONE',  ( -59.10788769728823411, 216.4690446883607535, 1.857196546604031662 ) ) ;
#20184=CARTESIAN_POINT ( 'NONE',  ( -55.93377896937849414, 208.3738570449995109, 6.530955311639247363 ) ) ;
#20186=CARTESIAN_POINT ( 'NONE',  ( -45.64211230271183695, 205.5309553116392465, 1.321298161741817356 ) ) ;
#20190=CARTESIAN_POINT ( 'NONE',  ( -57.72247103062156270, 207.6499508600178387, 3.839350919129076445 ) ) ;
#20191=CARTESIAN_POINT ( 'NONE',  ( -50.20163769728823411, 217.4189793300686233, -4.149950860017907139 ) ) ;
#20195=CARTESIAN_POINT ( 'NONE',  ( -37.13169563604516554, 210.1155267958017703, 6.500000000000000888 ) ) ;
#20206=CARTESIAN_POINT ( 'NONE',  ( -45.05580436395489841, 216.5000000000000000, 0.1155267958017343610 ) ) ;
#20216=MECHANICAL_DESIGN_GEOMETRIC_PRESENTATION_REPRESENTATION('',(#9309),#6902);
#20234=CARTESIAN_POINT ( 'NONE',  ( -40.70163769728823411, 213.9548777149308592, -2.149950860017830756 ) ) ;
#20292=CARTESIAN_POINT ( 'NONE',  ( -37.33705436395490551, 205.3262412349647263, -4.842901733360204020 ) ) ;
#20328=CARTESIAN_POINT ( 'NONE',  ( -65.63169563604516554, 210.1155267958018271, 8.500000000000003553 ) ) ;
#20330=( LENGTH_UNIT ( ) NAMED_UNIT ( * ) SI_UNIT ( .MILLI., .METRE. ) );
#20333=CARTESIAN_POINT ( 'NONE',  ( -54.15252896937849414, 207.6499508600178387, -3.839350919129087547 ) ) ;
#20334=CARTESIAN_POINT ( 'NONE',  ( -45.84747103062156981, 213.3500491399821328, -5.571401726697985168 ) ) ;
#20340=CARTESIAN_POINT ( 'NONE',  ( -62.47247103062156981, 205.6499508600178956, 7.303452534266880569 ) ) ;
#20345=CARTESIAN_POINT ( 'NONE',  ( -42.48288769728824121, 203.5309553116391896, -1.857196546604028997 ) ) ;
#20357=CARTESIAN_POINT ( 'NONE',  ( -55.94122103062156270, 208.3738570449993404, -6.530955311639226935 ) ) ;
#20376=CARTESIAN_POINT ( 'NONE',  ( -52.17336230271183695, 215.6869285224997270, 3.149950860017831200 ) ) ;
#20378=CARTESIAN_POINT ( 'NONE',  ( -32.77752896937849414, 212.3500491399821613, 3.839350919129088435 ) ) ;
#20381=CARTESIAN_POINT ( 'NONE',  ( -53.76413769728823411, 212.1499508600178387, 3.954877714930865817 ) ) ;
#20382=CARTESIAN_POINT ( 'NONE',  ( -48.61830436395490551, 209.8844732041983150, 8.500000000000003553 ) ) ;
#20387=CARTESIAN_POINT ( 'NONE',  ( -59.49627896937850835, 201.4690446883607251, -2.162041339862721845 ) ) ;
#20398=CARTESIAN_POINT ( 'NONE',  ( -52.18080436395490551, 203.5000000000000000, -0.1155267958017335561 ) ) ;
#20424=CARTESIAN_POINT ( 'NONE',  ( -38.92038769728823411, 208.6787018382581778, 4.469044688360752637 ) ) ;
#20429=CARTESIAN_POINT ( 'NONE',  ( -53.76413769728823411, 213.1499508600178672, 5.686928522499718142 ) ) ;
#20430=CARTESIAN_POINT ( 'NONE',  ( -44.65252896937850835, 205.6499508600178103, -7.303452534266820173 ) ) ;
#20444=CARTESIAN_POINT ( 'NONE',  ( -69.20163769728823411, 215.6869285224996986, -3.149950860017881382 ) ) ;
#20480=CARTESIAN_POINT ( 'NONE',  ( -35.75372103062156981, 216.5309553116391612, -1.626142955000564383 ) ) ;
#20517=CARTESIAN_POINT ( 'NONE',  ( -32.97544563604516554, 214.8429017333602360, 4.673758765035156415 ) ) ;
#20521=CARTESIAN_POINT ( 'NONE',  ( -53.16294563604516554, 213.2096571498974527, -3.378800118222469617 ) ) ;
#20522=CARTESIAN_POINT ( 'NONE',  ( -31.99330436395490196, 210.1155267958017134, -6.500000000000000888 ) ) ;
#20526=CARTESIAN_POINT ( 'NONE',  ( -57.52455436395489841, 203.6929966515020283, 6.137860380172978303 ) ) ;
#20531=CARTESIAN_POINT ( 'NONE',  ( -44.26413769728823411, 213.1499508600178672, 5.686928522499718142 ) ) ;
#20543=CARTESIAN_POINT ( 'NONE',  ( -57.92038769728821990, 208.1428034533959703, 6.469044688360770401 ) ) ;
#20558=CARTESIAN_POINT ( 'NONE',  ( -47.22544563604515844, 214.8429017333602360, 4.673758765035156415 ) ) ;
#20560=CARTESIAN_POINT ( 'NONE',  ( -35.74627896937850124, 205.4690446883607535, -1.090244570138286351 ) ) ;
#20564=CARTESIAN_POINT ( 'NONE',  ( -64.05580436395490551, 214.5000000000000284, 0.1155267958017899832 ) ) ;
#20565=CARTESIAN_POINT ( 'NONE',  ( -65.24330436395489130, 210.1155267958017134, -6.500000000000000888 ) ) ;
#20569=CARTESIAN_POINT ( 'NONE',  ( -52.17336230271184405, 217.4189793300686233, 4.149950860017807663 ) ) ;
#20580=CARTESIAN_POINT ( 'NONE',  ( -55.94122103062156270, 208.3738570449993404, -6.530955311639226935 ) ) ;
#20610=CARTESIAN_POINT ( 'NONE',  ( -34.56622103062156981, 211.0902445701382533, 4.530955311639240257 ) ) ;
#20614=CARTESIAN_POINT ( 'NONE',  ( -56.73288769728823411, 203.5309553116391612, -1.857196546604028775 ) ) ;
#20615=CARTESIAN_POINT ( 'NONE',  ( -48.80877896937850124, 212.1620413398627534, -8.530955311639255356 ) ) ;
#20620=CARTESIAN_POINT ( 'NONE',  ( -56.92336230271182984, 215.6869285224997270, 3.149950860017831200 ) ) ;
#20664=CARTESIAN_POINT ( 'NONE',  ( -63.26413769728823411, 212.1499508600178387, 3.954877714930865817 ) ) ;
#20699=CARTESIAN_POINT ( 'NONE',  ( -35.94419563604516554, 203.5000000000000000, 0.1155267958017914542 ) ) ;
#20702=CARTESIAN_POINT ( 'NONE',  ( -57.91294563604517265, 213.2096571498974527, -3.378800118222469617 ) ) ;
#20703=CARTESIAN_POINT ( 'NONE',  ( -33.97247103062156270, 206.6499508600178672, 5.571401726697986057 ) ) ;
#20709=CARTESIAN_POINT ( 'NONE',  ( -64.64955436395490551, 216.3070033484980002, -6.137860380172975638 ) ) ;
#20715=CARTESIAN_POINT ( 'NONE',  ( -38.32663769728824121, 204.3130714775002730, 3.149950860017883603 ) ) ;
#20727=CARTESIAN_POINT ( 'NONE',  ( -51.78497103062156981, 204.4285982733020148, -3.350049139982115509 ) ) ;
#20744=CARTESIAN_POINT ( 'NONE',  ( -47.42336230271183695, 215.6869285224997270, 3.149950860017831200 ) ) ;
#20746=CARTESIAN_POINT ( 'NONE',  ( -31.19419563604517265, 205.4999999999999716, 0.1155267958017633378 ) ) ;
#20750=CARTESIAN_POINT ( 'NONE',  ( -56.13913769728823411, 207.8500491399821613, -3.954877714930864485 ) ) ;
#20751=CARTESIAN_POINT ( 'NONE',  ( -65.44122103062157692, 208.3738570449993404, -6.530955311639226935 ) ) ;
#20755=CARTESIAN_POINT ( 'NONE',  ( -60.68377896937850835, 207.8379586601372750, 8.530955311639258909 ) ) ;
#20768=CARTESIAN_POINT ( 'NONE',  ( -48.61830436395490551, 209.8844732041982581, 6.500000000000000888 ) ) ;
#20796=CARTESIAN_POINT ( 'NONE',  ( -36.34747103062156981, 212.3500491399821613, -3.839350919129076445 ) ) ;
#20801=CARTESIAN_POINT ( 'NONE',  ( -59.30580436395489841, 216.5000000000000000, 0.1155267958017343610 ) ) ;
#20802=CARTESIAN_POINT ( 'NONE',  ( -66.03497103062157692, 202.6965474657331185, -4.350049139982091084 ) ) ;
#20808=CARTESIAN_POINT ( 'NONE',  ( -60.68377896937848703, 208.3738570449995109, 6.530955311639247363 ) ) ;
#20857=CARTESIAN_POINT ( 'NONE',  ( -34.36830436395490551, 209.8844732041982581, 6.500000000000000888 ) ) ;
#20890=CARTESIAN_POINT ( 'NONE',  ( -64.64211230271182274, 201.5309553116392181, 2.393094931466368980 ) ) ;
#20893=CARTESIAN_POINT ( 'NONE',  ( -63.65252896937850124, 207.6499508600178387, -3.839350919129087547 ) ) ;
#20901=CARTESIAN_POINT ( 'NONE',  ( -62.27455436395490551, 203.6929966515020283, 6.137860380172978303 ) ) ;
#20939=CARTESIAN_POINT ( 'NONE',  ( -39.90252896937850124, 206.6499508600178387, -5.571401726697954970 ) ) ;
#20941=CARTESIAN_POINT ( 'NONE',  ( -65.63169563604516554, 210.1155267958017703, 6.500000000000000888 ) ) ;
#20945=CARTESIAN_POINT ( 'NONE',  ( -58.90997103062156981, 213.8393509191290889, 2.350049139982164359 ) ) ;
#20946=CARTESIAN_POINT ( 'NONE',  ( -67.61830436395489130, 209.8844732041982581, 6.500000000000000888 ) ) ;
#20950=CARTESIAN_POINT ( 'NONE',  ( -64.44419563604517975, 201.5000000000000000, 0.1155267958018195706 ) ) ;
#20962=CARTESIAN_POINT ( 'NONE',  ( -55.34747103062156981, 213.3500491399821328, -5.571401726697985168 ) ) ;
#20989=CARTESIAN_POINT ( 'NONE',  ( -37.53497103062155560, 206.1606490808709111, -2.350049139982163027 ) ) ;
#20993=CARTESIAN_POINT ( 'NONE',  ( -59.50372103062156981, 216.5309553116391612, -1.626142955000564383 ) ) ;
#20994=CARTESIAN_POINT ( 'NONE',  ( -33.56919563604517265, 218.5000000000000000, -0.1155267958018185298 ) ) ;
#20999=CARTESIAN_POINT ( 'NONE',  ( -61.87127896937849414, 216.5309553116391612, 1.626142955000506873 ) ) ;
#21008=CARTESIAN_POINT ( 'NONE',  ( -63.26413769728824121, 213.1499508600178672, 5.686928522499718142 ) ) ;
#21045=CARTESIAN_POINT ( 'NONE',  ( -33.18080436395490551, 203.5000000000000000, -0.1155267958017335561 ) ) ;
#21085=CARTESIAN_POINT ( 'NONE',  ( -62.46502896937850124, 217.3034525342667962, -4.350049139982195001 ) ) ;
#21087=CARTESIAN_POINT ( 'NONE',  ( -39.50669563604516554, 209.8844732041982297, -4.499999999999996447 ) ) ;
#21093=CARTESIAN_POINT ( 'NONE',  ( -45.25372103062157692, 218.5309553116391896, -2.162041339862839084 ) ) ;
#21101=CARTESIAN_POINT ( 'NONE',  ( -34.36830436395490551, 209.8844732041982581, 6.500000000000000888 ) ) ;
#21125=CARTESIAN_POINT ( 'NONE',  ( -40.49627896937849414, 203.4690446883607535, -1.626142955000504209 ) ) ;
#21128=CARTESIAN_POINT ( 'NONE',  ( -66.81919563604517975, 216.5000000000000000, -0.1155267958017906493 ) ) ;
#21131=CARTESIAN_POINT ( 'NONE',  ( -48.02455436395490551, 206.6211998817774997, 3.209657149897401585 ) ) ;
#21133=CARTESIAN_POINT ( 'NONE',  ( -33.77455436395489841, 203.6929966515020283, 6.137860380172978303 ) ) ;
#21137=CARTESIAN_POINT ( 'NONE',  ( -58.50669563604516554, 209.8844732041981729, -8.500000000000003553 ) ) ;
#21147=CARTESIAN_POINT ( 'NONE',  ( -42.08705436395489841, 205.3262412349647263, -4.842901733360204020 ) ) ;
#21175=CARTESIAN_POINT ( 'NONE',  ( -67.01711230271185116, 214.4690446883608104, -1.321298161741814914 ) ) ;
#21179=CARTESIAN_POINT ( 'NONE',  ( -64.25372103062154849, 216.5309553116391612, -1.626142955000564383 ) ) ;
#21180=CARTESIAN_POINT ( 'NONE',  ( -32.57961230271184405, 212.3930949314663792, 8.469044688360751749 ) ) ;
#21186=CARTESIAN_POINT ( 'NONE',  ( -54.94419563604517265, 203.5000000000000000, 0.1155267958017914542 ) ) ;
#21195=CARTESIAN_POINT ( 'NONE',  ( -68.01413769728823411, 213.1499508600178672, 5.686928522499718142 ) ) ;
#21199=CARTESIAN_POINT ( 'NONE',  ( -41.29538769728824121, 212.3930949314662371, -8.469044688360781947 ) ) ;
#21219=EDGE_CURVE ( 'NONE', #16114, #33325, #12485, .T. ) ;
#21273=CARTESIAN_POINT ( 'NONE',  ( -58.50669563604516554, 209.8844732041981729, -8.500000000000003553 ) ) ;
#21277=CARTESIAN_POINT ( 'NONE',  ( -39.11086230271183695, 212.1499508600178387, -3.954877714930852495 ) ) ;
#21278=CARTESIAN_POINT ( 'NONE',  ( -36.54538769728823411, 211.8571965466039444, -6.469044688360768625 ) ) ;
#21283=CARTESIAN_POINT ( 'NONE',  ( -44.85788769728823411, 218.4690446883607535, 2.393094931466250408 ) ) ;
#21313=CARTESIAN_POINT ( 'NONE',  ( -39.70461230271183695, 208.1428034533958851, -6.469044688360754414 ) ) ;
#21314=CARTESIAN_POINT ( 'NONE',  ( -56.72544563604517265, 214.8429017333602360, 4.673758765035156415 ) ) ;
#21318=CARTESIAN_POINT ( 'NONE',  ( -48.81622103062156981, 211.0902445701382533, 4.530955311639240257 ) ) ;
#21320=CARTESIAN_POINT ( 'NONE',  ( -68.60788769728823411, 216.4690446883607535, 1.857196546604031662 ) ) ;
#21324=CARTESIAN_POINT ( 'NONE',  ( -39.50669563604516554, 209.8844732041981729, -8.500000000000003553 ) ) ;
#21337=CARTESIAN_POINT ( 'NONE',  ( -43.07663769728823411, 204.3130714775002730, 3.149950860017883603 ) ) ;
#21363=CARTESIAN_POINT ( 'NONE',  ( -35.75372103062156981, 214.5309553116392749, -1.090244570138262148 ) ) ;
#21367=CARTESIAN_POINT ( 'NONE',  ( -44.65997103062156981, 215.5714017266979852, 3.350049139982118618 ) ) ;
#21368=CARTESIAN_POINT ( 'NONE',  ( -65.04538769728823411, 212.3930949314662371, -8.469044688360781947 ) ) ;
#21373=CARTESIAN_POINT ( 'NONE',  ( -45.84002896937850124, 204.4285982733020433, 3.350049139982171020 ) ) ;
#21381=CARTESIAN_POINT ( 'NONE',  ( -61.68080436395489841, 203.5000000000000000, -0.1155267958017335561 ) ) ;
#21385=CARTESIAN_POINT ( 'NONE',  ( -41.09747103062157692, 214.3500491399821044, -7.303452534266878793 ) ) ;
#21460=CARTESIAN_POINT ( 'NONE',  ( -51.38169563604516554, 210.1155267958018271, 8.500000000000003553 ) ) ;
#21464=CARTESIAN_POINT ( 'NONE',  ( -43.46502896937849414, 213.8393509191290889, -2.350049139982142155 ) ) ;
#21472=CARTESIAN_POINT ( 'NONE',  ( -43.86830436395490551, 209.8844732041983150, 8.500000000000003553 ) ) ;
#21503=CARTESIAN_POINT ( 'NONE',  ( -43.66294563604516554, 214.6737587650350747, -4.842901733360248429 ) ) ;
#21504=CARTESIAN_POINT ( 'NONE',  ( -53.36086230271183695, 213.1499508600178387, -5.686928522499747451 ) ) ;
#21507=CARTESIAN_POINT ( 'NONE',  ( -42.08705436395490551, 206.7903428501026042, -3.378800118222489157 ) ) ;
#21508=CARTESIAN_POINT ( 'NONE',  ( -59.50372103062156981, 216.5309553116391612, -1.626142955000564383 ) ) ;
#21512=CARTESIAN_POINT ( 'NONE',  ( -42.67336230271183695, 217.4189793300686233, 4.149950860017807663 ) ) ;
#21523=CARTESIAN_POINT ( 'NONE',  ( -38.32663769728824121, 204.3130714775002730, 3.149950860017883603 ) ) ;
#21549=CARTESIAN_POINT ( 'NONE',  ( -51.97544563604517265, 213.3788001182224718, 3.209657149897419348 ) ) ;
#21554=CARTESIAN_POINT ( 'NONE',  ( -50.59747103062156270, 213.3500491399821328, -5.571401726697985168 ) ) ;
#21555=CARTESIAN_POINT ( 'NONE',  ( -54.15997103062156981, 217.3034525342668815, 4.350049139982096413 ) ) ;
#21561=CARTESIAN_POINT ( 'NONE',  ( -40.49627896937849414, 203.4690446883607535, -1.626142955000504209 ) ) ;
#21568=CARTESIAN_POINT ( 'NONE',  ( -56.33705436395489841, 205.3262412349647548, -4.842901733360204908 ) ) ;
#21572=CARTESIAN_POINT ( 'NONE',  ( -36.54538769728824121, 212.3930949314662371, -8.469044688360781947 ) ) ;
#21582=CARTESIAN_POINT ( 'NONE',  ( -69.00372103062157692, 216.5309553116391612, -1.626142955000564383 ) ) ;
#21596=CARTESIAN_POINT ( 'NONE',  ( -59.70163769728823411, 213.9548777149308592, -2.149950860017830756 ) ) ;
#21640=CARTESIAN_POINT ( 'NONE',  ( -60.28794563604517975, 203.8621396198271043, 6.307003348498029460 ) ) ;
#21644=CARTESIAN_POINT ( 'NONE',  ( -48.21502896937850124, 213.8393509191290889, -2.350049139982142155 ) ) ;
#21650=CARTESIAN_POINT ( 'NONE',  ( -44.46205436395490551, 216.1378603801730094, 6.307003348497944195 ) ) ;
#21657=CARTESIAN_POINT ( 'NONE',  ( -35.55580436395490551, 216.5000000000000000, 0.1155267958017343610 ) ) ;
#21681=CARTESIAN_POINT ( 'NONE',  ( -43.06919563604516554, 216.5000000000000000, -0.1155267958017906493 ) ) ;
#21682=CARTESIAN_POINT ( 'NONE',  ( -53.95461230271181563, 208.1428034533959135, -6.469044688360754414 ) ) ;
#21686=CARTESIAN_POINT ( 'NONE',  ( -47.23288769728824121, 205.5309553116392465, -1.321298161741839117 ) ) ;
#21687=CARTESIAN_POINT ( 'NONE',  ( -62.86830436395490551, 209.8844732041982581, 6.500000000000000888 ) ) ;
#21692=CARTESIAN_POINT ( 'NONE',  ( -46.03794563604517975, 203.8621396198271043, 6.307003348498029460 ) ) ;
#21705=CARTESIAN_POINT ( 'NONE',  ( -39.11830436395489841, 209.8844732041982581, 6.500000000000000888 ) ) ;
#21711=EDGE_LOOP ( 'NONE', ( #7493, #7048 ) ) ;
#21733=CARTESIAN_POINT ( 'NONE',  ( -48.80877896937850124, 211.0902445701383101, -4.530955311639234040 ) ) ;
#21737=CARTESIAN_POINT ( 'NONE',  ( -41.09747103062156981, 213.3500491399821328, -5.571401726697985168 ) ) ;
#21738=CARTESIAN_POINT ( 'NONE',  ( -55.94122103062156981, 207.8379586601371329, -8.530955311639223382 ) ) ;
#21744=CARTESIAN_POINT ( 'NONE',  ( -44.65252896937850835, 206.6499508600178387, -5.571401726697954970 ) ) ;
#21751=CARTESIAN_POINT ( 'NONE',  ( -57.52455436395489130, 205.1570982666397640, 4.673758765035199048 ) ) ;
#21756=CARTESIAN_POINT ( 'NONE',  ( -32.38913769728823411, 205.8500491399820760, -7.418979330068584233 ) ) ;
#21781=CARTESIAN_POINT ( 'NONE',  ( -52.18080436395490551, 205.4999999999999716, -0.1155267958017894420 ) ) ;
#21828=CARTESIAN_POINT ( 'NONE',  ( -49.79836230271183695, 202.5810206699313767, -4.149950860017804111 ) ) ;
#21831=CARTESIAN_POINT ( 'NONE',  ( -44.65252896937850835, 207.6499508600178387, -3.839350919129087547 ) ) ;
#21865=CARTESIAN_POINT ( 'NONE',  ( -30.60044563604516199, 205.1570982666397072, -4.673758765035155527 ) ) ;
#21866=CARTESIAN_POINT ( 'NONE',  ( -54.35044563604515133, 205.1570982666397072, -4.673758765035155527 ) ) ;
#21869=CARTESIAN_POINT ( 'NONE',  ( -45.25372103062157692, 214.5309553116392749, -1.090244570138262148 ) ) ;
#21870=CARTESIAN_POINT ( 'NONE',  ( -56.33705436395489841, 205.3262412349647263, -4.842901733360204020 ) ) ;
#21874=CARTESIAN_POINT ( 'NONE',  ( -47.22544563604517265, 216.3070033484980854, 6.137860380172893926 ) ) ;
#21916=CARTESIAN_POINT ( 'NONE',  ( -60.68377896937850835, 208.9097554298617183, 4.530955311639234040 ) ) ;
#21921=CARTESIAN_POINT ( 'NONE',  ( -43.86830436395490551, 209.8844732041982581, 6.500000000000000888 ) ) ;
#21922=CARTESIAN_POINT ( 'NONE',  ( -56.53497103062156270, 202.6965474657331185, -4.350049139982091084 ) ) ;
#21928=CARTESIAN_POINT ( 'NONE',  ( -42.27752896937850124, 213.3500491399821613, 5.571401726697954970 ) ) ;
#21938=CARTESIAN_POINT ( 'NONE',  ( -58.11830436395490551, 209.8844732041982581, 6.500000000000000888 ) ) ;
#21943=CARTESIAN_POINT ( 'NONE',  ( -37.53497103062155560, 202.6965474657331185, -4.350049139982091084 ) ) ;
#21967=CARTESIAN_POINT ( 'NONE',  ( -57.92038769728823411, 208.6787018382581778, 4.469044688360752637 ) ) ;
#22015=CARTESIAN_POINT ( 'NONE',  ( -53.55877896937850124, 212.1620413398627534, -8.530955311639255356 ) ) ;
#22019=CARTESIAN_POINT ( 'NONE',  ( -65.63169563604516554, 210.1155267958017703, 6.500000000000000888 ) ) ;
#22053=CARTESIAN_POINT ( 'NONE',  ( -52.96502896937850124, 215.5714017266979567, -3.350049139982168800 ) ) ;
#22058=CARTESIAN_POINT ( 'NONE',  ( -67.01711230271185116, 214.4690446883608104, -1.321298161741814914 ) ) ;
#22060=CARTESIAN_POINT ( 'NONE',  ( -55.14955436395487709, 214.8429017333601792, -4.673758765035196383 ) ) ;
#22065=CARTESIAN_POINT ( 'NONE',  ( -42.27752896937850835, 214.3500491399821897, 7.303452534266821949 ) ) ;
#22103=CARTESIAN_POINT ( 'NONE',  ( -67.01711230271183695, 216.4690446883607535, -1.857196546604089393 ) ) ;
#22105=CARTESIAN_POINT ( 'NONE',  ( -53.95461230271185116, 208.6787018382582346, -4.469044688360757966 ) ) ;
#22109=CARTESIAN_POINT ( 'NONE',  ( -69.39955436395489130, 213.3788001182225003, -3.209657149897400252 ) ) ;
#22110=CARTESIAN_POINT ( 'NONE',  ( -62.47247103062156981, 205.6499508600178956, 7.303452534266880569 ) ) ;
#22115=CARTESIAN_POINT ( 'NONE',  ( -43.06919563604516554, 216.5000000000000000, -0.1155267958017906493 ) ) ;
#22124=CARTESIAN_POINT ( 'NONE',  ( -50.20163769728823411, 215.6869285224996986, -3.149950860017881382 ) ) ;
#22129=CARTESIAN_POINT ( 'NONE',  ( -60.69122103062155560, 208.3738570449993404, -6.530955311639226935 ) ) ;
#22156=CARTESIAN_POINT ( 'NONE',  ( -59.89955436395489841, 213.3788001182225003, -3.209657149897400252 ) ) ;
#22203=CARTESIAN_POINT ( 'NONE',  ( -46.82961230271182984, 212.3930949314663792, 8.469044688360751749 ) ) ;
#22206=CARTESIAN_POINT ( 'NONE',  ( -35.15252896937850124, 207.6499508600178387, -3.839350919129087547 ) ) ;
#22210=CARTESIAN_POINT ( 'NONE',  ( -38.52455436395488420, 205.1570982666397356, 4.673758765035198159 ) ) ;
#22244=CARTESIAN_POINT ( 'NONE',  ( -47.22544563604515844, 214.8429017333602360, 4.673758765035156415 ) ) ;
#22247=CARTESIAN_POINT ( 'NONE',  ( -40.50372103062156981, 214.5309553116392749, -1.090244570138262148 ) ) ;
#22248=CARTESIAN_POINT ( 'NONE',  ( -53.56622103062157692, 211.6261429550005744, 6.530955311639227823 ) ) ;
#22252=CARTESIAN_POINT ( 'NONE',  ( -34.36086230271182984, 214.1499508600178387, -7.418979330068641964 ) ) ;
#22270=CARTESIAN_POINT ( 'NONE',  ( -61.48288769728821990, 203.5309553116391612, -1.857196546604028775 ) ) ;
#22287=CARTESIAN_POINT ( 'NONE',  ( -65.82961230271182274, 211.8571965466040581, 6.469044688360755302 ) ) ;
#22289=CARTESIAN_POINT ( 'NONE',  ( -57.71502896937850835, 213.8393509191290889, -2.350049139982142155 ) ) ;
#22293=CARTESIAN_POINT ( 'NONE',  ( -69.20163769728823411, 213.9548777149308592, -2.149950860017830756 ) ) ;
#22294=CARTESIAN_POINT ( 'NONE',  ( -62.86830436395490551, 209.8844732041983150, 8.500000000000003553 ) ) ;
#22299=CARTESIAN_POINT ( 'NONE',  ( -34.36086230271183695, 213.1499508600178387, -5.686928522499747451 ) ) ;
#22307=CARTESIAN_POINT ( 'NONE',  ( -43.47247103062156981, 206.6499508600178672, 5.571401726697986057 ) ) ;
#22311=CARTESIAN_POINT ( 'NONE',  ( -57.52455436395488420, 205.1570982666397356, 4.673758765035198159 ) ) ;
#22336=CARTESIAN_POINT ( 'NONE',  ( -62.67038769728824121, 208.6787018382581778, 4.469044688360752637 ) ) ;
#22385=CARTESIAN_POINT ( 'NONE',  ( -39.90252896937850124, 205.6499508600178103, -7.303452534266820173 ) ) ;
#22388=CARTESIAN_POINT ( 'NONE',  ( -37.92336230271182984, 213.9548777149308023, 2.149950860017852960 ) ) ;
#22393=CARTESIAN_POINT ( 'NONE',  ( -46.83705436395489841, 205.3262412349647263, -4.842901733360204020 ) ) ;
#22423=CARTESIAN_POINT ( 'NONE',  ( -31.19419563604516910, 203.5000000000000000, 0.1155267958017914542 ) ) ;
#22424=CARTESIAN_POINT ( 'NONE',  ( -47.81919563604517265, 216.5000000000000000, -0.1155267958017906493 ) ) ;
#22430=CARTESIAN_POINT ( 'NONE',  ( -40.10788769728823411, 214.4690446883608104, 1.321298161741840893 ) ) ;
#22431=CARTESIAN_POINT ( 'NONE',  ( -50.20163769728823411, 215.6869285224996986, -3.149950860017881382 ) ) ;
#22435=CARTESIAN_POINT ( 'NONE',  ( -67.22247103062156270, 205.6499508600178956, 7.303452534266880569 ) ) ;
#22454=CARTESIAN_POINT ( 'NONE',  ( -67.22247103062156270, 206.6499508600178672, 5.571401726697986057 ) ) ;
#22472=CARTESIAN_POINT ( 'NONE',  ( -60.68377896937849414, 208.3738570449995109, 6.530955311639247363 ) ) ;
#22475=CARTESIAN_POINT ( 'NONE',  ( -46.82961230271182984, 211.3212981617417938, 4.469044688360757966 ) ) ;
#22480=CARTESIAN_POINT ( 'NONE',  ( -38.52455436395488420, 205.1570982666397356, 4.673758765035198159 ) ) ;
#22481=CARTESIAN_POINT ( 'NONE',  ( -50.79538769728824121, 212.3930949314662371, -8.469044688360781947 ) ) ;
#22488=CARTESIAN_POINT ( 'NONE',  ( -66.62127896937849414, 218.5309553116392465, 2.162041339862725842 ) ) ;
#22495=CARTESIAN_POINT ( 'NONE',  ( -45.84747103062156981, 213.3500491399821328, -5.571401726697985168 ) ) ;
#22499=CARTESIAN_POINT ( 'NONE',  ( -67.22247103062156270, 206.6499508600178672, 5.571401726697986057 ) ) ;
#22524=CARTESIAN_POINT ( 'NONE',  ( -37.73288769728823411, 205.5309553116392465, -1.321298161741839117 ) ) ;
#22527=CARTESIAN_POINT ( 'NONE',  ( -69.59747103062156270, 213.3500491399821328, -5.571401726697985168 ) ) ;
#22571=CARTESIAN_POINT ( 'NONE',  ( -47.02752896937850835, 214.3500491399821897, 7.303452534266821949 ) ) ;
#22574=CARTESIAN_POINT ( 'NONE',  ( -38.71502896937850124, 213.8393509191290889, -2.350049139982142155 ) ) ;
#22578=CARTESIAN_POINT ( 'NONE',  ( -48.61830436395490551, 209.8844732041982581, 6.500000000000000888 ) ) ;
#22612=CARTESIAN_POINT ( 'NONE',  ( -45.84002896937850124, 204.4285982733020433, 3.350049139982171020 ) ) ;
#22617=CARTESIAN_POINT ( 'NONE',  ( -35.15997103062156270, 213.8393509191290889, 2.350049139982164359 ) ) ;
#22618=CARTESIAN_POINT ( 'NONE',  ( -41.09747103062156981, 213.3500491399821328, -5.571401726697985168 ) ) ;
#22623=CARTESIAN_POINT ( 'NONE',  ( -32.57961230271184405, 212.3930949314663792, 8.469044688360751749 ) ) ;
#22664=CARTESIAN_POINT ( 'NONE',  ( -58.50669563604516554, 209.8844732041982013, -6.500000000000000888 ) ) ;
#22666=CARTESIAN_POINT ( 'NONE',  ( -36.34002896937849414, 206.1606490808709111, 2.350049139982143931 ) ) ;
#22669=CARTESIAN_POINT ( 'NONE',  ( -31.99330436395490196, 210.1155267958017134, -6.500000000000000888 ) ) ;
#22670=CARTESIAN_POINT ( 'NONE',  ( -46.44122103062156981, 207.8379586601371329, -8.530955311639223382 ) ) ;
#22674=CARTESIAN_POINT ( 'NONE',  ( -33.37127896937850124, 216.5309553116391612, 1.626142955000506873 ) ) ;
#22688=CARTESIAN_POINT ( 'NONE',  ( -67.42038769728823411, 208.1428034533959703, 6.469044688360770401 ) ) ;
#22715=CARTESIAN_POINT ( 'NONE',  ( -46.44122103062156981, 208.9097554298617752, -4.530955311639240257 ) ) ;
#22756=CARTESIAN_POINT ( 'NONE',  ( -45.24627896937850835, 201.4690446883607251, -2.162041339862721845 ) ) ;
#22759=CARTESIAN_POINT ( 'NONE',  ( -62.66294563604517975, 214.6737587650350747, -4.842901733360249317 ) ) ;
#22762=CIRCLE ( 'NONE', #3379, 1.000000000000002220 ) ;
#22763=CARTESIAN_POINT ( 'NONE',  ( -49.01413769728823411, 213.1499508600178672, 5.686928522499718142 ) ) ;
#22794=CARTESIAN_POINT ( 'NONE',  ( -39.50669563604517265, 209.8844732041982013, -6.500000000000000888 ) ) ;
#22798=CARTESIAN_POINT ( 'NONE',  ( -68.00669563604516554, 209.8844732041982297, -4.499999999999996447 ) ) ;
#22799=CARTESIAN_POINT ( 'NONE',  ( -50.00372103062157692, 216.5309553116391612, -1.626142955000564383 ) ) ;
#22806=CARTESIAN_POINT ( 'NONE',  ( -33.56919563604517265, 218.5000000000000000, -0.1155267958018185298 ) ) ;
#22845=CARTESIAN_POINT ( 'NONE',  ( -65.03794563604516554, 205.3262412349648116, 4.842901733360249317 ) ) ;
#22847=CARTESIAN_POINT ( 'NONE',  ( -44.05877896937850124, 211.0902445701383101, -4.530955311639234040 ) ) ;
#22851=CARTESIAN_POINT ( 'NONE',  ( -33.18080436395490551, 203.5000000000000000, -0.1155267958017335561 ) ) ;
#22852=CARTESIAN_POINT ( 'NONE',  ( -44.26413769728823411, 214.1499508600179240, 7.418979330068584233 ) ) ;
#22856=CARTESIAN_POINT ( 'NONE',  ( -38.12127896937848703, 216.5309553116391612, 1.626142955000506873 ) ) ;
#22867=CARTESIAN_POINT ( 'NONE',  ( -56.73288769728823411, 203.5309553116391612, -1.857196546604028775 ) ) ;
#22894=CARTESIAN_POINT ( 'NONE',  ( -50.20163769728823411, 213.9548777149308592, -2.149950860017830756 ) ) ;
#22949=CARTESIAN_POINT ( 'NONE',  ( -49.40997103062156981, 215.5714017266979852, 3.350049139982118618 ) ) ;
#22980=CARTESIAN_POINT ( 'NONE',  ( -37.13169563604516554, 210.1155267958017703, 6.500000000000000888 ) ) ;
#22983=CARTESIAN_POINT ( 'NONE',  ( -55.73586230271182984, 207.8500491399821613, 3.954877714930852495 ) ) ;
#22984=CARTESIAN_POINT ( 'NONE',  ( -40.30580436395489841, 216.5000000000000000, 0.1155267958017343610 ) ) ;
#22990=CARTESIAN_POINT ( 'NONE',  ( -36.34002896937849414, 202.6965474657332038, 4.350049139982197666 ) ) ;
#23006=CARTESIAN_POINT ( 'NONE',  ( -52.97247103062156981, 206.6499508600178672, 5.571401726697986057 ) ) ;
#23019=AXIS2_PLACEMENT_3D ( 'NONE', #37014, #27931, #16940 ) ;
#23026=CARTESIAN_POINT ( 'NONE',  ( -54.54836230271182984, 204.3130714775002446, -3.149950860017828091 ) ) ;
#23028=CARTESIAN_POINT ( 'NONE',  ( -36.73586230271183695, 207.8500491399821613, 3.954877714930852495 ) ) ;
#23033=CARTESIAN_POINT ( 'NONE',  ( -63.85788769728821990, 214.4690446883608104, 1.321298161741840893 ) ) ;
#23034=CARTESIAN_POINT ( 'NONE',  ( -42.08705436395490551, 203.8621396198270475, -6.307003348497942419 ) ) ;
#23039=CARTESIAN_POINT ( 'NONE',  ( -36.73586230271183695, 206.8500491399821328, 5.686928522499748340 ) ) ;
#23051=CARTESIAN_POINT ( 'NONE',  ( -47.43080436395489841, 203.5000000000000000, -0.1155267958017335561 ) ) ;
#23075=CARTESIAN_POINT ( 'NONE',  ( -43.07663769728824121, 206.0451222850691408, 2.149950860017832532 ) ) ;
#23080=CARTESIAN_POINT ( 'NONE',  ( -67.42038769728823411, 208.1428034533959703, 6.469044688360770401 ) ) ;
#23133=CARTESIAN_POINT ( 'NONE',  ( -69.79538769728823411, 211.3212981617418222, -4.469044688360751749 ) ) ;
#23167=CARTESIAN_POINT ( 'NONE',  ( -67.41294563604516554, 216.1378603801729241, -6.307003348498026796 ) ) ;
#23170=CARTESIAN_POINT ( 'NONE',  ( -61.27752896937849414, 212.3500491399821613, 3.839350919129088435 ) ) ;
#23171=CARTESIAN_POINT ( 'NONE',  ( -45.25372103062155560, 216.5309553116391612, -1.626142955000564383 ) ) ;
#23176=CARTESIAN_POINT ( 'NONE',  ( -64.45163769728823411, 217.4189793300686233, -4.149950860017907139 ) ) ;
#23182=CARTESIAN_POINT ( 'NONE',  ( -38.12872103062155560, 203.4690446883607535, 1.626142955000567936 ) ) ;
#23194=CARTESIAN_POINT ( 'NONE',  ( -58.90997103062156270, 215.5714017266979852, 3.350049139982118618 ) ) ;
#23211=CARTESIAN_POINT ( 'NONE',  ( -49.00669563604516554, 209.8844732041982013, -6.500000000000000888 ) ) ;
#23214=CARTESIAN_POINT ( 'NONE',  ( -41.68377896937850124, 208.9097554298617183, 4.530955311639234040 ) ) ;
#23218=CARTESIAN_POINT ( 'NONE',  ( -65.24330436395489130, 210.1155267958017703, -4.499999999999996447 ) ) ;
#23219=CARTESIAN_POINT ( 'NONE',  ( -39.31622103062156981, 212.1620413398628671, 8.530955311639223382 ) ) ;
#23223=CARTESIAN_POINT ( 'NONE',  ( -59.29836230271182984, 202.5810206699313767, -4.149950860017804111 ) ) ;
#23234=CARTESIAN_POINT ( 'NONE',  ( -53.96205436395489130, 214.6737587650352168, 4.842901733360204908 ) ) ;
#23262=CARTESIAN_POINT ( 'NONE',  ( -46.04538769728823411, 211.3212981617418222, -4.469044688360751749 ) ) ;
#23266=CARTESIAN_POINT ( 'NONE',  ( -59.89955436395490551, 214.8429017333601792, -4.673758765035196383 ) ) ;
#23270=STYLED_ITEM('',(#37542),#8321);
#23315=CARTESIAN_POINT ( 'NONE',  ( -69.39955436395489130, 213.3788001182225003, -3.209657149897400252 ) ) ;
#23349=CARTESIAN_POINT ( 'NONE',  ( -31.78794563604516554, 205.3262412349647832, 4.842901733360250205 ) ) ;
#23352=CARTESIAN_POINT ( 'NONE',  ( -55.53794563604517975, 206.7903428501025758, 3.378800118222471838 ) ) ;
#23353=CARTESIAN_POINT ( 'NONE',  ( -37.33705436395490551, 205.3262412349647263, -4.842901733360204020 ) ) ;
#23358=CARTESIAN_POINT ( 'NONE',  ( -60.88913769728824121, 205.8500491399820760, -7.418979330068584233 ) ) ;
#23364=ORIENTED_EDGE ( 'NONE', *, *, #15916, .T. ) ;
#23365=CARTESIAN_POINT ( 'NONE',  ( -45.25372103062156270, 216.5309553116392181, -1.626142955000564383 ) ) ;
#23378=CARTESIAN_POINT ( 'NONE',  ( -57.52455436395488420, 205.1570982666397356, 4.673758765035198159 ) ) ;
#23395=CARTESIAN_POINT ( 'NONE',  ( -49.40252896937850124, 206.6499508600178387, -5.571401726697954970 ) ) ;
#23397=CARTESIAN_POINT ( 'NONE',  ( -67.21502896937850835, 215.5714017266979567, -3.350049139982168800 ) ) ;
#23400=CARTESIAN_POINT ( 'NONE',  ( -54.75372103062156270, 214.5309553116392749, -1.090244570138262148 ) ) ;
#23401=CARTESIAN_POINT ( 'NONE',  ( -33.57663769728823411, 202.5810206699313767, 4.149950860017909804 ) ) ;
#23405=CARTESIAN_POINT ( 'NONE',  ( -61.47544563604516554, 216.3070033484980854, 6.137860380172893926 ) ) ;
#23416=CARTESIAN_POINT ( 'NONE',  ( -46.24330436395489841, 210.1155267958017134, -6.500000000000000888 ) ) ;
#23441=CARTESIAN_POINT ( 'NONE',  ( -65.82961230271185116, 211.3212981617417938, 4.469044688360757966 ) ) ;
#23446=CARTESIAN_POINT ( 'NONE',  ( -64.84747103062156270, 213.3500491399821328, -5.571401726697985168 ) ) ;
#23447=CARTESIAN_POINT ( 'NONE',  ( -45.64211230271183695, 201.5309553116392181, 2.393094931466368980 ) ) ;
#23452=CARTESIAN_POINT ( 'NONE',  ( -53.16294563604517265, 214.6737587650350747, -4.842901733360249317 ) ) ;
#23460=CARTESIAN_POINT ( 'NONE',  ( -66.03497103062157692, 204.4285982733020148, -3.350049139982115509 ) ) ;
#23499=CARTESIAN_POINT ( 'NONE',  ( -65.63913769728821990, 207.8500491399821613, -3.954877714930864485 ) ) ;
#23538=CARTESIAN_POINT ( 'NONE',  ( -32.38169563604517265, 210.1155267958017703, 6.500000000000000888 ) ) ;
#23542=CARTESIAN_POINT ( 'NONE',  ( -61.87127896937851546, 214.5309553116392749, 1.090244570138288127 ) ) ;
#23548=CARTESIAN_POINT ( 'NONE',  ( -56.13913769728823411, 205.8500491399820760, -7.418979330068584233 ) ) ;
#23555=CARTESIAN_POINT ( 'NONE',  ( -38.72247103062156981, 206.6499508600178672, 5.571401726697986057 ) ) ;
#23567=CARTESIAN_POINT ( 'NONE',  ( -52.18080436395490551, 203.5000000000000000, -0.1155267958017335561 ) ) ;
#23583=CARTESIAN_POINT ( 'NONE',  ( -45.84002896937850124, 204.4285982733020433, 3.350049139982171020 ) ) ;
#23585=CARTESIAN_POINT ( 'NONE',  ( -67.61086230271183695, 213.1499508600178387, -5.686928522499747451 ) ) ;
#23588=CARTESIAN_POINT ( 'NONE',  ( -57.12872103062156270, 205.4690446883607535, 1.090244570138264368 ) ) ;
#23589=CARTESIAN_POINT ( 'NONE',  ( -66.43080436395490551, 203.5000000000000000, -0.1155267958017335561 ) ) ;
#23593=CARTESIAN_POINT ( 'NONE',  ( -63.85044563604516554, 203.6929966515019430, -6.137860380172892150 ) ) ;
#23603=CARTESIAN_POINT ( 'NONE',  ( -50.00372103062157692, 216.5309553116391612, -1.626142955000564383 ) ) ;
#23634=CARTESIAN_POINT ( 'NONE',  ( -66.42336230271182274, 213.9548777149308023, 2.149950860017852960 ) ) ;
#23638=CARTESIAN_POINT ( 'NONE',  ( -63.06622103062156981, 211.6261429550005744, 6.530955311639227823 ) ) ;
#23639=CARTESIAN_POINT ( 'NONE',  ( -30.00669563604516554, 209.8844732041981729, -8.500000000000003553 ) ) ;
#23645=CARTESIAN_POINT ( 'NONE',  ( -51.97544563604516554, 214.8429017333602360, 4.673758765035156415 ) ) ;
#23687=CARTESIAN_POINT ( 'NONE',  ( -34.96205436395488420, 214.6737587650352168, 4.842901733360204908 ) ) ;
#23728=CARTESIAN_POINT ( 'NONE',  ( -65.23586230271183695, 205.8500491399821613, 7.418979330068642852 ) ) ;
#23731=CARTESIAN_POINT ( 'NONE',  ( -63.05877896937850835, 211.0902445701383101, -4.530955311639234040 ) ) ;
#23736=CARTESIAN_POINT ( 'NONE',  ( -65.24330436395489130, 210.1155267958016850, -8.500000000000003553 ) ) ;
#23743=CARTESIAN_POINT ( 'NONE',  ( -34.56622103062156270, 211.6261429550005744, 6.530955311639228711 ) ) ;
#23771=CARTESIAN_POINT ( 'NONE',  ( -34.36086230271183695, 213.1499508600178387, -5.686928522499747451 ) ) ;
#23773=CARTESIAN_POINT ( 'NONE',  ( -34.36086230271182984, 212.1499508600178387, -3.954877714930852495 ) ) ;
#23777=CARTESIAN_POINT ( 'NONE',  ( -58.31622103062156981, 211.0902445701382533, 4.530955311639240257 ) ) ;
#23779=CARTESIAN_POINT ( 'NONE',  ( -69.00372103062157692, 216.5309553116391612, -1.626142955000564383 ) ) ;
#23783=CARTESIAN_POINT ( 'NONE',  ( -53.36086230271183695, 214.1499508600178387, -7.418979330068641964 ) ) ;
#23793=CARTESIAN_POINT ( 'NONE',  ( -54.35788769728821279, 216.4690446883607535, 1.857196546604031662 ) ) ;
#23820=CARTESIAN_POINT ( 'NONE',  ( -65.63169563604516554, 210.1155267958017703, 4.499999999999996447 ) ) ;
#23824=CARTESIAN_POINT ( 'NONE',  ( -62.07663769728823411, 204.3130714775002730, 3.149950860017883603 ) ) ;
#23825=CARTESIAN_POINT ( 'NONE',  ( -33.37127896937850124, 218.5309553116392465, 2.162041339862725842 ) ) ;
#23831=CARTESIAN_POINT ( 'NONE',  ( -58.30877896937847993, 211.6261429550004607, -6.530955311639245586 ) ) ;
#23840=CARTESIAN_POINT ( 'NONE',  ( -64.05580436395490551, 216.5000000000000000, 0.1155267958017343610 ) ) ;
#23881=CARTESIAN_POINT ( 'NONE',  ( -66.03497103062157692, 206.1606490808709111, -2.350049139982163027 ) ) ;
#23894=ORIENTED_EDGE ( 'NONE', *, *, #21219, .T. ) ;
#23918=CARTESIAN_POINT ( 'NONE',  ( -35.35044563604516554, 205.1570982666397072, -4.673758765035155527 ) ) ;
#23922=CARTESIAN_POINT ( 'NONE',  ( -40.29836230271183695, 206.0451222850691977, -2.149950860017851184 ) ) ;
#23923=CARTESIAN_POINT ( 'NONE',  ( -32.78497103062156981, 204.4285982733020148, -3.350049139982115509 ) ) ;
#23928=CARTESIAN_POINT ( 'NONE',  ( -48.61830436395490551, 209.8844732041983150, 8.500000000000003553 ) ) ;
#23961=CARTESIAN_POINT ( 'NONE',  ( -32.97544563604516554, 214.8429017333602360, 4.673758765035156415 ) ) ;
#23963=CARTESIAN_POINT ( 'NONE',  ( -62.86086230271182984, 213.1499508600178387, -5.686928522499747451 ) ) ;
#23967=CARTESIAN_POINT ( 'NONE',  ( -47.62872103062157692, 205.4690446883607535, 1.090244570138264368 ) ) ;
#23968=CARTESIAN_POINT ( 'NONE',  ( -34.17038769728823411, 207.6069050685337913, 8.469044688360781947 ) ) ;
#23973=CARTESIAN_POINT ( 'NONE',  ( -55.34002896937850124, 202.6965474657332038, 4.350049139982197666 ) ) ;
#23974=DIRECTION ( 'NONE',  ( 0.9933043639548628789, -0.1155267958017759528, 0.000000000000000000 ) ) ;
#23985=CARTESIAN_POINT ( 'NONE',  ( -37.33705436395490551, 205.3262412349647263, -4.842901733360204020 ) ) ;
#24012=CARTESIAN_POINT ( 'NONE',  ( -64.84002896937849414, 206.1606490808709111, 2.350049139982143931 ) ) ;
#24016=CARTESIAN_POINT ( 'NONE',  ( -62.47247103062156981, 206.6499508600178672, 5.571401726697986057 ) ) ;
#24017=CARTESIAN_POINT ( 'NONE',  ( -67.22247103062156270, 205.6499508600178956, 7.303452534266880569 ) ) ;
#24021=CARTESIAN_POINT ( 'NONE',  ( -60.28794563604516554, 205.3262412349647832, 4.842901733360250205 ) ) ;
#24033=CARTESIAN_POINT ( 'NONE',  ( -42.87872103062157692, 201.4690446883607819, 2.162041339862843525 ) ) ;
#24106=CARTESIAN_POINT ( 'NONE',  ( -49.99627896937850835, 201.4690446883607251, -2.162041339862721845 ) ) ;
#24110=CARTESIAN_POINT ( 'NONE',  ( -45.24627896937850835, 205.4690446883607535, -1.090244570138286351 ) ) ;
#24117=CARTESIAN_POINT ( 'NONE',  ( -45.05580436395490551, 218.5000000000000000, 0.1155267958017064944 ) ) ;
#24147=CARTESIAN_POINT ( 'NONE',  ( -36.34002896937850124, 204.4285982733020433, 3.350049139982171020 ) ) ;
#24148=CARTESIAN_POINT ( 'NONE',  ( -67.01711230271183695, 216.4690446883607535, -1.857196546604089393 ) ) ;
#24151=CARTESIAN_POINT ( 'NONE',  ( -52.37872103062156981, 205.4690446883607535, 1.090244570138264368 ) ) ;
#24152=CARTESIAN_POINT ( 'NONE',  ( -36.54538769728824121, 212.3930949314662371, -8.469044688360781947 ) ) ;
#24156=CARTESIAN_POINT ( 'NONE',  ( -40.10044563604517265, 203.6929966515019430, -6.137860380172892150 ) ) ;
#24167=CARTESIAN_POINT ( 'NONE',  ( -33.97247103062156270, 206.6499508600178672, 5.571401726697986057 ) ) ;
#24195=CARTESIAN_POINT ( 'NONE',  ( -35.95163769728824121, 213.9548777149308592, -2.149950860017830756 ) ) ;
#24199=CARTESIAN_POINT ( 'NONE',  ( -49.40997103062156981, 215.5714017266979852, 3.350049139982118618 ) ) ;
#24200=CARTESIAN_POINT ( 'NONE',  ( -65.83705436395491972, 203.8621396198270475, -6.307003348497942419 ) ) ;
#24205=CARTESIAN_POINT ( 'NONE',  ( -40.10044563604517265, 205.1570982666397072, -4.673758765035155527 ) ) ;
#24213=CARTESIAN_POINT ( 'NONE',  ( -56.93080436395490551, 203.5000000000000000, -0.1155267958017335561 ) ) ;
#24217=CARTESIAN_POINT ( 'NONE',  ( -39.31622103062156981, 212.1620413398628671, 8.530955311639223382 ) ) ;
#24295=CARTESIAN_POINT ( 'NONE',  ( -50.98586230271183695, 205.8500491399821613, 7.418979330068642852 ) ) ;
#24298=CARTESIAN_POINT ( 'NONE',  ( -45.84002896937850124, 206.1606490808709111, 2.350049139982143931 ) ) ;
#24304=CARTESIAN_POINT ( 'NONE',  ( -47.03497103062157692, 202.6965474657331185, -4.350049139982091084 ) ) ;
#24311=CARTESIAN_POINT ( 'NONE',  ( -33.18080436395490551, 203.5000000000000000, -0.1155267958017335561 ) ) ;
#24336=CARTESIAN_POINT ( 'NONE',  ( -41.88169563604517265, 210.1155267958017703, 6.500000000000000888 ) ) ;
#24337=CARTESIAN_POINT ( 'NONE',  ( -53.75669563604516554, 209.8844732041982013, -6.500000000000000888 ) ) ;
#24341=CARTESIAN_POINT ( 'NONE',  ( -42.28497103062156270, 206.1606490808709111, -2.350049139982163027 ) ) ;
#24342=CARTESIAN_POINT ( 'NONE',  ( -56.13913769728823411, 206.8500491399821044, -5.686928522499717253 ) ) ;
#24346=CARTESIAN_POINT ( 'NONE',  ( -43.26711230271184405, 218.4690446883607535, -2.393094931466363651 ) ) ;
#24358=CARTESIAN_POINT ( 'NONE',  ( -35.75372103062156981, 216.5309553116391612, -1.626142955000564383 ) ) ;
#24383=CARTESIAN_POINT ( 'NONE',  ( -50.19419563604517975, 205.4999999999999716, 0.1155267958017633378 ) ) ;
#24387=CARTESIAN_POINT ( 'NONE',  ( -50.39955436395490551, 214.8429017333601792, -4.673758765035196383 ) ) ;
#24388=CARTESIAN_POINT ( 'NONE',  ( -63.85788769728821990, 218.4690446883607535, 2.393094931466250408 ) ) ;
#24392=CARTESIAN_POINT ( 'NONE',  ( -48.41294563604515133, 214.6737587650350747, -4.842901733360249317 ) ) ;
#24400=CARTESIAN_POINT ( 'NONE',  ( -61.48288769728822700, 203.5309553116391896, -1.857196546604028997 ) ) ;
#24404=CARTESIAN_POINT ( 'NONE',  ( -36.34747103062156981, 214.3500491399821044, -7.303452534266878793 ) ) ;
#24471=AXIS2_PLACEMENT_3D ( 'NONE', #30545, #27871, #1903 ) ;
#24479=CARTESIAN_POINT ( 'NONE',  ( -50.78794563604517975, 203.8621396198271043, 6.307003348498029460 ) ) ;
#24483=CARTESIAN_POINT ( 'NONE',  ( -49.60044563604517265, 206.6211998817775566, -3.209657149897419348 ) ) ;
#24490=CARTESIAN_POINT ( 'NONE',  ( -52.37872103062156981, 201.4690446883607819, 2.162041339862843525 ) ) ;
#24517=CARTESIAN_POINT ( 'NONE',  ( -42.27752896937850124, 213.3500491399821613, 5.571401726697954970 ) ) ;
#24518=CARTESIAN_POINT ( 'NONE',  ( -58.50669563604516554, 209.8844732041982013, -6.500000000000000888 ) ) ;
#24522=CARTESIAN_POINT ( 'NONE',  ( -46.44122103062156981, 208.9097554298617752, -4.530955311639240257 ) ) ;
#24523=CARTESIAN_POINT ( 'NONE',  ( -59.70163769728823411, 215.6869285224996986, -3.149950860017881382 ) ) ;
#24527=CARTESIAN_POINT ( 'NONE',  ( -43.46502896937849414, 217.3034525342667962, -4.350049139982195001 ) ) ;
#24538=CARTESIAN_POINT ( 'NONE',  ( -42.68080436395489841, 203.5000000000000000, -0.1155267958017335561 ) ) ;
#24565=CARTESIAN_POINT ( 'NONE',  ( -49.99627896937850835, 205.4690446883607535, -1.090244570138286351 ) ) ;
#24568=CARTESIAN_POINT ( 'NONE',  ( -48.22247103062156270, 206.6499508600178672, 5.571401726697986057 ) ) ;
#24569=CARTESIAN_POINT ( 'NONE',  ( -61.48288769728824121, 201.5309553116392181, -2.393094931466246855 ) ) ;
#24576=CARTESIAN_POINT ( 'NONE',  ( -50.78794563604515133, 205.3262412349647832, 4.842901733360250205 ) ) ;
#24583=CARTESIAN_POINT ( 'NONE',  ( -60.88913769728823411, 206.8500491399821044, -5.686928522499717253 ) ) ;
#24587=CARTESIAN_POINT ( 'NONE',  ( -38.32663769728823411, 202.5810206699313767, 4.149950860017909804 ) ) ;
#24597=CARTESIAN_POINT ( 'NONE',  ( -66.62872103062152007, 203.4690446883607535, 1.626142955000567936 ) ) ;
#24612=CARTESIAN_POINT ( 'NONE',  ( -57.32663769728824121, 206.0451222850691408, 2.149950860017832532 ) ) ;
#24657=ADVANCED_FACE ( 'NONE', ( #566 ), #14986, .F. ) ;
#24658=CARTESIAN_POINT ( 'NONE',  ( -51.57961230271184405, 212.3930949314663792, 8.469044688360751749 ) ) ;
#24661=CARTESIAN_POINT ( 'NONE',  ( -42.87127896937849414, 214.5309553116392749, 1.090244570138288127 ) ) ;
#24668=CARTESIAN_POINT ( 'NONE',  ( -51.58705436395489841, 203.8621396198270475, -6.307003348497942419 ) ) ;
#24698=CARTESIAN_POINT ( 'NONE',  ( -57.51711230271181563, 216.4690446883607535, -1.857196546604089393 ) ) ;
#24702=CARTESIAN_POINT ( 'NONE',  ( -44.65997103062156981, 213.8393509191290889, 2.350049139982164359 ) ) ;
#24703=CARTESIAN_POINT ( 'NONE',  ( -63.46205436395489841, 214.6737587650352168, 4.842901733360204908 ) ) ;
#24708=CARTESIAN_POINT ( 'NONE',  ( -51.18377896937850835, 207.8379586601372750, 8.530955311639258909 ) ) ;
#24719=CARTESIAN_POINT ( 'NONE',  ( -42.28497103062156270, 204.4285982733020148, -3.350049139982115509 ) ) ;
#24748=CARTESIAN_POINT ( 'NONE',  ( -51.77752896937850124, 212.3500491399821613, 3.839350919129088435 ) ) ;
#24752=CARTESIAN_POINT ( 'NONE',  ( -49.80580436395490551, 216.5000000000000000, 0.1155267958017343610 ) ) ;
#24753=CARTESIAN_POINT ( 'NONE',  ( -51.19122103062157692, 207.8379586601371329, -8.530955311639223382 ) ) ;
#24757=CARTESIAN_POINT ( 'NONE',  ( -48.21502896937850124, 215.5714017266979567, -3.350049139982168800 ) ) ;
#24765=CARTESIAN_POINT ( 'NONE',  ( -51.78497103062156981, 204.4285982733020148, -3.350049139982115509 ) ) ;
#24771=CARTESIAN_POINT ( 'NONE',  ( -42.08705436395490551, 203.8621396198270475, -6.307003348497942419 ) ) ;
#24796=CARTESIAN_POINT ( 'NONE',  ( -61.87872103062156981, 205.4690446883607535, 1.090244570138264368 ) ) ;
#24844=CARTESIAN_POINT ( 'NONE',  ( -52.96502896937850124, 217.3034525342667962, -4.350049139982195001 ) ) ;
#24848=CARTESIAN_POINT ( 'NONE',  ( -36.93377896937849414, 208.9097554298617183, 4.530955311639234040 ) ) ;
#24885=CARTESIAN_POINT ( 'NONE',  ( -30.99627896937850480, 203.4690446883607535, -1.626142955000504209 ) ) ;
#24886=CARTESIAN_POINT ( 'NONE',  ( -55.53794563604516554, 205.3262412349647832, 4.842901733360250205 ) ) ;
#24890=CARTESIAN_POINT ( 'NONE',  ( -39.71205436395491262, 213.2096571498974242, 3.378800118222489601 ) ) ;
#24891=CARTESIAN_POINT ( 'NONE',  ( -55.54538769728823411, 211.8571965466039444, -6.469044688360768625 ) ) ;
#24896=CARTESIAN_POINT ( 'NONE',  ( -44.65252896937850835, 205.6499508600178103, -7.303452534266820173 ) ) ;
#24930=CARTESIAN_POINT ( 'NONE',  ( -63.85044563604516554, 205.1570982666397072, -4.673758765035155527 ) ) ;
#24932=CARTESIAN_POINT ( 'NONE',  ( -55.14211230271182984, 205.5309553116392465, 1.321298161741817356 ) ) ;
#24935=CARTESIAN_POINT ( 'NONE',  ( -44.85788769728821990, 216.4690446883607535, 1.857196546604031662 ) ) ;
#24936=CARTESIAN_POINT ( 'NONE',  ( -63.65997103062157692, 217.3034525342668815, 4.350049139982096413 ) ) ;
#24940=CARTESIAN_POINT ( 'NONE',  ( -46.23586230271182984, 206.8500491399821328, 5.686928522499748340 ) ) ;
#24947=CARTESIAN_POINT ( 'NONE',  ( -50.39955436395489841, 214.8429017333601792, -4.673758765035197271 ) ) ;
#24951=CARTESIAN_POINT ( 'NONE',  ( -61.48288769728821990, 203.5309553116391612, -1.857196546604028775 ) ) ;
#24974=CARTESIAN_POINT ( 'NONE',  ( -62.27455436395490551, 206.6211998817774997, 3.209657149897401585 ) ) ;
#24996=EDGE_CURVE ( 'NONE', #33325, #14550, #22762, .T. ) ;
#25026=CARTESIAN_POINT ( 'NONE',  ( -37.13169563604516554, 210.1155267958018271, 8.500000000000003553 ) ) ;
#25029=CARTESIAN_POINT ( 'NONE',  ( -34.16294563604517265, 213.2096571498974527, -3.378800118222469617 ) ) ;
#25068=CARTESIAN_POINT ( 'NONE',  ( -59.69419563604516554, 203.5000000000000000, 0.1155267958017914542 ) ) ;
#25071=PRODUCT_DEFINITION_FORMATION_WITH_SPECIFIED_SOURCE ( 'ANY', '', #17435, .NOT_KNOWN. ) ;
#25074=CARTESIAN_POINT ( 'NONE',  ( -37.93080436395490551, 205.4999999999999716, -0.1155267958017894420 ) ) ;
#25075=CARTESIAN_POINT ( 'NONE',  ( -59.30580436395489841, 216.5000000000000000, 0.1155267958017343610 ) ) ;
#25079=CARTESIAN_POINT ( 'NONE',  ( -69.59747103062156270, 214.3500491399821044, -7.303452534266878793 ) ) ;
#25092=DIRECTION ( 'NONE',  ( -0.9933043639548644332, 0.1155267958017622554, 0.000000000000000000 ) ) ;
#25117=CARTESIAN_POINT ( 'NONE',  ( -68.00669563604516554, 209.8844732041982013, -6.500000000000000888 ) ) ;
#25121=CARTESIAN_POINT ( 'NONE',  ( -52.76711230271184405, 214.4690446883608104, -1.321298161741814914 ) ) ;
#25124=CARTESIAN_POINT ( 'NONE',  ( -38.92038769728823411, 208.1428034533959703, 6.469044688360770401 ) ) ;
#25125=CARTESIAN_POINT ( 'NONE',  ( -57.72247103062156270, 205.6499508600178956, 7.303452534266880569 ) ) ;
#25130=CARTESIAN_POINT ( 'NONE',  ( -67.61086230271183695, 214.1499508600178387, -7.418979330068641964 ) ) ;
#25140=CARTESIAN_POINT ( 'NONE',  ( -45.64955436395490551, 214.8429017333601792, -4.673758765035197271 ) ) ;
#25144=CARTESIAN_POINT ( 'NONE',  ( -58.51413769728823411, 213.1499508600178672, 5.686928522499718142 ) ) ;
#25172=CARTESIAN_POINT ( 'NONE',  ( -54.55580436395489841, 214.5000000000000284, 0.1155267958017899832 ) ) ;
#25220=CARTESIAN_POINT ( 'NONE',  ( -39.30877896937850124, 212.1620413398627534, -8.530955311639255356 ) ) ;
#25223=CARTESIAN_POINT ( 'NONE',  ( -35.35044563604517265, 206.6211998817775566, -3.209657149897419348 ) ) ;
#25226=CARTESIAN_POINT ( 'NONE',  ( -45.84747103062156981, 213.3500491399821328, -5.571401726697985168 ) ) ;
#25260=CARTESIAN_POINT ( 'NONE',  ( -41.48586230271182984, 206.8500491399821328, 5.686928522499748340 ) ) ;
#25263=CARTESIAN_POINT ( 'NONE',  ( -37.73288769728823411, 205.5309553116392465, -1.321298161741839117 ) ) ;
#25264=CARTESIAN_POINT ( 'NONE',  ( -40.50372103062156981, 216.5309553116391612, -1.626142955000564383 ) ) ;
#25268=CARTESIAN_POINT ( 'NONE',  ( -67.81622103062157692, 212.1620413398628671, 8.530955311639223382 ) ) ;
#25287=CARTESIAN_POINT ( 'NONE',  ( -68.40997103062156270, 215.5714017266979852, 3.350049139982118618 ) ) ;
#25303=CARTESIAN_POINT ( 'NONE',  ( -66.42336230271182274, 215.6869285224997270, 3.149950860017831200 ) ) ;
#25305=CARTESIAN_POINT ( 'NONE',  ( -43.86086230271183695, 212.1499508600178387, -3.954877714930852495 ) ) ;
#25309=CARTESIAN_POINT ( 'NONE',  ( -67.42038769728826253, 208.6787018382581778, 4.469044688360752637 ) ) ;
#25310=CARTESIAN_POINT ( 'NONE',  ( -54.35788769728822700, 218.4690446883607535, 2.393094931466250408 ) ) ;
#25315=CARTESIAN_POINT ( 'NONE',  ( -33.76711230271183695, 216.4690446883607535, -1.857196546604089393 ) ) ;
#25325=CARTESIAN_POINT ( 'NONE',  ( -41.09747103062156981, 213.3500491399821328, -5.571401726697985168 ) ) ;
#25329=CARTESIAN_POINT ( 'NONE',  ( -67.81622103062156270, 211.6261429550005744, 6.530955311639227823 ) ) ;
#25356=CARTESIAN_POINT ( 'NONE',  ( -41.09747103062157692, 212.3500491399821613, -3.839350919129076445 ) ) ;
#25402=CARTESIAN_POINT ( 'NONE',  ( -43.66294563604516554, 216.1378603801729241, -6.307003348498026796 ) ) ;
#25405=CARTESIAN_POINT ( 'NONE',  ( -31.59002896937850124, 206.1606490808709111, 2.350049139982143931 ) ) ;
#25408=CARTESIAN_POINT ( 'NONE',  ( -40.70163769728823411, 215.6869285224996986, -3.149950860017881382 ) ) ;
#25441=CARTESIAN_POINT ( 'NONE',  ( -44.45461230271182274, 208.1428034533959135, -6.469044688360754414 ) ) ;
#25445=CARTESIAN_POINT ( 'NONE',  ( -37.13913769728823411, 207.8500491399821613, -3.954877714930864485 ) ) ;
#25446=CARTESIAN_POINT ( 'NONE',  ( -41.69122103062155560, 208.3738570449993404, -6.530955311639226935 ) ) ;
#25451=CARTESIAN_POINT ( 'NONE',  ( -38.71502896937850124, 217.3034525342667962, -4.350049139982195001 ) ) ;
#25488=CARTESIAN_POINT ( 'NONE',  ( -62.66294563604517975, 214.6737587650350747, -4.842901733360248429 ) ) ;
#25490=CARTESIAN_POINT ( 'NONE',  ( -38.31919563604515844, 214.5000000000000284, -0.1155267958017627827 ) ) ;
#25495=CARTESIAN_POINT ( 'NONE',  ( -34.36830436395490551, 209.8844732041982581, 6.500000000000000888 ) ) ;
#25496=CARTESIAN_POINT ( 'NONE',  ( -38.52455436395490551, 203.6929966515020283, 6.137860380172978303 ) ) ;
#25501=CARTESIAN_POINT ( 'NONE',  ( -37.32961230271182274, 211.8571965466040297, 6.469044688360755302 ) ) ;
#25512=CARTESIAN_POINT ( 'NONE',  ( -59.89955436395490551, 214.8429017333601792, -4.673758765035196383 ) ) ;
#25538=CARTESIAN_POINT ( 'NONE',  ( -48.81622103062156981, 211.0902445701382533, 4.530955311639240257 ) ) ;
#25585=CARTESIAN_POINT ( 'NONE',  ( -38.71502896937850124, 217.3034525342667962, -4.350049139982195001 ) ) ;
#25588=CARTESIAN_POINT ( 'NONE',  ( -67.21502896937850835, 215.5714017266979567, -3.350049139982168800 ) ) ;
#25591=CARTESIAN_POINT ( 'NONE',  ( -44.06622103062156981, 211.6261429550005744, 6.530955311639227823 ) ) ;
#25625=CARTESIAN_POINT ( 'NONE',  ( -43.46502896937849414, 215.5714017266979567, -3.350049139982168800 ) ) ;
#25628=CARTESIAN_POINT ( 'NONE',  ( -67.61086230271183695, 212.1499508600178387, -3.954877714930852495 ) ) ;
#25629=CARTESIAN_POINT ( 'NONE',  ( -39.11830436395489841, 209.8844732041982581, 6.500000000000000888 ) ) ;
#25635=CARTESIAN_POINT ( 'NONE',  ( -30.79836230271183339, 202.5810206699313767, -4.149950860017804111 ) ) ;
#25636=COLOUR_RGB ( '',0.8941176470588234615, 0.8941176470588234615, 0.8941176470588234615 ) ;
#25653=EDGE_LOOP ( 'NONE', ( #5708, #15569 ) ) ;
#25654=CARTESIAN_POINT ( 'NONE',  ( -64.05580436395490551, 216.5000000000000000, 0.1155267958017343610 ) ) ;
#25677=CARTESIAN_POINT ( 'NONE',  ( -66.22544563604516554, 214.8429017333602360, 4.673758765035156415 ) ) ;
#25679=CARTESIAN_POINT ( 'NONE',  ( -47.81919563604517265, 214.5000000000000284, -0.1155267958017627827 ) ) ;
#25683=CARTESIAN_POINT ( 'NONE',  ( -40.10788769728823411, 216.4690446883607535, 1.857196546604031662 ) ) ;
#25684=CARTESIAN_POINT ( 'NONE',  ( -47.43080436395489841, 201.5000000000000000, -0.1155267958017054536 ) ) ;
#25689=CARTESIAN_POINT ( 'NONE',  ( -32.18377896937850835, 208.3738570449995109, 6.530955311639247363 ) ) ;
#25699=CARTESIAN_POINT ( 'NONE',  ( -62.67038769728823411, 208.1428034533959703, 6.469044688360770401 ) ) ;
#25724=CARTESIAN_POINT ( 'NONE',  ( -46.83705436395489130, 206.7903428501026042, -3.378800118222489157 ) ) ;
#25771=CARTESIAN_POINT ( 'NONE',  ( -53.75669563604516554, 209.8844732041982013, -6.500000000000000888 ) ) ;
#25776=CARTESIAN_POINT ( 'NONE',  ( -40.10788769728823411, 216.4690446883607535, 1.857196546604031662 ) ) ;
#25811=CARTESIAN_POINT ( 'NONE',  ( -37.52752896937850124, 213.3500491399821613, 5.571401726697954970 ) ) ;
#25816=CARTESIAN_POINT ( 'NONE',  ( -62.46502896937850124, 213.8393509191290889, -2.350049139982142155 ) ) ;
#25817=CARTESIAN_POINT ( 'NONE',  ( -40.89955436395488420, 214.8429017333601792, -4.673758765035196383 ) ) ;
#25823=CARTESIAN_POINT ( 'NONE',  ( -38.31919563604515844, 218.5000000000000000, -0.1155267958018185298 ) ) ;
#25839=CARTESIAN_POINT ( 'NONE',  ( -50.39955436395490551, 214.8429017333601792, -4.673758765035196383 ) ) ;
#25859=CARTESIAN_POINT ( 'NONE',  ( -54.35044563604515844, 205.1570982666397072, -4.673758765035155527 ) ) ;
#25861=CARTESIAN_POINT ( 'NONE',  ( -39.50669563604516554, 209.8844732041982297, -4.499999999999996447 ) ) ;
#25865=CARTESIAN_POINT ( 'NONE',  ( -69.79538769728823411, 211.3212981617418222, -4.469044688360751749 ) ) ;
#25866=CARTESIAN_POINT ( 'NONE',  ( -44.85788769728823411, 218.4690446883607535, 2.393094931466250408 ) ) ;
#25871=CARTESIAN_POINT ( 'NONE',  ( -68.00669563604516554, 209.8844732041981729, -8.500000000000003553 ) ) ;
#25883=CARTESIAN_POINT ( 'NONE',  ( -51.19122103062155560, 208.3738570449993404, -6.530955311639226935 ) ) ;
#25911=CARTESIAN_POINT ( 'NONE',  ( -48.61830436395490551, 209.8844732041982297, 4.499999999999996447 ) ) ;
#25963=CARTESIAN_POINT ( 'NONE',  ( -38.72247103062156981, 206.6499508600178672, 5.571401726697986057 ) ) ;
#25997=CARTESIAN_POINT ( 'NONE',  ( -62.06919563604516554, 218.5000000000000000, -0.1155267958018185298 ) ) ;
#26001=CARTESIAN_POINT ( 'NONE',  ( -51.97544563604517265, 213.3788001182224718, 3.209657149897419348 ) ) ;
#26002=CARTESIAN_POINT ( 'NONE',  ( -44.65997103062156981, 215.5714017266979852, 3.350049139982118618 ) ) ;
#26008=CARTESIAN_POINT ( 'NONE',  ( -59.89955436395489841, 216.3070033484980002, -6.137860380172975638 ) ) ;
#26013=CARTESIAN_POINT ( 'NONE',  ( -42.28497103062156270, 204.4285982733020148, -3.350049139982115509 ) ) ;
#26024=CARTESIAN_POINT ( 'NONE',  ( -57.72247103062156270, 206.6499508600178672, 5.571401726697986057 ) ) ;
#26045=CARTESIAN_POINT ( 'NONE',  ( -51.57961230271182984, 211.8571965466040581, 6.469044688360755302 ) ) ;
#26047=CARTESIAN_POINT ( 'NONE',  ( -44.65252896937850835, 207.6499508600178387, -3.839350919129087547 ) ) ;
#26050=CARTESIAN_POINT ( 'NONE',  ( -54.15997103062156981, 213.8393509191290889, 2.350049139982164359 ) ) ;
#26051=CARTESIAN_POINT ( 'NONE',  ( -40.10788769728823411, 218.4690446883607535, 2.393094931466250408 ) ) ;
#26055=CARTESIAN_POINT ( 'NONE',  ( -54.15252896937849414, 205.6499508600178103, -7.303452534266820173 ) ) ;
#26068=CARTESIAN_POINT ( 'NONE',  ( -54.95163769728823411, 215.6869285224996986, -3.149950860017881382 ) ) ;
#26094=CARTESIAN_POINT ( 'NONE',  ( -45.05580436395490551, 214.5000000000000284, 0.1155267958017899832 ) ) ;
#26098=CARTESIAN_POINT ( 'NONE',  ( -57.32663769728823411, 204.3130714775002730, 3.149950860017883603 ) ) ;
#26147=CARTESIAN_POINT ( 'NONE',  ( -66.43080436395490551, 205.4999999999999716, -0.1155267958017894420 ) ) ;
#26179=CARTESIAN_POINT ( 'NONE',  ( -33.17336230271182984, 215.6869285224997270, 3.149950860017831200 ) ) ;
#26182=CARTESIAN_POINT ( 'NONE',  ( -53.75669563604516554, 209.8844732041982297, -4.499999999999996447 ) ) ;
#26183=CARTESIAN_POINT ( 'NONE',  ( -35.15997103062156270, 215.5714017266979852, 3.350049139982118618 ) ) ;
#26189=CARTESIAN_POINT ( 'NONE',  ( -57.92038769728823411, 207.6069050685337913, 8.469044688360781947 ) ) ;
#26195=CARTESIAN_POINT ( 'NONE',  ( -44.65997103062156981, 215.5714017266979852, 3.350049139982118618 ) ) ;
#26207=CARTESIAN_POINT ( 'NONE',  ( -59.89955436395490551, 214.8429017333601792, -4.673758765035196383 ) ) ;
#26223=CARTESIAN_POINT ( 'NONE',  ( -50.19419563604517265, 203.5000000000000000, 0.1155267958017914542 ) ) ;
#26225=CARTESIAN_POINT ( 'NONE',  ( -31.78794563604516910, 206.7903428501025758, 3.378800118222471838 ) ) ;
#26228=CARTESIAN_POINT ( 'NONE',  ( -54.55580436395489841, 214.5000000000000284, 0.1155267958017899832 ) ) ;
#26229=CARTESIAN_POINT ( 'NONE',  ( -49.40997103062157692, 217.3034525342668815, 4.350049139982096413 ) ) ;
#26233=CARTESIAN_POINT ( 'NONE',  ( -53.55877896937850124, 212.1620413398627534, -8.530955311639255356 ) ) ;
#26245=CARTESIAN_POINT ( 'NONE',  ( -45.25372103062155560, 216.5309553116391612, -1.626142955000564383 ) ) ;
#26274=CARTESIAN_POINT ( 'NONE',  ( -63.05877896937850835, 211.0902445701383101, -4.530955311639234040 ) ) ;
#26279=CARTESIAN_POINT ( 'NONE',  ( -65.63913769728823411, 206.8500491399821044, -5.686928522499717253 ) ) ;
#26280=CARTESIAN_POINT ( 'NONE',  ( -37.32961230271184405, 212.3930949314663792, 8.469044688360751749 ) ) ;
#26329=CARTESIAN_POINT ( 'NONE',  ( -68.01413769728823411, 212.1499508600178387, 3.954877714930865817 ) ) ;
#26366=CARTESIAN_POINT ( 'NONE',  ( -35.74627896937850124, 203.4690446883607535, -1.626142955000504209 ) ) ;
#26370=CARTESIAN_POINT ( 'NONE',  ( -61.67336230271184405, 213.9548777149308023, 2.149950860017852960 ) ) ;
#26376=CARTESIAN_POINT ( 'NONE',  ( -59.10788769728823411, 218.4690446883607535, 2.393094931466250408 ) ) ;
#26382=CARTESIAN_POINT ( 'NONE',  ( -47.03497103062156981, 204.4285982733020148, -3.350049139982115509 ) ) ;
#26397=CARTESIAN_POINT ( 'NONE',  ( -54.15997103062156981, 215.5714017266979852, 3.350049139982118618 ) ) ;
#26411=CARTESIAN_POINT ( 'NONE',  ( -46.23586230271182984, 206.8500491399821328, 5.686928522499748340 ) ) ;
#26412=CARTESIAN_POINT ( 'NONE',  ( -64.84002896937850835, 204.4285982733020433, 3.350049139982171020 ) ) ;
#26415=CARTESIAN_POINT ( 'NONE',  ( -59.30580436395490551, 214.5000000000000284, 0.1155267958017899832 ) ) ;
#26417=CARTESIAN_POINT ( 'NONE',  ( -37.53497103062155560, 202.6965474657331185, -4.350049139982091084 ) ) ;
#26421=CARTESIAN_POINT ( 'NONE',  ( -61.67336230271184405, 217.4189793300686233, 4.149950860017807663 ) ) ;
#26433=CARTESIAN_POINT ( 'NONE',  ( -53.36830436395489841, 209.8844732041982581, 6.500000000000000888 ) ) ;
#26460=CARTESIAN_POINT ( 'NONE',  ( -33.77455436395489841, 206.6211998817774997, 3.209657149897401585 ) ) ;
#26464=CARTESIAN_POINT ( 'NONE',  ( -61.68080436395489841, 203.5000000000000000, -0.1155267958017335561 ) ) ;
#26466=CARTESIAN_POINT ( 'NONE',  ( -35.74627896937850124, 201.4690446883607251, -2.162041339862721845 ) ) ;
#26471=CARTESIAN_POINT ( 'NONE',  ( -57.91294563604515133, 214.6737587650350747, -4.842901733360249317 ) ) ;
#26478=CARTESIAN_POINT ( 'NONE',  ( -65.04538769728823411, 211.8571965466040012, -6.469044688360769513 ) ) ;
#26507=PRODUCT_DEFINITION_SHAPE ( 'NONE', 'NONE',  #31497 ) ;
#26517=CARTESIAN_POINT ( 'NONE',  ( -69.00372103062157692, 214.5309553116392749, -1.090244570138262148 ) ) ;
#26554=CARTESIAN_POINT ( 'NONE',  ( -30.00669563604516910, 209.8844732041982013, -6.500000000000000888 ) ) ;
#26559=CARTESIAN_POINT ( 'NONE',  ( -56.52752896937850124, 212.3500491399821613, 3.839350919129088435 ) ) ;
#26560=CARTESIAN_POINT ( 'NONE',  ( -35.95163769728823411, 215.6869285224996986, -3.149950860017881382 ) ) ;
#26565=CARTESIAN_POINT ( 'NONE',  ( -61.87872103062156981, 201.4690446883607819, 2.162041339862843525 ) ) ;
#26571=UNCERTAINTY_MEASURE_WITH_UNIT (LENGTH_MEASURE( 1.000000000000000082E-05 ), #37252, 'distance_accuracy_value', 'NONE');
#26584=CARTESIAN_POINT ( 'NONE',  ( -51.19122103062155560, 208.3738570449993404, -6.530955311639226935 ) ) ;
#26599=CARTESIAN_POINT ( 'NONE',  ( -44.85044563604515844, 205.1570982666397072, -4.673758765035155527 ) ) ;
#26601=CARTESIAN_POINT ( 'NONE',  ( -65.23586230271183695, 206.8500491399821328, 5.686928522499748340 ) ) ;
#26606=CARTESIAN_POINT ( 'NONE',  ( -65.83705436395491972, 206.7903428501026042, -3.378800118222489157 ) ) ;
#26607=CARTESIAN_POINT ( 'NONE',  ( -35.75372103062156981, 218.5309553116391896, -2.162041339862839084 ) ) ;
#26612=CARTESIAN_POINT ( 'NONE',  ( -54.35044563604515844, 203.6929966515019430, -6.137860380172892150 ) ) ;
#26622=CARTESIAN_POINT ( 'NONE',  ( -51.38913769728823411, 206.8500491399821044, -5.686928522499717253 ) ) ;
#26649=CARTESIAN_POINT ( 'NONE',  ( -66.62127896937849414, 214.5309553116392749, 1.090244570138288127 ) ) ;
#26653=CARTESIAN_POINT ( 'NONE',  ( -55.94122103062156270, 208.3738570449993404, -6.530955311639226935 ) ) ;
#26654=CARTESIAN_POINT ( 'NONE',  ( -32.38169563604516554, 210.1155267958018271, 8.500000000000003553 ) ) ;
#26660=CARTESIAN_POINT ( 'NONE',  ( -57.31919563604516554, 216.5000000000000000, -0.1155267958017906493 ) ) ;
#26667=CARTESIAN_POINT ( 'NONE',  ( -65.24330436395489130, 210.1155267958017134, -6.500000000000000888 ) ) ;
#26705=CARTESIAN_POINT ( 'NONE',  ( -68.60788769728823411, 214.4690446883608104, 1.321298161741840893 ) ) ;
#26743=CARTESIAN_POINT ( 'NONE',  ( -67.01711230271185116, 218.4690446883607535, -2.393094931466363651 ) ) ;
#26748=CARTESIAN_POINT ( 'NONE',  ( -50.78794563604517975, 206.7903428501025758, 3.378800118222471838 ) ) ;
#26750=CARTESIAN_POINT ( 'NONE',  ( -37.53497103062156981, 204.4285982733020148, -3.350049139982115509 ) ) ;
#26755=CARTESIAN_POINT ( 'NONE',  ( -65.83705436395491972, 203.8621396198270475, -6.307003348497942419 ) ) ;
#26790=CARTESIAN_POINT ( 'NONE',  ( -40.89211230271182274, 203.5309553116391896, 1.857196546604092724 ) ) ;
#26792=CARTESIAN_POINT ( 'NONE',  ( -63.45461230271182274, 208.1428034533959135, -6.469044688360754414 ) ) ;
#26796=CARTESIAN_POINT ( 'NONE',  ( -64.25372103062157692, 214.5309553116392749, -1.090244570138262148 ) ) ;
#26797=CARTESIAN_POINT ( 'NONE',  ( -36.14955436395489841, 216.3070033484980002, -6.137860380172975638 ) ) ;
#26801=CARTESIAN_POINT ( 'NONE',  ( -64.04836230271183695, 202.5810206699313767, -4.149950860017804111 ) ) ;
#26813=CARTESIAN_POINT ( 'NONE',  ( -34.17038769728823411, 208.1428034533959703, 6.469044688360770401 ) ) ;
#26841=CARTESIAN_POINT ( 'NONE',  ( -67.41294563604516554, 213.2096571498974527, -3.378800118222469617 ) ) ;
#26845=CARTESIAN_POINT ( 'NONE',  ( -56.33705436395489841, 205.3262412349647263, -4.842901733360204020 ) ) ;
#26846=CARTESIAN_POINT ( 'NONE',  ( -69.79538769728823411, 212.3930949314662371, -8.469044688360781947 ) ) ;
#26852=CARTESIAN_POINT ( 'NONE',  ( -56.32961230271183695, 211.8571965466040297, 6.469044688360755302 ) ) ;
#26859=CARTESIAN_POINT ( 'NONE',  ( -66.23288769728823411, 203.5309553116391896, -1.857196546604028997 ) ) ;
#26864=CARTESIAN_POINT ( 'NONE',  ( -35.35788769728823411, 218.4690446883607535, 2.393094931466250408 ) ) ;
#26900=CARTESIAN_POINT ( 'NONE',  ( -34.56622103062155560, 211.6261429550005744, 6.530955311639227823 ) ) ;
#26935=CARTESIAN_POINT ( 'NONE',  ( -56.13169563604517265, 210.1155267958018271, 8.500000000000003553 ) ) ;
#26938=CARTESIAN_POINT ( 'NONE',  ( -46.03794563604517975, 206.7903428501025758, 3.378800118222471838 ) ) ;
#26945=CARTESIAN_POINT ( 'NONE',  ( -54.15997103062156981, 217.3034525342668815, 4.350049139982096413 ) ) ;
#26980=CARTESIAN_POINT ( 'NONE',  ( -39.30877896937849414, 211.6261429550004891, -6.530955311639245586 ) ) ;
#26982=CARTESIAN_POINT ( 'NONE',  ( -66.42336230271182274, 215.6869285224997270, 3.149950860017831200 ) ) ;
#26985=CARTESIAN_POINT ( 'NONE',  ( -46.24330436395489841, 210.1155267958017703, -4.499999999999996447 ) ) ;
#26986=CARTESIAN_POINT ( 'NONE',  ( -68.80580436395490551, 216.5000000000000000, 0.1155267958017343610 ) ) ;
#26989=CARTESIAN_POINT ( 'NONE',  ( -40.69419563604516554, 201.5000000000000000, 0.1155267958018195706 ) ) ;
#26991=DIRECTION ( 'NONE',  ( -0.1155267958017759666, -0.9933043639548629899, 2.756973438308332598E-14 ) ) ;
#27004=CARTESIAN_POINT ( 'NONE',  ( -31.99330436395490196, 210.1155267958017134, -6.500000000000000888 ) ) ;
#27033=CARTESIAN_POINT ( 'NONE',  ( -62.46502896937850124, 213.8393509191290889, -2.350049139982142155 ) ) ;
#27037=CARTESIAN_POINT ( 'NONE',  ( -47.62872103062154849, 203.4690446883607535, 1.626142955000567936 ) ) ;
#27038=CARTESIAN_POINT ( 'NONE',  ( -34.75669563604515844, 209.8844732041981729, -8.500000000000003553 ) ) ;
#27043=CARTESIAN_POINT ( 'NONE',  ( -56.13169563604517265, 210.1155267958017703, 6.500000000000000888 ) ) ;
#27052=CARTESIAN_POINT ( 'NONE',  ( -61.87872103062155560, 203.4690446883607535, 1.626142955000567936 ) ) ;
#27056=CARTESIAN_POINT ( 'NONE',  ( -40.89955436395489841, 216.3070033484980002, -6.137860380172975638 ) ) ;
#27129=CARTESIAN_POINT ( 'NONE',  ( -53.16294563604516554, 216.1378603801729241, -6.307003348498026796 ) ) ;
#27132=CARTESIAN_POINT ( 'NONE',  ( -42.07961230271182984, 211.3212981617417938, 4.469044688360757966 ) ) ;
#27138=CARTESIAN_POINT ( 'NONE',  ( -47.62872103062157692, 201.4690446883607819, 2.162041339862843525 ) ) ;
#27169=CARTESIAN_POINT ( 'NONE',  ( -41.09002896937850124, 204.4285982733020433, 3.350049139982171020 ) ) ;
#27170=CARTESIAN_POINT ( 'NONE',  ( -60.68377896937848703, 208.3738570449995109, 6.530955311639247363 ) ) ;
#27174=CARTESIAN_POINT ( 'NONE',  ( -49.40997103062157692, 213.8393509191290889, 2.350049139982164359 ) ) ;
#27175=CARTESIAN_POINT ( 'NONE',  ( -52.18080436395490551, 203.5000000000000000, -0.1155267958017335561 ) ) ;
#27179=CARTESIAN_POINT ( 'NONE',  ( -50.59002896937850835, 202.6965474657332038, 4.350049139982197666 ) ) ;
#27219=CARTESIAN_POINT ( 'NONE',  ( -56.52752896937850124, 212.3500491399821613, 3.839350919129088435 ) ) ;
#27223=CARTESIAN_POINT ( 'NONE',  ( -42.28497103062156270, 204.4285982733020148, -3.350049139982115509 ) ) ;
#27224=CARTESIAN_POINT ( 'NONE',  ( -64.05580436395490551, 218.5000000000000000, 0.1155267958017064944 ) ) ;
#27230=CARTESIAN_POINT ( 'NONE',  ( -47.22544563604515844, 214.8429017333602360, 4.673758765035156415 ) ) ;
#27239=CARTESIAN_POINT ( 'NONE',  ( -49.60788769728822700, 216.4690446883607535, 1.857196546604031662 ) ) ;
#27243=CARTESIAN_POINT ( 'NONE',  ( -38.72247103062156981, 205.6499508600178956, 7.303452534266880569 ) ) ;
#27317=CARTESIAN_POINT ( 'NONE',  ( -53.36086230271183695, 214.1499508600178387, -7.418979330068641964 ) ) ;
#27320=CARTESIAN_POINT ( 'NONE',  ( -40.10044563604517265, 206.6211998817775566, -3.209657149897419348 ) ) ;
#27326=CARTESIAN_POINT ( 'NONE',  ( -52.97247103062156270, 205.6499508600178956, 7.303452534266880569 ) ) ;
#27355=CARTESIAN_POINT ( 'NONE',  ( -35.35044563604516554, 205.1570982666397072, -4.673758765035155527 ) ) ;
#27356=CARTESIAN_POINT ( 'NONE',  ( -50.78794563604515133, 205.3262412349647832, 4.842901733360250205 ) ) ;
#27360=CARTESIAN_POINT ( 'NONE',  ( -41.29538769728824121, 211.3212981617418222, -4.469044688360751749 ) ) ;
#27361=CARTESIAN_POINT ( 'NONE',  ( -62.07663769728823411, 204.3130714775002730, 3.149950860017883603 ) ) ;
#27365=CARTESIAN_POINT ( 'NONE',  ( -47.62127896937850124, 218.5309553116392465, 2.162041339862725842 ) ) ;
#27376=CARTESIAN_POINT ( 'NONE',  ( -38.92038769728823411, 208.1428034533959703, 6.469044688360770401 ) ) ;
#27402=CARTESIAN_POINT ( 'NONE',  ( -50.59002896937850835, 206.1606490808709111, 2.350049139982143931 ) ) ;
#27406=CARTESIAN_POINT ( 'NONE',  ( -41.88913769728823411, 206.8500491399821044, -5.686928522499717253 ) ) ;
#27407=CARTESIAN_POINT ( 'NONE',  ( -53.36830436395490551, 209.8844732041983150, 8.500000000000003553 ) ) ;
#27412=CARTESIAN_POINT ( 'NONE',  ( -45.44419563604516554, 203.5000000000000000, 0.1155267958017914542 ) ) ;
#27420=CARTESIAN_POINT ( 'NONE',  ( -59.89955436395489841, 214.8429017333601792, -4.673758765035197271 ) ) ;
#27425=CARTESIAN_POINT ( 'NONE',  ( -33.37872103062156981, 201.4690446883607819, 2.162041339862843525 ) ) ;
#27436=CARTESIAN_POINT ( 'NONE',  ( -60.88913769728823411, 206.8500491399821044, -5.686928522499717253 ) ) ;
#27455=CARTESIAN_POINT ( 'NONE',  ( -55.14955436395491262, 213.3788001182225003, -3.209657149897400252 ) ) ;
#27507=CARTESIAN_POINT ( 'NONE',  ( -55.14211230271182984, 201.5309553116392181, 2.393094931466368980 ) ) ;
#27511=CARTESIAN_POINT ( 'NONE',  ( -50.98586230271183695, 207.8500491399821613, 3.954877714930852495 ) ) ;
#27517=CARTESIAN_POINT ( 'NONE',  ( -48.42038769728824832, 207.6069050685337913, 8.469044688360781947 ) ) ;
#27545=CARTESIAN_POINT ( 'NONE',  ( -37.13169563604516554, 210.1155267958017703, 6.500000000000000888 ) ) ;
#27546=CARTESIAN_POINT ( 'NONE',  ( -58.90252896937850124, 206.6499508600178387, -5.571401726697954970 ) ) ;
#27549=CARTESIAN_POINT ( 'NONE',  ( -47.03497103062157692, 206.1606490808709111, -2.350049139982163027 ) ) ;
#27551=CARTESIAN_POINT ( 'NONE',  ( -60.09747103062156981, 213.3500491399821328, -5.571401726697985168 ) ) ;
#27556=CARTESIAN_POINT ( 'NONE',  ( -41.48586230271182984, 205.8500491399821613, 7.418979330068642852 ) ) ;
#27567=CARTESIAN_POINT ( 'NONE',  ( -33.37872103062156981, 203.4690446883607535, 1.626142955000567936 ) ) ;
#27594=CARTESIAN_POINT ( 'NONE',  ( -54.74627896937850835, 205.4690446883607535, -1.090244570138286351 ) ) ;
#27597=CARTESIAN_POINT ( 'NONE',  ( -51.78497103062156981, 204.4285982733020148, -3.350049139982115509 ) ) ;
#27598=CARTESIAN_POINT ( 'NONE',  ( -51.78497103062156981, 202.6965474657331185, -4.350049139982091084 ) ) ;
#27604=CARTESIAN_POINT ( 'NONE',  ( -49.20461230271183695, 208.1428034533959135, -6.469044688360754414 ) ) ;
#27613=CARTESIAN_POINT ( 'NONE',  ( -61.28497103062156981, 204.4285982733020148, -3.350049139982115509 ) ) ;
#27617=CARTESIAN_POINT ( 'NONE',  ( -41.88913769728823411, 205.8500491399820760, -7.418979330068584233 ) ) ;
#27644=CARTESIAN_POINT ( 'NONE',  ( -50.59747103062156981, 212.3500491399821613, -3.839350919129076445 ) ) ;
#27690=CARTESIAN_POINT ( 'NONE',  ( -52.37127896937850835, 218.5309553116392465, 2.162041339862725842 ) ) ;
#27695=CARTESIAN_POINT ( 'NONE',  ( -66.62127896937846572, 216.5309553116391612, 1.626142955000506873 ) ) ;
#27732=CARTESIAN_POINT ( 'NONE',  ( -56.13169563604517265, 210.1155267958017703, 6.500000000000000888 ) ) ;
#27735=CARTESIAN_POINT ( 'NONE',  ( -35.75372103062156981, 214.5309553116392749, -1.090244570138262148 ) ) ;
#27736=CARTESIAN_POINT ( 'NONE',  ( -61.87872103062154849, 203.4690446883607535, 1.626142955000567936 ) ) ;
#27742=CARTESIAN_POINT ( 'NONE',  ( -48.61086230271182984, 214.1499508600178387, -7.418979330068641964 ) ) ;
#27783=CARTESIAN_POINT ( 'NONE',  ( -57.12127896937850124, 214.5309553116392749, 1.090244570138288127 ) ) ;
#27787=CARTESIAN_POINT ( 'NONE',  ( -47.23288769728823411, 203.5309553116391612, -1.857196546604028775 ) ) ;
#27788=CARTESIAN_POINT ( 'NONE',  ( -60.29538769728823411, 212.3930949314662371, -8.469044688360781947 ) ) ;
#27792=CARTESIAN_POINT ( 'NONE',  ( -49.60044563604517265, 205.1570982666397072, -4.673758765035155527 ) ) ;
#27801=CARTESIAN_POINT ( 'NONE',  ( -52.18080436395490551, 203.5000000000000000, -0.1155267958017335561 ) ) ;
#27805=CARTESIAN_POINT ( 'NONE',  ( -67.61830436395489130, 209.8844732041982581, 6.500000000000000888 ) ) ;
#27827=CARTESIAN_POINT ( 'NONE',  ( -56.73288769728824832, 205.5309553116392465, -1.321298161741839117 ) ) ;
#27871=DIRECTION ( 'NONE',  ( -0.1155267958017757585, -0.9933043639548629899, 1.378486719154166141E-14 ) ) ;
#27873=CARTESIAN_POINT ( 'NONE',  ( -38.51711230271182984, 218.4690446883607535, -2.393094931466363651 ) ) ;
#27876=CARTESIAN_POINT ( 'NONE',  ( -67.80877896937850835, 211.6261429550004607, -6.530955311639245586 ) ) ;
#27913=CARTESIAN_POINT ( 'NONE',  ( -56.52752896937850124, 213.3500491399821613, 5.571401726697954970 ) ) ;
#27916=CARTESIAN_POINT ( 'NONE',  ( -35.55580436395489130, 214.5000000000000284, 0.1155267958017899832 ) ) ;
#27917=CARTESIAN_POINT ( 'NONE',  ( -58.31622103062155560, 211.6261429550005744, 6.530955311639227823 ) ) ;
#27921=CARTESIAN_POINT ( 'NONE',  ( -69.39955436395489130, 216.3070033484980002, -6.137860380172975638 ) ) ;
#27931=DIRECTION ( 'NONE',  ( 0.1155267958017759666, 0.9933043639548631010, -1.378486719154166141E-14 ) ) ;
#27961=CARTESIAN_POINT ( 'NONE',  ( -60.09002896937850124, 204.4285982733020433, 3.350049139982171020 ) ) ;
#27963=CARTESIAN_POINT ( 'NONE',  ( -59.49627896937850835, 205.4690446883607535, -1.090244570138286351 ) ) ;
#27968=CARTESIAN_POINT ( 'NONE',  ( -67.61830436395490551, 209.8844732041982297, 4.499999999999996447 ) ) ;
#27969=CARTESIAN_POINT ( 'NONE',  ( -58.71205436395490551, 216.1378603801730094, 6.307003348497944195 ) ) ;
#27973=CARTESIAN_POINT ( 'NONE',  ( -41.48586230271182984, 206.8500491399821328, 5.686928522499748340 ) ) ;
#27982=CARTESIAN_POINT ( 'NONE',  ( -53.17038769728823411, 208.1428034533959703, 6.469044688360771289 ) ) ;
#27987=CARTESIAN_POINT ( 'NONE',  ( -69.00372103062157692, 216.5309553116391612, -1.626142955000564383 ) ) ;
#28010=CARTESIAN_POINT ( 'NONE',  ( -56.33705436395490551, 206.7903428501026042, -3.378800118222489157 ) ) ;
#28059=CARTESIAN_POINT ( 'NONE',  ( -41.48586230271182984, 205.8500491399821613, 7.418979330068642852 ) ) ;
#28062=CARTESIAN_POINT ( 'NONE',  ( -66.42336230271182274, 215.6869285224997270, 3.149950860017831200 ) ) ;
#28066=CARTESIAN_POINT ( 'NONE',  ( -43.47247103062156981, 206.6499508600178672, 5.571401726697986057 ) ) ;
#28097=CARTESIAN_POINT ( 'NONE',  ( -43.86086230271183695, 213.1499508600178387, -5.686928522499747451 ) ) ;
#28103=CARTESIAN_POINT ( 'NONE',  ( -64.84002896937849414, 206.1606490808709111, 2.350049139982143931 ) ) ;
#28105=CARTESIAN_POINT ( 'NONE',  ( -47.82663769728823411, 204.3130714775002730, 3.149950860017883603 ) ) ;
#28109=CARTESIAN_POINT ( 'NONE',  ( -68.21205436395490551, 216.1378603801730094, 6.307003348497944195 ) ) ;
#28145=CARTESIAN_POINT ( 'NONE',  ( -63.25669563604516554, 209.8844732041982013, -6.500000000000000888 ) ) ;
#28147=CARTESIAN_POINT ( 'NONE',  ( -39.90252896937850124, 207.6499508600178387, -3.839350919129087547 ) ) ;
#28151=CARTESIAN_POINT ( 'NONE',  ( -36.34747103062156981, 213.3500491399821328, -5.571401726697985168 ) ) ;
#28152=CARTESIAN_POINT ( 'NONE',  ( -55.14955436395491262, 216.3070033484980002, -6.137860380172975638 ) ) ;
#28156=CARTESIAN_POINT ( 'NONE',  ( -65.63169563604516554, 210.1155267958018271, 8.500000000000003553 ) ) ;
#28166=CARTESIAN_POINT ( 'NONE',  ( -47.62872103062156270, 203.4690446883607535, 1.626142955000567936 ) ) ;
#28171=CARTESIAN_POINT ( 'NONE',  ( -56.53497103062156270, 204.4285982733020148, -3.350049139982115509 ) ) ;
#28172=( NAMED_UNIT ( * ) SI_UNIT ( $, .STERADIAN. ) SOLID_ANGLE_UNIT ( ) );
#28198=CARTESIAN_POINT ( 'NONE',  ( -53.56622103062157692, 211.0902445701382533, 4.530955311639240257 ) ) ;
#28202=CARTESIAN_POINT ( 'NONE',  ( -66.23288769728823411, 203.5309553116391612, -1.857196546604028775 ) ) ;
#28248=CARTESIAN_POINT ( 'NONE',  ( -36.93377896937849414, 207.8379586601372750, 8.530955311639258909 ) ) ;
#28251=CARTESIAN_POINT ( 'NONE',  ( -38.51711230271182984, 214.4690446883608104, -1.321298161741814914 ) ) ;
#28254=CARTESIAN_POINT ( 'NONE',  ( -45.25372103062155560, 216.5309553116391612, -1.626142955000564383 ) ) ;
#28283=CARTESIAN_POINT ( 'NONE',  ( -44.25669563604516554, 209.8844732041982013, -6.500000000000000888 ) ) ;
#28287=CARTESIAN_POINT ( 'NONE',  ( -33.18080436395489841, 205.4999999999999716, -0.1155267958017894420 ) ) ;
#28288=CARTESIAN_POINT ( 'NONE',  ( -43.86830436395490551, 209.8844732041982581, 6.500000000000000888 ) ) ;
#28293=CARTESIAN_POINT ( 'NONE',  ( -31.19419563604517265, 201.5000000000000000, 0.1155267958018195706 ) ) ;
#28312=CARTESIAN_POINT ( 'NONE',  ( -66.03497103062157692, 204.4285982733020148, -3.350049139982115509 ) ) ;
#28328=CARTESIAN_POINT ( 'NONE',  ( -57.71502896937850124, 215.5714017266979567, -3.350049139982168800 ) ) ;
#28331=CARTESIAN_POINT ( 'NONE',  ( -38.91294563604516554, 213.2096571498974527, -3.378800118222469617 ) ) ;
#28335=CARTESIAN_POINT ( 'NONE',  ( -37.73288769728821279, 203.5309553116391612, -1.857196546604028775 ) ) ;
#28336=CARTESIAN_POINT ( 'NONE',  ( -40.89955436395489841, 216.3070033484980002, -6.137860380172975638 ) ) ;
#28342=CARTESIAN_POINT ( 'NONE',  ( -65.03794563604515133, 203.8621396198271043, 6.307003348498029460 ) ) ;
#28352=CARTESIAN_POINT ( 'NONE',  ( -60.88913769728823411, 206.8500491399821044, -5.686928522499717253 ) ) ;
#28377=CARTESIAN_POINT ( 'NONE',  ( -41.49330436395490551, 210.1155267958017703, -4.499999999999996447 ) ) ;
#28421=CARTESIAN_POINT ( 'NONE',  ( -40.10044563604517265, 203.6929966515019430, -6.137860380172892150 ) ) ;
#28424=CARTESIAN_POINT ( 'NONE',  ( -30.99627896937850480, 205.4690446883607535, -1.090244570138286351 ) ) ;
#28429=CARTESIAN_POINT ( 'NONE',  ( -44.26413769728823411, 213.1499508600178672, 5.686928522499718142 ) ) ;
#28464=CARTESIAN_POINT ( 'NONE',  ( -39.30877896937850124, 211.6261429550004607, -6.530955311639245586 ) ) ;
#28468=CARTESIAN_POINT ( 'NONE',  ( -32.38913769728823411, 207.8500491399821613, -3.954877714930864485 ) ) ;
#28469=CARTESIAN_POINT ( 'NONE',  ( -43.67038769728823411, 208.1428034533959703, 6.469044688360770401 ) ) ;
#28475=CARTESIAN_POINT ( 'NONE',  ( -36.73586230271183695, 205.8500491399821613, 7.418979330068642852 ) ) ;
#28493=CARTESIAN_POINT ( 'NONE',  ( -65.83705436395487709, 205.3262412349647263, -4.842901733360204020 ) ) ;
#28510=CARTESIAN_POINT ( 'NONE',  ( -60.48586230271183695, 206.8500491399821328, 5.686928522499748340 ) ) ;
#28512=CARTESIAN_POINT ( 'NONE',  ( -42.47544563604517265, 213.3788001182224718, 3.209657149897419348 ) ) ;
#28515=CARTESIAN_POINT ( 'NONE',  ( -34.96205436395488420, 214.6737587650352168, 4.842901733360204908 ) ) ;
#28516=CARTESIAN_POINT ( 'NONE',  ( -47.03497103062157692, 202.6965474657331185, -4.350049139982091084 ) ) ;
#28521=CARTESIAN_POINT ( 'NONE',  ( -32.38169563604517265, 210.1155267958017703, 6.500000000000000888 ) ) ;
#28532=CARTESIAN_POINT ( 'NONE',  ( -58.11830436395490551, 209.8844732041982581, 6.500000000000000888 ) ) ;
#28557=CARTESIAN_POINT ( 'NONE',  ( -47.03497103062157692, 206.1606490808709111, -2.350049139982163027 ) ) ;
#28608=CARTESIAN_POINT ( 'NONE',  ( -54.35044563604515133, 205.1570982666397072, -4.673758765035155527 ) ) ;
#28611=CARTESIAN_POINT ( 'NONE',  ( -40.50372103062156981, 216.5309553116391612, -1.626142955000564383 ) ) ;
#28649=CARTESIAN_POINT ( 'NONE',  ( -38.12127896937848703, 216.5309553116391612, 1.626142955000506873 ) ) ;
#28652=CARTESIAN_POINT ( 'NONE',  ( -59.89211230271182274, 205.5309553116392465, 1.321298161741817356 ) ) ;
#28653=CARTESIAN_POINT ( 'NONE',  ( -42.68080436395489841, 203.5000000000000000, -0.1155267958017335561 ) ) ;
#28658=CARTESIAN_POINT ( 'NONE',  ( -32.38169563604516554, 210.1155267958018271, 8.500000000000003553 ) ) ;
#28698=CARTESIAN_POINT ( 'NONE',  ( -55.73586230271182984, 206.8500491399821328, 5.686928522499748340 ) ) ;
#28700=CARTESIAN_POINT ( 'NONE',  ( -41.09002896937850124, 206.1606490808709111, 2.350049139982143931 ) ) ;
#28703=CARTESIAN_POINT ( 'NONE',  ( -37.93080436395489841, 203.5000000000000000, -0.1155267958017335561 ) ) ;
#28704=CARTESIAN_POINT ( 'NONE',  ( -43.27455436395490551, 203.6929966515020283, 6.137860380172978303 ) ) ;
#28709=CARTESIAN_POINT ( 'NONE',  ( -35.94419563604516554, 203.5000000000000000, 0.1155267958017914542 ) ) ;
#28720=CARTESIAN_POINT ( 'NONE',  ( -51.58705436395488420, 205.3262412349647263, -4.842901733360204020 ) ) ;
#28743=CARTESIAN_POINT ( 'NONE',  ( -40.30580436395490551, 214.5000000000000284, 0.1155267958017899832 ) ) ;
#28799=CARTESIAN_POINT ( 'NONE',  ( -44.65997103062156981, 215.5714017266979852, 3.350049139982118618 ) ) ;
#28833=CARTESIAN_POINT ( 'NONE',  ( -36.14211230271182984, 203.5309553116391612, 1.857196546604092280 ) ) ;
#28838=CARTESIAN_POINT ( 'NONE',  ( -60.09002896937850124, 206.1606490808709111, 2.350049139982143931 ) ) ;
#28839=CARTESIAN_POINT ( 'NONE',  ( -40.10788769728823411, 216.4690446883607535, 1.857196546604031662 ) ) ;
#28845=CARTESIAN_POINT ( 'NONE',  ( -61.08705436395490551, 203.8621396198270475, -6.307003348497942419 ) ) ;
#28851=CARTESIAN_POINT ( 'NONE',  ( -38.92038769728823411, 208.1428034533959703, 6.469044688360771289 ) ) ;
#28863=CARTESIAN_POINT ( 'NONE',  ( -56.93080436395490551, 203.5000000000000000, -0.1155267958017335561 ) ) ;
#28883=CARTESIAN_POINT ( 'NONE',  ( -53.55877896937849414, 211.6261429550004891, -6.530955311639245586 ) ) ;
#28886=CARTESIAN_POINT ( 'NONE',  ( -36.14211230271182984, 205.5309553116392465, 1.321298161741817356 ) ) ;
#28890=CARTESIAN_POINT ( 'NONE',  ( -59.89955436395489841, 213.3788001182225003, -3.209657149897400252 ) ) ;
#28891=CARTESIAN_POINT ( 'NONE',  ( -41.09747103062157692, 214.3500491399821044, -7.303452534266878793 ) ) ;
#28895=CARTESIAN_POINT ( 'NONE',  ( -62.66294563604517265, 216.1378603801729241, -6.307003348498026796 ) ) ;
#28906=CARTESIAN_POINT ( 'NONE',  ( -50.39955436395490551, 214.8429017333601792, -4.673758765035196383 ) ) ;
#28934=CARTESIAN_POINT ( 'NONE',  ( -39.71205436395491262, 213.2096571498974242, 3.378800118222489601 ) ) ;
#28938=CARTESIAN_POINT ( 'NONE',  ( -58.71205436395488420, 214.6737587650352168, 4.842901733360204908 ) ) ;
#28983=CARTESIAN_POINT ( 'NONE',  ( -35.35788769728823411, 216.4690446883607535, 1.857196546604031662 ) ) ;
#29014=CARTESIAN_POINT ( 'NONE',  ( -32.18377896937850835, 208.3738570449995109, 6.530955311639247363 ) ) ;
#29017=CARTESIAN_POINT ( 'NONE',  ( -56.32961230271183695, 211.3212981617417938, 4.469044688360757966 ) ) ;
#29018=CARTESIAN_POINT ( 'NONE',  ( -38.32663769728824121, 204.3130714775002730, 3.149950860017883603 ) ) ;
#29026=CARTESIAN_POINT ( 'NONE',  ( -58.71205436395490551, 216.1378603801730094, 6.307003348497944195 ) ) ;
#29032=CARTESIAN_POINT ( 'NONE',  ( -37.13913769728823411, 206.8500491399821044, -5.686928522499717253 ) ) ;
#29043=CARTESIAN_POINT ( 'NONE',  ( -56.13913769728823411, 206.8500491399821044, -5.686928522499717253 ) ) ;
#29061=CARTESIAN_POINT ( 'NONE',  ( -48.61086230271182984, 213.1499508600178387, -5.686928522499747451 ) ) ;
#29063=CARTESIAN_POINT ( 'NONE',  ( -33.17336230271183695, 213.9548777149308023, 2.149950860017852960 ) ) ;
#29067=CARTESIAN_POINT ( 'NONE',  ( -64.84747103062156270, 212.3500491399821613, -3.839350919129076445 ) ) ;
#29069=CARTESIAN_POINT ( 'NONE',  ( -39.11830436395489841, 209.8844732041983150, 8.500000000000003553 ) ) ;
#29073=CARTESIAN_POINT ( 'NONE',  ( -61.07961230271182984, 212.3930949314663792, 8.469044688360751749 ) ) ;
#29087=CARTESIAN_POINT ( 'NONE',  ( -45.64955436395490551, 214.8429017333601792, -4.673758765035196383 ) ) ;
#29112=CARTESIAN_POINT ( 'NONE',  ( -37.93080436395490551, 205.4999999999999716, -0.1155267958017894420 ) ) ;
#29116=CARTESIAN_POINT ( 'NONE',  ( -53.56622103062157692, 211.6261429550005744, 6.530955311639227823 ) ) ;
#29117=CARTESIAN_POINT ( 'NONE',  ( -36.53794563604517265, 203.8621396198271043, 6.307003348498029460 ) ) ;
#29131=CARTESIAN_POINT ( 'NONE',  ( -68.21205436395490551, 214.6737587650351884, 4.842901733360205796 ) ) ;
#29132=CIRCLE ( 'NONE', #30373, 1.000000000000002220 ) ;
#29168=CARTESIAN_POINT ( 'NONE',  ( -64.25372103062157692, 214.5309553116392749, -1.090244570138262148 ) ) ;
#29206=CARTESIAN_POINT ( 'NONE',  ( -67.80877896937849414, 212.1620413398627534, -8.530955311639255356 ) ) ;
#29210=CARTESIAN_POINT ( 'NONE',  ( -52.17336230271184405, 213.9548777149308023, 2.149950860017852960 ) ) ;
#29216=CARTESIAN_POINT ( 'NONE',  ( -62.67038769728824121, 207.6069050685337913, 8.469044688360781947 ) ) ;
#29222=CARTESIAN_POINT ( 'NONE',  ( -47.43080436395489841, 203.5000000000000000, -0.1155267958017335561 ) ) ;
#29236=CARTESIAN_POINT ( 'NONE',  ( -53.17038769728823411, 208.1428034533959703, 6.469044688360770401 ) ) ;
#29251=CARTESIAN_POINT ( 'NONE',  ( -46.63169563604516554, 210.1155267958017703, 6.500000000000000888 ) ) ;
#29252=CARTESIAN_POINT ( 'NONE',  ( -65.82961230271179431, 211.8571965466040297, 6.469044688360755302 ) ) ;
#29256=CARTESIAN_POINT ( 'NONE',  ( -63.06622103062156270, 211.0902445701382533, 4.530955311639240257 ) ) ;
#29258=CARTESIAN_POINT ( 'NONE',  ( -64.45163769728823411, 215.6869285224996986, -3.149950860017881382 ) ) ;
#29263=CARTESIAN_POINT ( 'NONE',  ( -63.65252896937850124, 205.6499508600178103, -7.303452534266820173 ) ) ;
#29275=CARTESIAN_POINT ( 'NONE',  ( -52.57663769728823411, 204.3130714775002730, 3.149950860017883603 ) ) ;
#29303=CARTESIAN_POINT ( 'NONE',  ( -62.66294563604517265, 213.2096571498974527, -3.378800118222469617 ) ) ;
#29308=CARTESIAN_POINT ( 'NONE',  ( -64.64955436395490551, 214.8429017333601792, -4.673758765035196383 ) ) ;
#29309=CARTESIAN_POINT ( 'NONE',  ( -31.78794563604516910, 203.8621396198271043, 6.307003348498029460 ) ) ;
#29314=CARTESIAN_POINT ( 'NONE',  ( -52.56919563604516554, 216.5000000000000000, -0.1155267958017906493 ) ) ;
#29323=CARTESIAN_POINT ( 'NONE',  ( -63.06622103062156981, 211.6261429550005744, 6.530955311639228711 ) ) ;
#29361=CARTESIAN_POINT ( 'NONE',  ( -32.19122103062156981, 208.3738570449993404, -6.530955311639226935 ) ) ;
#29401=APPLICATION_CONTEXT ( 'automotive_design' ) ;
#29402=CARTESIAN_POINT ( 'NONE',  ( -30.60044563604515488, 205.1570982666397072, -4.673758765035155527 ) ) ;
#29406=CARTESIAN_POINT ( 'NONE',  ( -63.45461230271184405, 208.6787018382582346, -4.469044688360757966 ) ) ;
#29408=CARTESIAN_POINT ( 'NONE',  ( -36.94122103062157692, 208.3738570449993404, -6.530955311639226935 ) ) ;
#29413=CARTESIAN_POINT ( 'NONE',  ( -54.35788769728822700, 218.4690446883607535, 2.393094931466250408 ) ) ;
#29418=CARTESIAN_POINT ( 'NONE',  ( -48.81622103062156981, 211.6261429550005744, 6.530955311639228711 ) ) ;
#29431=CARTESIAN_POINT ( 'NONE',  ( -60.29538769728823411, 211.8571965466039444, -6.469044688360768625 ) ) ;
#29446=CARTESIAN_POINT ( 'NONE',  ( -50.78794563604516554, 205.3262412349648116, 4.842901733360249317 ) ) ;
#29448=CARTESIAN_POINT ( 'NONE',  ( -30.20461230271183339, 208.6787018382582346, -4.469044688360757966 ) ) ;
#29451=CARTESIAN_POINT ( 'NONE',  ( -62.07663769728824121, 206.0451222850691408, 2.149950860017832532 ) ) ;
#29452=CARTESIAN_POINT ( 'NONE',  ( -64.25372103062154849, 216.5309553116391612, -1.626142955000564383 ) ) ;
#29456=CARTESIAN_POINT ( 'NONE',  ( -57.31919563604516554, 218.5000000000000000, -0.1155267958018185298 ) ) ;
#29468=CARTESIAN_POINT ( 'NONE',  ( -50.79538769728821990, 211.8571965466039444, -6.469044688360768625 ) ) ;
#29495=CARTESIAN_POINT ( 'NONE',  ( -34.76413769728823411, 212.1499508600178387, 3.954877714930865817 ) ) ;
#29499=CARTESIAN_POINT ( 'NONE',  ( -59.70163769728823411, 215.6869285224996986, -3.149950860017881382 ) ) ;
#29500=CARTESIAN_POINT ( 'NONE',  ( -66.62872103062156270, 201.4690446883607819, 2.162041339862843525 ) ) ;
#29505=CARTESIAN_POINT ( 'NONE',  ( -57.51711230271181563, 216.4690446883607535, -1.857196546604089393 ) ) ;
#29513=CARTESIAN_POINT ( 'NONE',  ( -67.81622103062156270, 211.6261429550005744, 6.530955311639228711 ) ) ;
#29553=CARTESIAN_POINT ( 'NONE',  ( -69.20163769728823411, 213.9548777149308592, -2.149950860017830756 ) ) ;
#29590=CARTESIAN_POINT ( 'NONE',  ( -63.85044563604516554, 203.6929966515019430, -6.137860380172892150 ) ) ;
#29594=CARTESIAN_POINT ( 'NONE',  ( -44.25669563604517265, 209.8844732041982297, -4.499999999999996447 ) ) ;
#29600=CARTESIAN_POINT ( 'NONE',  ( -59.70163769728823411, 217.4189793300686233, -4.149950860017907139 ) ) ;
#29634=CARTESIAN_POINT ( 'NONE',  ( -33.56919563604517265, 216.5000000000000000, -0.1155267958017906493 ) ) ;
#29636=CARTESIAN_POINT ( 'NONE',  ( -33.76711230271183695, 214.4690446883608104, -1.321298161741814914 ) ) ;
#29639=CARTESIAN_POINT ( 'NONE',  ( -62.47247103062156981, 207.6499508600178387, 3.839350919129076445 ) ) ;
#29641=CARTESIAN_POINT ( 'NONE',  ( -38.12872103062156270, 201.4690446883607819, 2.162041339862843525 ) ) ;
#29644=CARTESIAN_POINT ( 'NONE',  ( -54.54836230271183695, 202.5810206699313767, -4.149950860017804111 ) ) ;
#29656=CARTESIAN_POINT ( 'NONE',  ( -43.47247103062156981, 206.6499508600178672, 5.571401726697986057 ) ) ;
#29683=CARTESIAN_POINT ( 'NONE',  ( -32.19122103062156270, 208.9097554298617752, -4.530955311639240257 ) ) ;
#29687=CARTESIAN_POINT ( 'NONE',  ( -55.14955436395487709, 214.8429017333601792, -4.673758765035196383 ) ) ;
#29688=CARTESIAN_POINT ( 'NONE',  ( -35.94419563604516554, 201.5000000000000000, 0.1155267958018195706 ) ) ;
#29693=CARTESIAN_POINT ( 'NONE',  ( -61.27752896937850124, 213.3500491399821613, 5.571401726697954970 ) ) ;
#29700=CARTESIAN_POINT ( 'NONE',  ( -63.85788769728821279, 216.4690446883607535, 1.857196546604031662 ) ) ;
#29739=CARTESIAN_POINT ( 'NONE',  ( -69.59747103062156270, 212.3500491399821613, -3.839350919129076445 ) ) ;
#29779=CARTESIAN_POINT ( 'NONE',  ( -67.21502896937850835, 217.3034525342667962, -4.350049139982195001 ) ) ;
#29783=CARTESIAN_POINT ( 'NONE',  ( -49.99627896937850835, 205.4690446883607535, -1.090244570138286351 ) ) ;
#29789=CARTESIAN_POINT ( 'NONE',  ( -52.77455436395490551, 203.6929966515020283, 6.137860380172978303 ) ) ;
#29796=CARTESIAN_POINT ( 'NONE',  ( -34.96205436395489130, 214.6737587650351884, 4.842901733360205796 ) ) ;
#29821=CARTESIAN_POINT ( 'NONE',  ( -43.26711230271183695, 216.4690446883607535, -1.857196546604089393 ) ) ;
#29823=CARTESIAN_POINT ( 'NONE',  ( -61.87127896937849414, 216.5309553116391612, 1.626142955000506873 ) ) ;
#29826=CARTESIAN_POINT ( 'NONE',  ( -45.45163769728823411, 213.9548777149308592, -2.149950860017830756 ) ) ;
#29827=CARTESIAN_POINT ( 'NONE',  ( -69.79538769728823411, 211.8571965466039444, -6.469044688360768625 ) ) ;
#29832=CARTESIAN_POINT ( 'NONE',  ( -40.49627896937850835, 201.4690446883607251, -2.162041339862721845 ) ) ;
#29833=FACE_OUTER_BOUND ( 'NONE', #25653, .T. ) ;
#29842=CARTESIAN_POINT ( 'NONE',  ( -41.69122103062155560, 208.3738570449993404, -6.530955311639226935 ) ) ;
#29873=CARTESIAN_POINT ( 'NONE',  ( -63.45461230271184405, 208.6787018382582346, -4.469044688360757966 ) ) ;
#29877=CARTESIAN_POINT ( 'NONE',  ( -52.57663769728823411, 204.3130714775002730, 3.149950860017883603 ) ) ;
#29878=CARTESIAN_POINT ( 'NONE',  ( -68.01413769728823411, 214.1499508600179240, 7.418979330068584233 ) ) ;
#29885=CARTESIAN_POINT ( 'NONE',  ( -63.65252896937849414, 206.6499508600178387, -5.571401726697954970 ) ) ;
#29893=CARTESIAN_POINT ( 'NONE',  ( -65.63913769728823411, 206.8500491399821044, -5.686928522499717253 ) ) ;
#29897=CARTESIAN_POINT ( 'NONE',  ( -31.99330436395490196, 210.1155267958016850, -8.500000000000003553 ) ) ;
#29947=VERTEX_POINT ( 'NONE', #15439 ) ;
#29970=CARTESIAN_POINT ( 'NONE',  ( -57.12127896937850124, 218.5309553116392465, 2.162041339862725842 ) ) ;
#29973=CARTESIAN_POINT ( 'NONE',  ( -45.04836230271183695, 206.0451222850691977, -2.149950860017851184 ) ) ;
#29980=CARTESIAN_POINT ( 'NONE',  ( -46.24330436395489841, 210.1155267958016850, -8.500000000000003553 ) ) ;
#29988=CARTESIAN_POINT ( 'NONE',  ( -36.34747103062156981, 213.3500491399821328, -5.571401726697985168 ) ) ;
#30013=CARTESIAN_POINT ( 'NONE',  ( -36.73586230271183695, 206.8500491399821328, 5.686928522499748340 ) ) ;
#30014=CARTESIAN_POINT ( 'NONE',  ( -49.40252896937850124, 206.6499508600178387, -5.571401726697954970 ) ) ;
#30018=CARTESIAN_POINT ( 'NONE',  ( -46.83705436395489130, 206.7903428501026042, -3.378800118222489157 ) ) ;
#30019=CARTESIAN_POINT ( 'NONE',  ( -67.22247103062156270, 206.6499508600178672, 5.571401726697986057 ) ) ;
#30023=CARTESIAN_POINT ( 'NONE',  ( -47.02752896937850835, 214.3500491399821897, 7.303452534266821949 ) ) ;
#30034=CARTESIAN_POINT ( 'NONE',  ( -41.49330436395490551, 210.1155267958017134, -6.500000000000000888 ) ) ;
#30062=CARTESIAN_POINT ( 'NONE',  ( -36.74330436395489130, 210.1155267958017703, -4.499999999999996447 ) ) ;
#30066=CARTESIAN_POINT ( 'NONE',  ( -49.01413769728823411, 213.1499508600178672, 5.686928522499718142 ) ) ;
#30067=CARTESIAN_POINT ( 'NONE',  ( -64.64955436395490551, 216.3070033484980002, -6.137860380172975638 ) ) ;
#30072=CARTESIAN_POINT ( 'NONE',  ( -39.30877896937850124, 211.6261429550004607, -6.530955311639245586 ) ) ;
#30080=CARTESIAN_POINT ( 'NONE',  ( -54.15997103062156981, 215.5714017266979852, 3.350049139982118618 ) ) ;
#30086=CARTESIAN_POINT ( 'NONE',  ( -69.59747103062156270, 213.3500491399821328, -5.571401726697985168 ) ) ;
#30162=CARTESIAN_POINT ( 'NONE',  ( -57.91294563604517265, 216.1378603801729241, -6.307003348498026796 ) ) ;
#30166=CARTESIAN_POINT ( 'NONE',  ( -49.00669563604517265, 209.8844732041982297, -4.499999999999996447 ) ) ;
#30172=CARTESIAN_POINT ( 'NONE',  ( -50.00372103062156981, 218.5309553116391896, -2.162041339862839084 ) ) ;
#30202=CARTESIAN_POINT ( 'NONE',  ( -41.28794563604515844, 205.3262412349648116, 4.842901733360249317 ) ) ;
#30203=CARTESIAN_POINT ( 'NONE',  ( -50.59002896937850124, 204.4285982733020433, 3.350049139982171020 ) ) ;
#30207=CARTESIAN_POINT ( 'NONE',  ( -41.69122103062156270, 208.9097554298617752, -4.530955311639240257 ) ) ;
#30208=CARTESIAN_POINT ( 'NONE',  ( -51.98288769728821990, 203.5309553116391612, -1.857196546604028775 ) ) ;
#30214=CARTESIAN_POINT ( 'NONE',  ( -45.64211230271183695, 201.5309553116392181, 2.393094931466368980 ) ) ;
#30226=CARTESIAN_POINT ( 'NONE',  ( -40.89955436395488420, 214.8429017333601792, -4.673758765035196383 ) ) ;
#30253=CARTESIAN_POINT ( 'NONE',  ( -60.48586230271183695, 207.8500491399821613, 3.954877714930852495 ) ) ;
#30258=CARTESIAN_POINT ( 'NONE',  ( -52.18080436395490551, 203.5000000000000000, -0.1155267958017335561 ) ) ;
#30259=CARTESIAN_POINT ( 'NONE',  ( -63.26413769728823411, 214.1499508600179240, 7.418979330068584233 ) ) ;
#30265=CARTESIAN_POINT ( 'NONE',  ( -43.66294563604516554, 214.6737587650350747, -4.842901733360249317 ) ) ;
#30272=CARTESIAN_POINT ( 'NONE',  ( -60.49330436395489841, 210.1155267958017134, -6.500000000000000888 ) ) ;
#30276=CARTESIAN_POINT ( 'NONE',  ( -38.92038769728823411, 207.6069050685337913, 8.469044688360781947 ) ) ;
#30287=CARTESIAN_POINT ( 'NONE',  ( -65.04538769728824832, 211.8571965466039444, -6.469044688360768625 ) ) ;
#30302=CARTESIAN_POINT ( 'NONE',  ( -61.48288769728824121, 205.5309553116392465, -1.321298161741839117 ) ) ;
#30353=CARTESIAN_POINT ( 'NONE',  ( -56.92336230271183695, 217.4189793300686233, 4.149950860017807663 ) ) ;
#30356=CARTESIAN_POINT ( 'NONE',  ( -42.47544563604517265, 213.3788001182224718, 3.209657149897419348 ) ) ;
#30362=CARTESIAN_POINT ( 'NONE',  ( -46.04538769728823411, 212.3930949314662371, -8.469044688360781947 ) ) ;
#30373=AXIS2_PLACEMENT_3D ( 'NONE', #13733, #4994, #25092 ) ;
#30385=DIRECTION ( 'NONE',  ( -0.9933043639548644332, 0.1155267958017622554, 0.000000000000000000 ) ) ;
#30392=CARTESIAN_POINT ( 'NONE',  ( -34.75669563604516554, 209.8844732041982013, -6.500000000000000888 ) ) ;
#30393=CARTESIAN_POINT ( 'NONE',  ( -54.54836230271182984, 204.3130714775002446, -3.149950860017828091 ) ) ;
#30398=CARTESIAN_POINT ( 'NONE',  ( -47.43080436395489841, 205.4999999999999716, -0.1155267958017894420 ) ) ;
#30399=CARTESIAN_POINT ( 'NONE',  ( -60.29538769728823411, 211.8571965466039444, -6.469044688360768625 ) ) ;
#30404=CARTESIAN_POINT ( 'NONE',  ( -43.06919563604516554, 218.5000000000000000, -0.1155267958018185298 ) ) ;
#30416=CARTESIAN_POINT ( 'NONE',  ( -33.57663769728823411, 204.3130714775002730, 3.149950860017883603 ) ) ;
#30448=CARTESIAN_POINT ( 'NONE',  ( -58.70461230271184405, 208.6787018382582346, -4.469044688360757966 ) ) ;
#30453=CARTESIAN_POINT ( 'NONE',  ( -51.98288769728821990, 203.5309553116391612, -1.857196546604028775 ) ) ;
#30454=CARTESIAN_POINT ( 'NONE',  ( -56.93080436395490551, 201.5000000000000000, -0.1155267958017054536 ) ) ;
#30460=CARTESIAN_POINT ( 'NONE',  ( -44.05877896937847993, 211.6261429550004607, -6.530955311639245586 ) ) ;
#30467=CARTESIAN_POINT ( 'NONE',  ( -55.54538769728823411, 211.8571965466040012, -6.469044688360769513 ) ) ;
#30471=CARTESIAN_POINT ( 'NONE',  ( -40.10788769728823411, 218.4690446883607535, 2.393094931466250408 ) ) ;
#30496=CARTESIAN_POINT ( 'NONE',  ( -52.97247103062156270, 207.6499508600178387, 3.839350919129076445 ) ) ;
#30545=CARTESIAN_POINT ( 'NONE',  ( -31.00000000000003553, 209.9999999999999716, -6.500000000000000888 ) ) ;
#30547=CARTESIAN_POINT ( 'NONE',  ( -54.94419563604517265, 201.5000000000000000, 0.1155267958018195706 ) ) ;
#30551=CARTESIAN_POINT ( 'NONE',  ( -32.97544563604516554, 213.3788001182224718, 3.209657149897419348 ) ) ;
#30588=CARTESIAN_POINT ( 'NONE',  ( -60.28794563604516554, 205.3262412349647832, 4.842901733360250205 ) ) ;
#30591=CARTESIAN_POINT ( 'NONE',  ( -48.22247103062156981, 207.6499508600178387, 3.839350919129076445 ) ) ;
#30592=CARTESIAN_POINT ( 'NONE',  ( -63.65997103062156981, 215.5714017266979852, 3.350049139982118618 ) ) ;
#30596=CARTESIAN_POINT ( 'NONE',  ( -44.25669563604517265, 209.8844732041981729, -8.500000000000003553 ) ) ;
#30632=CARTESIAN_POINT ( 'NONE',  ( -62.46502896937850124, 215.5714017266979567, -3.350049139982168800 ) ) ;
#30634=CARTESIAN_POINT ( 'NONE',  ( -59.10044563604517265, 206.6211998817775566, -3.209657149897419348 ) ) ;
#30637=CARTESIAN_POINT ( 'NONE',  ( -47.03497103062156981, 204.4285982733020148, -3.350049139982115509 ) ) ;
#30638=CARTESIAN_POINT ( 'NONE',  ( -53.17038769728823411, 207.6069050685337913, 8.469044688360781947 ) ) ;
#30643=CARTESIAN_POINT ( 'NONE',  ( -40.89211230271181563, 203.5309553116391612, 1.857196546604092280 ) ) ;
#30653=CARTESIAN_POINT ( 'NONE',  ( -55.14955436395489130, 214.8429017333601792, -4.673758765035197271 ) ) ;
#30657=CARTESIAN_POINT ( 'NONE',  ( -69.99330436395490551, 210.1155267958017134, -6.500000000000000888 ) ) ;
#30680=CARTESIAN_POINT ( 'NONE',  ( -58.90997103062156981, 213.8393509191290889, 2.350049139982164359 ) ) ;
#30728=CARTESIAN_POINT ( 'NONE',  ( -59.10044563604517265, 203.6929966515019430, -6.137860380172892150 ) ) ;
#30733=CARTESIAN_POINT ( 'NONE',  ( -65.43377896937850835, 208.3738570449995109, 6.530955311639247363 ) ) ;
#30767=CARTESIAN_POINT ( 'NONE',  ( -59.89211230271182984, 203.5309553116391612, 1.857196546604092280 ) ) ;
#30771=CARTESIAN_POINT ( 'NONE',  ( -67.21502896937850835, 213.8393509191290889, -2.350049139982142155 ) ) ;
#30772=CARTESIAN_POINT ( 'NONE',  ( -54.75372103062154849, 216.5309553116391612, -1.626142955000564383 ) ) ;
#30775=CARTESIAN_POINT ( 'NONE',  ( -35.54836230271182984, 202.5810206699313767, -4.149950860017804111 ) ) ;
#30813=CARTESIAN_POINT ( 'NONE',  ( -58.90252896937850124, 206.6499508600178387, -5.571401726697954970 ) ) ;
#30815=CARTESIAN_POINT ( 'NONE',  ( -53.16294563604516554, 213.2096571498974527, -3.378800118222469617 ) ) ;
#30818=CARTESIAN_POINT ( 'NONE',  ( -68.01413769728823411, 212.1499508600178387, 3.954877714930865817 ) ) ;
#30819=CARTESIAN_POINT ( 'NONE',  ( -63.46205436395489841, 216.1378603801730094, 6.307003348497944195 ) ) ;
#30825=CARTESIAN_POINT ( 'NONE',  ( -46.82961230271183695, 211.8571965466040297, 6.469044688360755302 ) ) ;
#30833=CARTESIAN_POINT ( 'NONE',  ( -54.55580436395489841, 216.5000000000000000, 0.1155267958017343610 ) ) ;
#30837=CARTESIAN_POINT ( 'NONE',  ( -58.90997103062156270, 215.5714017266979852, 3.350049139982118618 ) ) ;
#30861=CARTESIAN_POINT ( 'NONE',  ( -56.53497103062156270, 206.1606490808709111, -2.350049139982163027 ) ) ;
#30911=CARTESIAN_POINT ( 'NONE',  ( -45.44419563604516554, 201.5000000000000000, 0.1155267958018195706 ) ) ;
#30914=CARTESIAN_POINT ( 'NONE',  ( -32.57961230271184405, 211.3212981617417938, 4.469044688360757966 ) ) ;
#30919=CARTESIAN_POINT ( 'NONE',  ( -49.80580436395490551, 216.5000000000000000, 0.1155267958017343610 ) ) ;
#30954=CARTESIAN_POINT ( 'NONE',  ( -47.42336230271183695, 215.6869285224997270, 3.149950860017831200 ) ) ;
#30958=CARTESIAN_POINT ( 'NONE',  ( -65.23586230271183695, 207.8500491399821613, 3.954877714930852495 ) ) ;
#30959=CARTESIAN_POINT ( 'NONE',  ( -52.57663769728823411, 204.3130714775002730, 3.149950860017883603 ) ) ;
#30963=CARTESIAN_POINT ( 'NONE',  ( -69.00372103062157692, 218.5309553116391896, -2.162041339862839084 ) ) ;
#31002=CARTESIAN_POINT ( 'NONE',  ( -67.80877896937849414, 211.6261429550004891, -6.530955311639245586 ) ) ;
#31004=CARTESIAN_POINT ( 'NONE',  ( -45.24627896937850835, 205.4690446883607535, -1.090244570138286351 ) ) ;
#31008=CARTESIAN_POINT ( 'NONE',  ( -66.43080436395490551, 205.4999999999999716, -0.1155267958017894420 ) ) ;
#31009=CARTESIAN_POINT ( 'NONE',  ( -62.27455436395490551, 203.6929966515020283, 6.137860380172978303 ) ) ;
#31013=CARTESIAN_POINT ( 'NONE',  ( -66.42336230271182274, 217.4189793300686233, 4.149950860017807663 ) ) ;
#31020=CARTESIAN_POINT ( 'NONE',  ( -44.46205436395489130, 214.6737587650351884, 4.842901733360205796 ) ) ;
#31025=CARTESIAN_POINT ( 'NONE',  ( -57.12872103062157692, 203.4690446883607535, 1.626142955000567936 ) ) ;
#31051=CARTESIAN_POINT ( 'NONE',  ( -54.15997103062156981, 213.8393509191290889, 2.350049139982164359 ) ) ;
#31054=CARTESIAN_POINT ( 'NONE',  ( -67.02455436395489130, 205.1570982666397356, 4.673758765035198159 ) ) ;
#31099=CARTESIAN_POINT ( 'NONE',  ( -44.05877896937850124, 212.1620413398627534, -8.530955311639255356 ) ) ;
#31102=CARTESIAN_POINT ( 'NONE',  ( -32.38169563604516554, 210.1155267958017703, 4.499999999999996447 ) ) ;
#31107=CARTESIAN_POINT ( 'NONE',  ( -42.08705436395489841, 205.3262412349647263, -4.842901733360204020 ) ) ;
#31138=CARTESIAN_POINT ( 'NONE',  ( -43.26711230271183695, 216.4690446883607535, -1.857196546604089393 ) ) ;
#31142=CARTESIAN_POINT ( 'NONE',  ( -39.90997103062156270, 213.8393509191290889, 2.350049139982164359 ) ) ;
#31143=CARTESIAN_POINT ( 'NONE',  ( -44.46205436395488420, 214.6737587650352168, 4.842901733360204908 ) ) ;
#31149=CARTESIAN_POINT ( 'NONE',  ( -35.74627896937850124, 201.4690446883607251, -2.162041339862721845 ) ) ;
#31167=CARTESIAN_POINT ( 'NONE',  ( -68.21205436395489130, 214.6737587650352168, 4.842901733360204908 ) ) ;
#31184=CARTESIAN_POINT ( 'NONE',  ( -67.41294563604516554, 214.6737587650350747, -4.842901733360248429 ) ) ;
#31186=CARTESIAN_POINT ( 'NONE',  ( -48.01711230271184405, 214.4690446883608104, -1.321298161741814914 ) ) ;
#31190=CARTESIAN_POINT ( 'NONE',  ( -35.35788769728823411, 216.4690446883607535, 1.857196546604031662 ) ) ;
#31191=CARTESIAN_POINT ( 'NONE',  ( -41.49330436395490551, 210.1155267958016850, -8.500000000000003553 ) ) ;
#31195=CARTESIAN_POINT ( 'NONE',  ( -66.81919563604516554, 218.5000000000000000, -0.1155267958018185298 ) ) ;
#31206=CARTESIAN_POINT ( 'NONE',  ( -63.06622103062156981, 211.6261429550005744, 6.530955311639227823 ) ) ;
#31231=CARTESIAN_POINT ( 'NONE',  ( -49.80580436395490551, 214.5000000000000284, 0.1155267958017899832 ) ) ;
#31279=CARTESIAN_POINT ( 'NONE',  ( -46.23586230271182984, 205.8500491399821613, 7.418979330068642852 ) ) ;
#31282=CARTESIAN_POINT ( 'NONE',  ( -30.79836230271183339, 206.0451222850691977, -2.149950860017851184 ) ) ;
#31286=CARTESIAN_POINT ( 'NONE',  ( -43.86830436395490551, 209.8844732041982581, 6.500000000000000888 ) ) ;
#31317=CARTESIAN_POINT ( 'NONE',  ( -40.69419563604516554, 203.5000000000000000, 0.1155267958017914542 ) ) ;
#31319=SURFACE_STYLE_FILL_AREA ( #218 ) ;
#31321=CARTESIAN_POINT ( 'NONE',  ( -38.12872103062156270, 205.4690446883607535, 1.090244570138264368 ) ) ;
#31322=CARTESIAN_POINT ( 'NONE',  ( -48.02455436395488420, 205.1570982666397356, 4.673758765035198159 ) ) ;
#31327=CARTESIAN_POINT ( 'NONE',  ( -68.01413769728823411, 214.1499508600179240, 7.418979330068584233 ) ) ;
#31344=CARTESIAN_POINT ( 'NONE',  ( -67.61830436395489130, 209.8844732041982581, 6.500000000000000888 ) ) ;
#31363=CARTESIAN_POINT ( 'NONE',  ( -62.06919563604516554, 216.5000000000000000, -0.1155267958017906493 ) ) ;
#31366=CARTESIAN_POINT ( 'NONE',  ( -40.10044563604517265, 206.6211998817775566, -3.209657149897419348 ) ) ;
#31370=CARTESIAN_POINT ( 'NONE',  ( -37.33705436395490551, 205.3262412349647263, -4.842901733360204020 ) ) ;
#31371=CARTESIAN_POINT ( 'NONE',  ( -48.22247103062156981, 205.6499508600178956, 7.303452534266880569 ) ) ;
#31378=CARTESIAN_POINT ( 'NONE',  ( -37.92336230271182984, 215.6869285224997270, 3.149950860017831200 ) ) ;
#31390=CARTESIAN_POINT ( 'NONE',  ( -63.26413769728824121, 213.1499508600178672, 5.686928522499718142 ) ) ;
#31399=EDGE_LOOP ( 'NONE', ( #34166, #23364, #36340, #8928 ) ) ;
#31416=CARTESIAN_POINT ( 'NONE',  ( -47.23288769728824121, 205.5309553116392465, -1.321298161741839117 ) ) ;
#31421=CARTESIAN_POINT ( 'NONE',  ( -68.40997103062156270, 215.5714017266979852, 3.350049139982118618 ) ) ;
#31463=CARTESIAN_POINT ( 'NONE',  ( -55.14211230271182274, 203.5309553116391612, 1.857196546604092280 ) ) ;
#31466=CARTESIAN_POINT ( 'NONE',  ( -50.00372103062157692, 216.5309553116391612, -1.626142955000564383 ) ) ;
#31497=PRODUCT_DEFINITION ( 'UNKNOWN', '', #25071, #17984 ) ;
#31500=CARTESIAN_POINT ( 'NONE',  ( -45.64211230271183695, 203.5309553116391612, 1.857196546604092280 ) ) ;
#31504=CARTESIAN_POINT ( 'NONE',  ( -37.33705436395491262, 206.7903428501026042, -3.378800118222489157 ) ) ;
#31505=CARTESIAN_POINT ( 'NONE',  ( -48.61830436395490551, 209.8844732041982581, 6.500000000000000888 ) ) ;
#31510=CARTESIAN_POINT ( 'NONE',  ( -37.52752896937849414, 214.3500491399821897, 7.303452534266821949 ) ) ;
#31528=CARTESIAN_POINT ( 'NONE',  ( -63.46205436395489841, 214.6737587650352168, 4.842901733360204908 ) ) ;
#31546=CARTESIAN_POINT ( 'NONE',  ( -56.32961230271183695, 211.8571965466040581, 6.469044688360755302 ) ) ;
#31549=CARTESIAN_POINT ( 'NONE',  ( -47.62127896937850124, 214.5309553116392749, 1.090244570138288127 ) ) ;
#31553=CARTESIAN_POINT ( 'NONE',  ( -38.72247103062156981, 206.6499508600178672, 5.571401726697986057 ) ) ;
#31554=CARTESIAN_POINT ( 'NONE',  ( -50.00372103062156981, 218.5309553116391896, -2.162041339862839084 ) ) ;
#31558=CARTESIAN_POINT ( 'NONE',  ( -31.98586230271182984, 206.8500491399821328, 5.686928522499748340 ) ) ;
#31570=CARTESIAN_POINT ( 'NONE',  ( -68.01413769728823411, 213.1499508600178672, 5.686928522499718142 ) ) ;
#31597=CARTESIAN_POINT ( 'NONE',  ( -41.88913769728823411, 207.8500491399821613, -3.954877714930864485 ) ) ;
#31601=CARTESIAN_POINT ( 'NONE',  ( -68.60788769728823411, 216.4690446883607535, 1.857196546604031662 ) ) ;
#31650=CARTESIAN_POINT ( 'NONE',  ( -48.81622103062156270, 211.6261429550005744, 6.530955311639227823 ) ) ;
#31683=CARTESIAN_POINT ( 'NONE',  ( -36.53794563604517265, 205.3262412349647832, 4.842901733360250205 ) ) ;
#31687=CARTESIAN_POINT ( 'NONE',  ( -52.96502896937850124, 213.8393509191290889, -2.350049139982142155 ) ) ;
#31688=CARTESIAN_POINT ( 'NONE',  ( -46.63913769728824121, 206.8500491399821044, -5.686928522499717253 ) ) ;
#31694=CARTESIAN_POINT ( 'NONE',  ( -57.12872103062156270, 201.4690446883607819, 2.162041339862843525 ) ) ;
#31702=CARTESIAN_POINT ( 'NONE',  ( -39.51413769728823411, 213.1499508600178672, 5.686928522499718142 ) ) ;
#31714=CARTESIAN_POINT ( 'NONE',  ( -51.58705436395488420, 205.3262412349647263, -4.842901733360204020 ) ) ;
#31734=CARTESIAN_POINT ( 'NONE',  ( -53.75669563604516554, 209.8844732041982013, -6.500000000000000888 ) ) ;
#31736=CARTESIAN_POINT ( 'NONE',  ( -40.29836230271183695, 206.0451222850691977, -2.149950860017851184 ) ) ;
#31739=CARTESIAN_POINT ( 'NONE',  ( -57.32663769728824121, 206.0451222850691408, 2.149950860017832532 ) ) ;
#31741=CARTESIAN_POINT ( 'NONE',  ( -45.45163769728823411, 217.4189793300686233, -4.149950860017907139 ) ) ;
#31745=CARTESIAN_POINT ( 'NONE',  ( -34.75669563604516554, 209.8844732041982013, -6.500000000000000888 ) ) ;
#31755=CARTESIAN_POINT ( 'NONE',  ( -52.37872103062156270, 203.4690446883607535, 1.626142955000567936 ) ) ;
#31777=CARTESIAN_POINT ( 'NONE',  ( -44.85788769728823411, 214.4690446883608104, 1.321298161741840893 ) ) ;
#31833=CARTESIAN_POINT ( 'NONE',  ( -35.95163769728823411, 215.6869285224996986, -3.149950860017881382 ) ) ;
#31869=CARTESIAN_POINT ( 'NONE',  ( -64.44419563604517975, 201.5000000000000000, 0.1155267958018195706 ) ) ;
#31871=( NAMED_UNIT ( * ) PLANE_ANGLE_UNIT ( ) SI_UNIT ( $, .RADIAN. ) );
#31875=CARTESIAN_POINT ( 'NONE',  ( -60.48586230271183695, 207.8500491399821613, 3.954877714930852495 ) ) ;
#31876=CARTESIAN_POINT ( 'NONE',  ( -50.79538769728821990, 211.8571965466039444, -6.469044688360768625 ) ) ;
#31882=CARTESIAN_POINT ( 'NONE',  ( -58.11830436395491262, 209.8844732041983150, 8.500000000000003553 ) ) ;
#31887=CARTESIAN_POINT ( 'NONE',  ( -37.73288769728822700, 203.5309553116391896, -1.857196546604028997 ) ) ;
#31899=CARTESIAN_POINT ( 'NONE',  ( -59.30580436395489841, 216.5000000000000000, 0.1155267958017343610 ) ) ;
#31918=CARTESIAN_POINT ( 'NONE',  ( -52.76711230271182984, 216.4690446883607535, -1.857196546604089393 ) ) ;
#31920=CARTESIAN_POINT ( 'NONE',  ( -33.96502896937850124, 213.8393509191290889, -2.350049139982142155 ) ) ;
#31923=CARTESIAN_POINT ( 'NONE',  ( -65.04538769728823411, 211.3212981617418222, -4.469044688360751749 ) ) ;
#31924=CARTESIAN_POINT ( 'NONE',  ( -45.25372103062157692, 218.5309553116391896, -2.162041339862839084 ) ) ;
#31928=CARTESIAN_POINT ( 'NONE',  ( -57.12127896937850124, 218.5309553116392465, 2.162041339862725842 ) ) ;
#31939=CARTESIAN_POINT ( 'NONE',  ( -55.54538769728823411, 211.8571965466039444, -6.469044688360768625 ) ) ;
#31969=CARTESIAN_POINT ( 'NONE',  ( -38.72247103062156981, 207.6499508600178387, 3.839350919129076445 ) ) ;
#31973=CARTESIAN_POINT ( 'NONE',  ( -61.28497103062156981, 204.4285982733020148, -3.350049139982115509 ) ) ;
#31974=CARTESIAN_POINT ( 'NONE',  ( -44.25669563604517265, 209.8844732041981729, -8.500000000000003553 ) ) ;
#32018=CARTESIAN_POINT ( 'NONE',  ( -64.45163769728823411, 213.9548777149308592, -2.149950860017830756 ) ) ;
#32057=CARTESIAN_POINT ( 'NONE',  ( -31.59002896937850124, 204.4285982733020433, 3.350049139982171020 ) ) ;
#32060=CARTESIAN_POINT ( 'NONE',  ( -64.24627896937850835, 205.4690446883607535, -1.090244570138286351 ) ) ;
#32064=ORIENTED_EDGE ( 'NONE', *, *, #19616, .T. ) ;
#32068=CARTESIAN_POINT ( 'NONE',  ( -61.28497103062156981, 202.6965474657331185, -4.350049139982091084 ) ) ;
#32073=CARTESIAN_POINT ( 'NONE',  ( -43.27455436395489841, 205.1570982666397640, 4.673758765035199048 ) ) ;
#32086=CARTESIAN_POINT ( 'NONE',  ( -54.75372103062154849, 216.5309553116391612, -1.626142955000564383 ) ) ;
#32102=CARTESIAN_POINT ( 'NONE',  ( -47.02752896937850124, 213.3500491399821613, 5.571401726697954970 ) ) ;
#32103=CARTESIAN_POINT ( 'NONE',  ( -35.35044563604517265, 206.6211998817775566, -3.209657149897419348 ) ) ;
#32106=CARTESIAN_POINT ( 'NONE',  ( -61.68080436395489841, 205.4999999999999716, -0.1155267958017894420 ) ) ;
#32107=CARTESIAN_POINT ( 'NONE',  ( -35.35788769728823411, 218.4690446883607535, 2.393094931466250408 ) ) ;
#32111=CARTESIAN_POINT ( 'NONE',  ( -52.76711230271184405, 218.4690446883607535, -2.393094931466363651 ) ) ;
#32124=CARTESIAN_POINT ( 'NONE',  ( -44.26413769728823411, 213.1499508600178672, 5.686928522499718142 ) ) ;
#32150=CARTESIAN_POINT ( 'NONE',  ( -63.85044563604516554, 206.6211998817775566, -3.209657149897419348 ) ) ;
#32154=CARTESIAN_POINT ( 'NONE',  ( -62.27455436395490551, 205.1570982666397356, 4.673758765035198159 ) ) ;
#32155=CARTESIAN_POINT ( 'NONE',  ( -34.36086230271182984, 214.1499508600178387, -7.418979330068641964 ) ) ;
#32160=CARTESIAN_POINT ( 'NONE',  ( -55.73586230271182984, 206.8500491399821328, 5.686928522499748340 ) ) ;
#32170=CARTESIAN_POINT ( 'NONE',  ( -66.62872103062154849, 203.4690446883607535, 1.626142955000567936 ) ) ;
#32210=CARTESIAN_POINT ( 'NONE',  ( -67.61830436395490551, 209.8844732041982297, 4.499999999999996447 ) ) ;
#32227=DIRECTION ( 'NONE',  ( -0.1155267958017759666, -0.9933043639548629899, 2.756973438308332598E-14 ) ) ;
#32243=CARTESIAN_POINT ( 'NONE',  ( -35.54836230271183695, 204.3130714775002446, -3.149950860017828091 ) ) ;
#32246=CARTESIAN_POINT ( 'NONE',  ( -56.92336230271183695, 213.9548777149308023, 2.149950860017852960 ) ) ;
#32247=CARTESIAN_POINT ( 'NONE',  ( -35.55580436395490551, 216.5000000000000000, 0.1155267958017343610 ) ) ;
#32252=CARTESIAN_POINT ( 'NONE',  ( -61.48288769728824121, 201.5309553116392181, -2.393094931466246855 ) ) ;
#32258=CARTESIAN_POINT ( 'NONE',  ( -40.50372103062156981, 216.5309553116392181, -1.626142955000564383 ) ) ;
#32266=CARTESIAN_POINT ( 'NONE',  ( -30.00669563604516910, 209.8844732041982013, -6.500000000000000888 ) ) ;
#32271=CARTESIAN_POINT ( 'NONE',  ( -58.71205436395488420, 214.6737587650352168, 4.842901733360204908 ) ) ;
#32288=CARTESIAN_POINT ( 'NONE',  ( -55.53794563604516554, 205.3262412349648116, 4.842901733360249317 ) ) ;
#32290=CARTESIAN_POINT ( 'NONE',  ( -32.18377896937850124, 208.9097554298617183, 4.530955311639234040 ) ) ;
#32295=CARTESIAN_POINT ( 'NONE',  ( -55.94122103062156981, 208.9097554298617752, -4.530955311639240257 ) ) ;
#32297=CARTESIAN_POINT ( 'NONE',  ( -66.23288769728823411, 203.5309553116391612, -1.857196546604028775 ) ) ;
#32301=CARTESIAN_POINT ( 'NONE',  ( -59.89211230271182274, 201.5309553116392181, 2.393094931466368980 ) ) ;
#32312=CARTESIAN_POINT ( 'NONE',  ( -53.17038769728823411, 208.1428034533959703, 6.469044688360770401 ) ) ;
#32339=CARTESIAN_POINT ( 'NONE',  ( -31.99330436395490196, 210.1155267958017703, -4.499999999999996447 ) ) ;
#32344=CARTESIAN_POINT ( 'NONE',  ( -63.26413769728824121, 213.1499508600178672, 5.686928522499718142 ) ) ;
#32345=CARTESIAN_POINT ( 'NONE',  ( -32.77752896937849414, 214.3500491399821897, 7.303452534266821949 ) ) ;
#32350=CARTESIAN_POINT ( 'NONE',  ( -60.09002896937850124, 204.4285982733020433, 3.350049139982171020 ) ) ;
#32396=CARTESIAN_POINT ( 'NONE',  ( -32.78497103062156981, 204.4285982733020148, -3.350049139982115509 ) ) ;
#32433=CARTESIAN_POINT ( 'NONE',  ( -64.24627896937850835, 201.4690446883607251, -2.162041339862721845 ) ) ;
#32436=CARTESIAN_POINT ( 'NONE',  ( -62.86086230271182984, 212.1499508600178387, -3.954877714930852495 ) ) ;
#32437=CARTESIAN_POINT ( 'NONE',  ( -34.56622103062155560, 211.6261429550005744, 6.530955311639227823 ) ) ;
#32442=CARTESIAN_POINT ( 'NONE',  ( -56.53497103062156270, 202.6965474657331185, -4.350049139982091084 ) ) ;
#32473=CARTESIAN_POINT ( 'NONE',  ( -42.67336230271183695, 215.6869285224997270, 3.149950860017831200 ) ) ;
#32474=CARTESIAN_POINT ( 'NONE',  ( -64.44419563604516554, 203.5000000000000000, 0.1155267958017914542 ) ) ;
#32478=CARTESIAN_POINT ( 'NONE',  ( -56.33705436395490551, 206.7903428501026042, -3.378800118222489157 ) ) ;
#32479=CARTESIAN_POINT ( 'NONE',  ( -32.78497103062156981, 202.6965474657331185, -4.350049139982091084 ) ) ;
#32483=CARTESIAN_POINT ( 'NONE',  ( -57.91294563604517265, 216.1378603801729241, -6.307003348498026796 ) ) ;
#32494=CARTESIAN_POINT ( 'NONE',  ( -39.51413769728823411, 213.1499508600178672, 5.686928522499718142 ) ) ;
#32523=CARTESIAN_POINT ( 'NONE',  ( -68.00669563604516554, 209.8844732041982297, -4.499999999999996447 ) ) ;
#32528=CARTESIAN_POINT ( 'NONE',  ( -58.31622103062155560, 211.6261429550005744, 6.530955311639227823 ) ) ;
#32529=CARTESIAN_POINT ( 'NONE',  ( -35.15252896937850124, 205.6499508600178103, -7.303452534266820173 ) ) ;
#32536=CARTESIAN_POINT ( 'NONE',  ( -59.89211230271182984, 203.5309553116391612, 1.857196546604092280 ) ) ;
#32542=CARTESIAN_POINT ( 'NONE',  ( -62.86830436395490551, 209.8844732041982581, 6.500000000000000888 ) ) ;
#32583=CARTESIAN_POINT ( 'NONE',  ( -66.62872103062156270, 205.4690446883607535, 1.090244570138264368 ) ) ;
#32623=CARTESIAN_POINT ( 'NONE',  ( -30.99627896937850124, 203.4690446883607535, -1.626142955000504209 ) ) ;
#32627=CARTESIAN_POINT ( 'NONE',  ( -41.68377896937850124, 208.9097554298617183, 4.530955311639234040 ) ) ;
#32633=CARTESIAN_POINT ( 'NONE',  ( -45.84747103062156981, 214.3500491399821044, -7.303452534266878793 ) ) ;
#32639=CARTESIAN_POINT ( 'NONE',  ( -34.76413769728823411, 213.1499508600178672, 5.686928522499718142 ) ) ;
#32664=CARTESIAN_POINT ( 'NONE',  ( -32.38169563604517265, 210.1155267958017703, 6.500000000000000888 ) ) ;
#32666=CARTESIAN_POINT ( 'NONE',  ( -62.46502896937850124, 215.5714017266979567, -3.350049139982168800 ) ) ;
#32669=CARTESIAN_POINT ( 'NONE',  ( -46.63913769728824121, 207.8500491399821613, -3.954877714930864485 ) ) ;
#32670=CARTESIAN_POINT ( 'NONE',  ( -32.19122103062156270, 207.8379586601371329, -8.530955311639223382 ) ) ;
#32674=CARTESIAN_POINT ( 'NONE',  ( -56.32961230271183695, 212.3930949314663792, 8.469044688360751749 ) ) ;
#32685=CARTESIAN_POINT ( 'NONE',  ( -39.31622103062156270, 211.6261429550005744, 6.530955311639227823 ) ) ;
#32714=CARTESIAN_POINT ( 'NONE',  ( -64.24627896937850835, 205.4690446883607535, -1.090244570138286351 ) ) ;
#32718=CARTESIAN_POINT ( 'NONE',  ( -45.05580436395489841, 216.5000000000000000, 0.1155267958017343610 ) ) ;
#32720=CARTESIAN_POINT ( 'NONE',  ( -68.21205436395490551, 216.1378603801730094, 6.307003348497944195 ) ) ;
#32726=CARTESIAN_POINT ( 'NONE',  ( -62.86086230271182984, 213.1499508600178387, -5.686928522499747451 ) ) ;
#32738=CARTESIAN_POINT ( 'NONE',  ( -43.27455436395490551, 203.6929966515020283, 6.137860380172978303 ) ) ;
#32810=CARTESIAN_POINT ( 'NONE',  ( -60.09002896937850124, 202.6965474657332038, 4.350049139982197666 ) ) ;
#32813=CARTESIAN_POINT ( 'NONE',  ( -48.41294563604517265, 213.2096571498974527, -3.378800118222469617 ) ) ;
#32819=CARTESIAN_POINT ( 'NONE',  ( -44.65997103062156981, 217.3034525342668815, 4.350049139982096413 ) ) ;
#32826=CARTESIAN_POINT ( 'NONE',  ( -34.17038769728823411, 208.1428034533959703, 6.469044688360771289 ) ) ;
#32850=CARTESIAN_POINT ( 'NONE',  ( -35.54836230271183695, 204.3130714775002446, -3.149950860017828091 ) ) ;
#32851=CARTESIAN_POINT ( 'NONE',  ( -61.27752896937850124, 213.3500491399821613, 5.571401726697954970 ) ) ;
#32856=CARTESIAN_POINT ( 'NONE',  ( -43.27455436395490551, 206.6211998817774997, 3.209657149897401585 ) ) ;
#32857=CARTESIAN_POINT ( 'NONE',  ( -68.01413769728823411, 213.1499508600178672, 5.686928522499718142 ) ) ;
#32860=( GEOMETRIC_REPRESENTATION_CONTEXT ( 3 ) GLOBAL_UNCERTAINTY_ASSIGNED_CONTEXT ( ( #26571 ) ) GLOBAL_UNIT_ASSIGNED_CONTEXT ( ( #37252, #36700, #28172 ) ) REPRESENTATION_CONTEXT ( 'NONE', 'WORKASPACE' ) );
#32864=CARTESIAN_POINT ( 'NONE',  ( -42.07961230271182984, 212.3930949314663792, 8.469044688360751749 ) ) ;
#32876=CARTESIAN_POINT ( 'NONE',  ( -35.55580436395490551, 216.5000000000000000, 0.1155267958017343610 ) ) ;
#32902=CARTESIAN_POINT ( 'NONE',  ( -61.87127896937851546, 214.5309553116392749, 1.090244570138288127 ) ) ;
#32906=CARTESIAN_POINT ( 'NONE',  ( -44.26413769728823411, 213.1499508600178672, 5.686928522499718142 ) ) ;
#32907=CARTESIAN_POINT ( 'NONE',  ( -31.39211230271183339, 201.5309553116392181, 2.393094931466368980 ) ) ;
#32912=CARTESIAN_POINT ( 'NONE',  ( -45.24627896937850835, 203.4690446883607535, -1.626142955000504209 ) ) ;
#32921=CARTESIAN_POINT ( 'NONE',  ( -60.29538769728823411, 211.8571965466040012, -6.469044688360769513 ) ) ;
#32925=CARTESIAN_POINT ( 'NONE',  ( -35.55580436395489130, 218.5000000000000000, 0.1155267958017064944 ) ) ;
#33001=CARTESIAN_POINT ( 'NONE',  ( -50.39211230271182984, 201.5309553116392181, 2.393094931466368980 ) ) ;
#33005=CARTESIAN_POINT ( 'NONE',  ( -43.66294563604516554, 213.2096571498974527, -3.378800118222469617 ) ) ;
#33012=CARTESIAN_POINT ( 'NONE',  ( -43.67038769728823411, 207.6069050685337913, 8.469044688360781947 ) ) ;
#33046=CARTESIAN_POINT ( 'NONE',  ( -42.87127896937850124, 216.5309553116392181, 1.626142955000506429 ) ) ;
#33047=CARTESIAN_POINT ( 'NONE',  ( -52.76711230271183695, 216.4690446883607535, -1.857196546604089393 ) ) ;
#33051=CARTESIAN_POINT ( 'NONE',  ( -44.46205436395490551, 213.2096571498974242, 3.378800118222489601 ) ) ;
#33052=CARTESIAN_POINT ( 'NONE',  ( -63.06622103062156981, 211.6261429550005744, 6.530955311639227823 ) ) ;
#33056=CARTESIAN_POINT ( 'NONE',  ( -41.28794563604517265, 203.8621396198271043, 6.307003348498029460 ) ) ;
#33070=CARTESIAN_POINT ( 'NONE',  ( -36.94122103062157692, 208.3738570449993404, -6.530955311639226935 ) ) ;
#33097=CARTESIAN_POINT ( 'NONE',  ( -49.00669563604517265, 209.8844732041982297, -4.499999999999996447 ) ) ;
#33101=CARTESIAN_POINT ( 'NONE',  ( -50.79538769728821990, 211.8571965466039444, -6.469044688360768625 ) ) ;
#33102=CARTESIAN_POINT ( 'NONE',  ( -53.96205436395491262, 216.1378603801730094, 6.307003348497944195 ) ) ;
#33106=CARTESIAN_POINT ( 'NONE',  ( -50.19419563604517265, 203.5000000000000000, 0.1155267958017914542 ) ) ;
#33113=CARTESIAN_POINT ( 'NONE',  ( -58.90997103062156270, 215.5714017266979852, 3.350049139982118618 ) ) ;
#33116=EDGE_CURVE ( 'NONE', #14550, #33325, #35349, .T. ) ;
#33118=CARTESIAN_POINT ( 'NONE',  ( -35.75372103062156981, 218.5309553116391896, -2.162041339862839084 ) ) ;
#33146=CARTESIAN_POINT ( 'NONE',  ( -51.98288769728823411, 205.5309553116392465, -1.321298161741839117 ) ) ;
#33192=CARTESIAN_POINT ( 'NONE',  ( -58.30877896937849414, 212.1620413398627534, -8.530955311639255356 ) ) ;
#33197=CARTESIAN_POINT ( 'NONE',  ( -51.57961230271184405, 211.3212981617417938, 4.469044688360757966 ) ) ;
#33204=CARTESIAN_POINT ( 'NONE',  ( -51.19122103062157692, 207.8379586601371329, -8.530955311639223382 ) ) ;
#33228=ADVANCED_FACE ( 'NONE', ( #34262 ), #1096, .T. ) ;
#33233=CARTESIAN_POINT ( 'NONE',  ( -41.68377896937850124, 208.3738570449995109, 6.530955311639247363 ) ) ;
#33234=CARTESIAN_POINT ( 'NONE',  ( -52.56919563604516554, 216.5000000000000000, -0.1155267958017906493 ) ) ;
#33238=CARTESIAN_POINT ( 'NONE',  ( -51.78497103062156981, 206.1606490808709111, -2.350049139982163027 ) ) ;
#33239=CARTESIAN_POINT ( 'NONE',  ( -60.49330436395489841, 210.1155267958017134, -6.500000000000000888 ) ) ;
#33242=CARTESIAN_POINT ( 'NONE',  ( -44.05877896937850124, 212.1620413398627534, -8.530955311639255356 ) ) ;
#33255=CARTESIAN_POINT ( 'NONE',  ( -36.14955436395490551, 214.8429017333601792, -4.673758765035196383 ) ) ;
#33284=CARTESIAN_POINT ( 'NONE',  ( -49.40252896937850124, 207.6499508600178387, -3.839350919129087547 ) ) ;
#33288=CARTESIAN_POINT ( 'NONE',  ( -40.89955436395488420, 214.8429017333601792, -4.673758765035196383 ) ) ;
#33289=CARTESIAN_POINT ( 'NONE',  ( -54.75372103062156270, 218.5309553116391896, -2.162041339862839084 ) ) ;
#33293=CARTESIAN_POINT ( 'NONE',  ( -48.01711230271182274, 216.4690446883607535, -1.857196546604089393 ) ) ;
#33303=CARTESIAN_POINT ( 'NONE',  ( -57.32663769728823411, 204.3130714775002730, 3.149950860017883603 ) ) ;
#33307=CARTESIAN_POINT ( 'NONE',  ( -40.70163769728823411, 217.4189793300686233, -4.149950860017907139 ) ) ;
#33325=VERTEX_POINT ( 'NONE', #16943 ) ;
#33331=CARTESIAN_POINT ( 'NONE',  ( -62.47247103062156981, 207.6499508600178387, 3.839350919129076445 ) ) ;
#33382=CARTESIAN_POINT ( 'NONE',  ( -55.53794563604517975, 203.8621396198271043, 6.307003348498029460 ) ) ;
#33385=CARTESIAN_POINT ( 'NONE',  ( -30.40252896937850124, 207.6499508600178387, -3.839350919129087547 ) ) ;
#33418=CARTESIAN_POINT ( 'NONE',  ( -51.57961230271182274, 211.8571965466040297, 6.469044688360755302 ) ) ;
#33422=CARTESIAN_POINT ( 'NONE',  ( -50.59747103062156981, 212.3500491399821613, -3.839350919129076445 ) ) ;
#33423=CARTESIAN_POINT ( 'NONE',  ( -55.74330436395489841, 210.1155267958017134, -6.500000000000000888 ) ) ;
#33426=CARTESIAN_POINT ( 'NONE',  ( -44.45461230271183695, 207.6069050685336492, -8.469044688360751749 ) ) ;
#33466=CARTESIAN_POINT ( 'NONE',  ( -61.07961230271182984, 211.3212981617417938, 4.469044688360757966 ) ) ;
#33470=CARTESIAN_POINT ( 'NONE',  ( -43.67038769728823411, 208.1428034533959703, 6.469044688360770401 ) ) ;
#33471=CARTESIAN_POINT ( 'NONE',  ( -55.54538769728824832, 212.3930949314662371, -8.469044688360781947 ) ) ;
#33475=CARTESIAN_POINT ( 'NONE',  ( -41.88169563604517265, 210.1155267958017703, 6.500000000000000888 ) ) ;
#33484=CARTESIAN_POINT ( 'NONE',  ( -58.71205436395489841, 214.6737587650351884, 4.842901733360205796 ) ) ;
#33488=CARTESIAN_POINT ( 'NONE',  ( -36.74330436395489130, 210.1155267958016850, -8.500000000000003553 ) ) ;
#33514=CARTESIAN_POINT ( 'NONE',  ( -57.52455436395489841, 206.6211998817774997, 3.209657149897401585 ) ) ;
#33568=CARTESIAN_POINT ( 'NONE',  ( -55.93377896937850124, 207.8379586601372750, 8.530955311639258909 ) ) ;
#33572=CARTESIAN_POINT ( 'NONE',  ( -38.91294563604516554, 213.2096571498974527, -3.378800118222469617 ) ) ;
#33608=CARTESIAN_POINT ( 'NONE',  ( -49.20461230271183695, 208.1428034533959135, -6.469044688360754414 ) ) ;
#33611=CARTESIAN_POINT ( 'NONE',  ( -33.97247103062156270, 207.6499508600178387, 3.839350919129076445 ) ) ;
#33612=CARTESIAN_POINT ( 'NONE',  ( -58.11830436395490551, 209.8844732041982581, 6.500000000000000888 ) ) ;
#33616=CARTESIAN_POINT ( 'NONE',  ( -41.68377896937850124, 207.8379586601372750, 8.530955311639258909 ) ) ;
#33652=CARTESIAN_POINT ( 'NONE',  ( -63.05877896937850124, 211.6261429550004891, -6.530955311639245586 ) ) ;
#33654=CARTESIAN_POINT ( 'NONE',  ( -53.75669563604516554, 209.8844732041982297, -4.499999999999996447 ) ) ;
#33658=CARTESIAN_POINT ( 'NONE',  ( -35.15997103062156270, 215.5714017266979852, 3.350049139982118618 ) ) ;
#33659=CARTESIAN_POINT ( 'NONE',  ( -60.69122103062156981, 207.8379586601371329, -8.530955311639223382 ) ) ;
#33663=CARTESIAN_POINT ( 'NONE',  ( -49.79836230271183695, 204.3130714775002446, -3.149950860017828091 ) ) ;
#33672=CARTESIAN_POINT ( 'NONE',  ( -50.00372103062156981, 216.5309553116392181, -1.626142955000564383 ) ) ;
#33676=CARTESIAN_POINT ( 'NONE',  ( -63.65997103062156981, 215.5714017266979852, 3.350049139982118618 ) ) ;
#33702=CARTESIAN_POINT ( 'NONE',  ( -57.12872103062156270, 205.4690446883607535, 1.090244570138264368 ) ) ;
#33752=CARTESIAN_POINT ( 'NONE',  ( -42.87127896937849414, 218.5309553116392465, 2.162041339862725842 ) ) ;
#33755=CARTESIAN_POINT ( 'NONE',  ( -34.55877896937850124, 211.0902445701383101, -4.530955311639234040 ) ) ;
#33760=CARTESIAN_POINT ( 'NONE',  ( -47.03497103062156981, 204.4285982733020148, -3.350049139982115509 ) ) ;
#33792=CARTESIAN_POINT ( 'NONE',  ( -44.65252896937850835, 206.6499508600178387, -5.571401726697954970 ) ) ;
#33798=CARTESIAN_POINT ( 'NONE',  ( -33.77455436395489841, 206.6211998817774997, 3.209657149897401585 ) ) ;
#33799=CARTESIAN_POINT ( 'NONE',  ( -53.36830436395489841, 209.8844732041982581, 6.500000000000000888 ) ) ;
#33804=CARTESIAN_POINT ( 'NONE',  ( -69.20163769728823411, 217.4189793300686233, -4.149950860017907139 ) ) ;
#33823=CARTESIAN_POINT ( 'NONE',  ( -61.08705436395488420, 205.3262412349647263, -4.842901733360204020 ) ) ;
#33841=CARTESIAN_POINT ( 'NONE',  ( -67.21502896937850835, 215.5714017266979567, -3.350049139982168800 ) ) ;
#33843=CARTESIAN_POINT ( 'NONE',  ( -51.57961230271184405, 211.3212981617417938, 4.469044688360757966 ) ) ;
#33846=CARTESIAN_POINT ( 'NONE',  ( -36.54538769728823411, 211.8571965466039444, -6.469044688360768625 ) ) ;
#33847=CARTESIAN_POINT ( 'NONE',  ( -58.11830436395491262, 209.8844732041983150, 8.500000000000003553 ) ) ;
#33851=CARTESIAN_POINT ( 'NONE',  ( -31.59002896937850124, 204.4285982733020433, 3.350049139982171020 ) ) ;
#33859=CARTESIAN_POINT ( 'NONE',  ( -43.07663769728823411, 204.3130714775002730, 3.149950860017883603 ) ) ;
#33863=CARTESIAN_POINT ( 'NONE',  ( -68.60788769728823411, 216.4690446883607535, 1.857196546604031662 ) ) ;
#33888=CARTESIAN_POINT ( 'NONE',  ( -58.71205436395490551, 213.2096571498974242, 3.378800118222489601 ) ) ;
#33935=CARTESIAN_POINT ( 'NONE',  ( -37.52752896937849414, 214.3500491399821897, 7.303452534266821949 ) ) ;
#33938=CARTESIAN_POINT ( 'NONE',  ( -36.53794563604517265, 206.7903428501025758, 3.378800118222471838 ) ) ;
#33941=CARTESIAN_POINT ( 'NONE',  ( -42.68080436395489841, 203.5000000000000000, -0.1155267958017335561 ) ) ;
#33974=CARTESIAN_POINT ( 'NONE',  ( -41.28794563604515133, 205.3262412349647832, 4.842901733360250205 ) ) ;
#33978=CARTESIAN_POINT ( 'NONE',  ( -66.62127896937849414, 214.5309553116392749, 1.090244570138288127 ) ) ;
#33979=CARTESIAN_POINT ( 'NONE',  ( -48.81622103062156270, 211.6261429550005744, 6.530955311639227823 ) ) ;
#33982=CARTESIAN_POINT ( 'NONE',  ( -67.61830436395490551, 209.8844732041983150, 8.500000000000003553 ) ) ;
#34021=CARTESIAN_POINT ( 'NONE',  ( -59.89211230271182984, 203.5309553116391896, 1.857196546604092724 ) ) ;
#34023=CARTESIAN_POINT ( 'NONE',  ( -43.26711230271184405, 214.4690446883608104, -1.321298161741814914 ) ) ;
#34027=CARTESIAN_POINT ( 'NONE',  ( -33.57663769728823411, 204.3130714775002730, 3.149950860017883603 ) ) ;
#34028=CARTESIAN_POINT ( 'NONE',  ( -42.48288769728823411, 201.5309553116392181, -2.393094931466246855 ) ) ;
#34034=CARTESIAN_POINT ( 'NONE',  ( -65.43377896937850835, 207.8379586601372750, 8.530955311639258909 ) ) ;
#34042=CARTESIAN_POINT ( 'NONE',  ( -40.89955436395488420, 214.8429017333601792, -4.673758765035197271 ) ) ;
#34046=CARTESIAN_POINT ( 'NONE',  ( -66.82663769728823411, 204.3130714775002730, 3.149950860017883603 ) ) ;
#34070=CARTESIAN_POINT ( 'NONE',  ( -43.67038769728823411, 208.6787018382581778, 4.469044688360752637 ) ) ;
#34117=CARTESIAN_POINT ( 'NONE',  ( -43.46502896937849414, 217.3034525342667962, -4.350049139982195001 ) ) ;
#34120=CARTESIAN_POINT ( 'NONE',  ( -35.74627896937850124, 205.4690446883607535, -1.090244570138286351 ) ) ;
#34123=CARTESIAN_POINT ( 'NONE',  ( -48.22247103062156270, 206.6499508600178672, 5.571401726697986057 ) ) ;
#34157=CARTESIAN_POINT ( 'NONE',  ( -30.79836230271183695, 204.3130714775002446, -3.149950860017828091 ) ) ;
#34159=CARTESIAN_POINT ( 'NONE',  ( -46.82961230271183695, 211.8571965466040297, 6.469044688360755302 ) ) ;
#34164=CARTESIAN_POINT ( 'NONE',  ( -66.42336230271182274, 213.9548777149308023, 2.149950860017852960 ) ) ;
#34165=CARTESIAN_POINT ( 'NONE',  ( -41.88913769728823411, 206.8500491399821044, -5.686928522499717253 ) ) ;
#34166=ORIENTED_EDGE ( 'NONE', *, *, #9030, .T. ) ;
#34170=CARTESIAN_POINT ( 'NONE',  ( -30.20461230271183339, 207.6069050685336492, -8.469044688360751749 ) ) ;
#34189=CARTESIAN_POINT ( 'NONE',  ( -69.59747103062156270, 213.3500491399821328, -5.571401726697985168 ) ) ;
#34208=CARTESIAN_POINT ( 'NONE',  ( -57.31919563604516554, 216.5000000000000000, -0.1155267958017906493 ) ) ;
#34210=CARTESIAN_POINT ( 'NONE',  ( -46.23586230271182984, 207.8500491399821613, 3.954877714930852495 ) ) ;
#34213=CARTESIAN_POINT ( 'NONE',  ( -69.99330436395489130, 210.1155267958017703, -4.499999999999996447 ) ) ;
#34214=CARTESIAN_POINT ( 'NONE',  ( -46.24330436395489841, 210.1155267958016850, -8.500000000000003553 ) ) ;
#34219=CARTESIAN_POINT ( 'NONE',  ( -36.53794563604517265, 205.3262412349647832, 4.842901733360250205 ) ) ;
#34232=CARTESIAN_POINT ( 'NONE',  ( -65.83705436395487709, 205.3262412349647263, -4.842901733360204020 ) ) ;
#34258=CARTESIAN_POINT ( 'NONE',  ( -44.26413769728823411, 212.1499508600178387, 3.954877714930865817 ) ) ;
#34262=FACE_OUTER_BOUND ( 'NONE', #31399, .T. ) ;
#34308=CARTESIAN_POINT ( 'NONE',  ( -54.74627896937848703, 203.4690446883607535, -1.626142955000504209 ) ) ;
#34311=CARTESIAN_POINT ( 'NONE',  ( -42.28497103062156270, 204.4285982733020148, -3.350049139982115509 ) ) ;
#34345=CARTESIAN_POINT ( 'NONE',  ( -38.31919563604516554, 216.5000000000000000, -0.1155267958017906493 ) ) ;
#34348=CARTESIAN_POINT ( 'NONE',  ( -69.99330436395490551, 210.1155267958017134, -6.500000000000000888 ) ) ;
#34349=CARTESIAN_POINT ( 'NONE',  ( -66.22544563604516554, 213.3788001182224718, 3.209657149897419348 ) ) ;
#34350=CARTESIAN_POINT ( 'NONE',  ( -49.01413769728823411, 213.1499508600178672, 5.686928522499718142 ) ) ;
#34355=CARTESIAN_POINT ( 'NONE',  ( -38.12127896937850835, 218.5309553116392465, 2.162041339862725842 ) ) ;
#34362=AXIS2_PLACEMENT_3D ( 'NONE', #35137, #26991, #23974 ) ;
#34374=CARTESIAN_POINT ( 'NONE',  ( -68.01413769728823411, 213.1499508600178672, 5.686928522499718142 ) ) ;
#34392=CARTESIAN_POINT ( 'NONE',  ( -44.45461230271182274, 208.1428034533958851, -6.469044688360754414 ) ) ;
#34396=CARTESIAN_POINT ( 'NONE',  ( -43.06919563604516554, 214.5000000000000284, -0.1155267958017627827 ) ) ;
#34400=CARTESIAN_POINT ( 'NONE',  ( -32.38913769728823411, 206.8500491399821044, -5.686928522499717253 ) ) ;
#34402=CARTESIAN_POINT ( 'NONE',  ( -44.06622103062156270, 212.1620413398628671, 8.530955311639223382 ) ) ;
#34406=CARTESIAN_POINT ( 'NONE',  ( -36.93377896937850124, 208.3738570449995109, 6.530955311639247363 ) ) ;
#34417=CARTESIAN_POINT ( 'NONE',  ( -66.23288769728823411, 203.5309553116391612, -1.857196546604028775 ) ) ;
#34441=CARTESIAN_POINT ( 'NONE',  ( -42.87872103062157692, 205.4690446883607535, 1.090244570138264368 ) ) ;
#34446=CARTESIAN_POINT ( 'NONE',  ( -69.20163769728823411, 215.6869285224996986, -3.149950860017881382 ) ) ;
#34494=CARTESIAN_POINT ( 'NONE',  ( -39.11830436395489841, 209.8844732041982581, 6.500000000000000888 ) ) ;
#34530=CARTESIAN_POINT ( 'NONE',  ( -36.93377896937850124, 208.3738570449995109, 6.530955311639247363 ) ) ;
#34533=CARTESIAN_POINT ( 'NONE',  ( -53.36086230271183695, 212.1499508600178387, -3.954877714930852495 ) ) ;
#34534=CARTESIAN_POINT ( 'NONE',  ( -47.23288769728823411, 203.5309553116391612, -1.857196546604028775 ) ) ;
#34540=CARTESIAN_POINT ( 'NONE',  ( -63.65997103062157692, 217.3034525342668815, 4.350049139982096413 ) ) ;
#34556=CARTESIAN_POINT ( 'NONE',  ( -53.96205436395489130, 214.6737587650352168, 4.842901733360204908 ) ) ;
#34574=CARTESIAN_POINT ( 'NONE',  ( -56.13169563604517265, 210.1155267958017703, 6.500000000000000888 ) ) ;
#34576=CARTESIAN_POINT ( 'NONE',  ( -47.22544563604517265, 213.3788001182224718, 3.209657149897419348 ) ) ;
#34580=CARTESIAN_POINT ( 'NONE',  ( -58.71205436395490551, 213.2096571498974242, 3.378800118222489601 ) ) ;
#34581=CARTESIAN_POINT ( 'NONE',  ( -41.88913769728823411, 205.8500491399820760, -7.418979330068584233 ) ) ;
#34585=CARTESIAN_POINT ( 'NONE',  ( -36.14211230271182984, 203.5309553116391612, 1.857196546604092280 ) ) ;
#34595=CARTESIAN_POINT ( 'NONE',  ( -47.82663769728823411, 204.3130714775002730, 3.149950860017883603 ) ) ;
#34620=CARTESIAN_POINT ( 'NONE',  ( -41.29538769728824121, 211.3212981617418222, -4.469044688360751749 ) ) ;
#34675=CARTESIAN_POINT ( 'NONE',  ( -36.94122103062157692, 208.3738570449993404, -6.530955311639226935 ) ) ;
#34709=CARTESIAN_POINT ( 'NONE',  ( -66.22544563604516554, 216.3070033484980854, 6.137860380172893926 ) ) ;
#34711=( NAMED_UNIT ( * ) SI_UNIT ( $, .STERADIAN. ) SOLID_ANGLE_UNIT ( ) );
#34713=CARTESIAN_POINT ( 'NONE',  ( -62.26711230271183695, 214.4690446883608104, -1.321298161741814914 ) ) ;
#34715=CARTESIAN_POINT ( 'NONE',  ( -47.62872103062154849, 203.4690446883607535, 1.626142955000567936 ) ) ;
#34721=CARTESIAN_POINT ( 'NONE',  ( -54.95163769728822700, 217.4189793300686233, -4.149950860017907139 ) ) ;
#34729=CARTESIAN_POINT ( 'NONE',  ( -44.85788769728822700, 216.4690446883607535, 1.857196546604031662 ) ) ;
#34742=CARTESIAN_POINT ( 'NONE',  ( -56.53497103062156270, 204.4285982733020148, -3.350049139982115509 ) ) ;
#34761=CARTESIAN_POINT ( 'NONE',  ( -51.18377896937849414, 208.3738570449995109, 6.530955311639247363 ) ) ;
#34763=CARTESIAN_POINT ( 'NONE',  ( -40.49627896937850835, 205.4690446883607535, -1.090244570138286351 ) ) ;
#34767=CARTESIAN_POINT ( 'NONE',  ( -53.96205436395491262, 213.2096571498974242, 3.378800118222489601 ) ) ;
#34768=CARTESIAN_POINT ( 'NONE',  ( -46.83705436395489130, 203.8621396198270475, -6.307003348497942419 ) ) ;
#34772=CARTESIAN_POINT ( 'NONE',  ( -55.14211230271182984, 201.5309553116392181, 2.393094931466368980 ) ) ;
#34782=CARTESIAN_POINT ( 'NONE',  ( -46.44122103062156270, 208.3738570449993404, -6.530955311639226935 ) ) ;
#34806=CARTESIAN_POINT ( 'NONE',  ( -47.82663769728823411, 206.0451222850691408, 2.149950860017832532 ) ) ;
#34810=CARTESIAN_POINT ( 'NONE',  ( -56.53497103062156270, 204.4285982733020148, -3.350049139982115509 ) ) ;
#34812=CARTESIAN_POINT ( 'NONE',  ( -37.72544563604516554, 216.3070033484980854, 6.137860380172893926 ) ) ;
#34824=CARTESIAN_POINT ( 'NONE',  ( -68.80580436395490551, 216.5000000000000000, 0.1155267958017343610 ) ) ;
#34863=CARTESIAN_POINT ( 'NONE',  ( -65.83705436395491972, 206.7903428501026042, -3.378800118222489157 ) ) ;
#34899=CARTESIAN_POINT ( 'NONE',  ( -63.45461230271184405, 207.6069050685336492, -8.469044688360751749 ) ) ;
#34904=CARTESIAN_POINT ( 'NONE',  ( -54.54836230271183695, 206.0451222850691977, -2.149950860017851184 ) ) ;
#34905=CARTESIAN_POINT ( 'NONE',  ( -33.18080436395490551, 203.5000000000000000, -0.1155267958017335561 ) ) ;
#34910=CARTESIAN_POINT ( 'NONE',  ( -60.09747103062157692, 214.3500491399821044, -7.303452534266878793 ) ) ;
#34915=CARTESIAN_POINT ( 'NONE',  ( -41.88913769728823411, 206.8500491399821044, -5.686928522499717253 ) ) ;
#34927=CARTESIAN_POINT ( 'NONE',  ( -59.70163769728823411, 215.6869285224996986, -3.149950860017881382 ) ) ;
#34943=CARTESIAN_POINT ( 'NONE',  ( -50.59002896937850124, 204.4285982733020433, 3.350049139982171020 ) ) ;
#34945=CARTESIAN_POINT ( 'NONE',  ( -66.62127896937846572, 216.5309553116391612, 1.626142955000506873 ) ) ;
#34948=CARTESIAN_POINT ( 'NONE',  ( -64.64955436395490551, 213.3788001182225003, -3.209657149897400252 ) ) ;
#34949=CARTESIAN_POINT ( 'NONE',  ( -65.83705436395487709, 205.3262412349647263, -4.842901733360204020 ) ) ;
#34954=CARTESIAN_POINT ( 'NONE',  ( -58.70461230271184405, 207.6069050685336492, -8.469044688360751749 ) ) ;
#34967=CARTESIAN_POINT ( 'NONE',  ( -47.03497103062156981, 204.4285982733020148, -3.350049139982115509 ) ) ;
#34995=CARTESIAN_POINT ( 'NONE',  ( -66.81919563604516554, 214.5000000000000284, -0.1155267958017627827 ) ) ;
#34999=CARTESIAN_POINT ( 'NONE',  ( -64.45163769728823411, 215.6869285224996986, -3.149950860017881382 ) ) ;
#35000=CARTESIAN_POINT ( 'NONE',  ( -44.45461230271183695, 207.6069050685336492, -8.469044688360751749 ) ) ;
#35005=CARTESIAN_POINT ( 'NONE',  ( -63.45461230271182274, 208.1428034533959135, -6.469044688360754414 ) ) ;
#35047=CARTESIAN_POINT ( 'NONE',  ( -63.65997103062157692, 213.8393509191290889, 2.350049139982164359 ) ) ;
#35082=CARTESIAN_POINT ( 'NONE',  ( -31.39211230271182984, 203.5309553116391612, 1.857196546604092280 ) ) ;
#35087=CARTESIAN_POINT ( 'NONE',  ( -58.30877896937849414, 211.0902445701383101, -4.530955311639234040 ) ) ;
#35088=CARTESIAN_POINT ( 'NONE',  ( -35.35788769728823411, 216.4690446883607535, 1.857196546604031662 ) ) ;
#35094=CARTESIAN_POINT ( 'NONE',  ( -55.74330436395489841, 210.1155267958016850, -8.500000000000003553 ) ) ;
#35099=CARTESIAN_POINT ( 'NONE',  ( -46.83705436395489841, 205.3262412349647548, -4.842901733360204908 ) ) ;
#35112=CARTESIAN_POINT ( 'NONE',  ( -51.98288769728821990, 203.5309553116391612, -1.857196546604028775 ) ) ;
#35126=CARTESIAN_POINT ( 'NONE',  ( -45.64211230271182984, 203.5309553116391896, 1.857196546604092724 ) ) ;
#35127=CARTESIAN_POINT ( 'NONE',  ( -64.24627896937849414, 203.4690446883607535, -1.626142955000504209 ) ) ;
#35130=CARTESIAN_POINT ( 'NONE',  ( -59.70163769728823411, 213.9548777149308592, -2.149950860017830756 ) ) ;
#35131=CARTESIAN_POINT ( 'NONE',  ( -36.34747103062156981, 214.3500491399821044, -7.303452534266878793 ) ) ;
#35135=CARTESIAN_POINT ( 'NONE',  ( -60.09002896937850124, 202.6965474657332038, 4.350049139982197666 ) ) ;
#35137=CARTESIAN_POINT ( 'NONE',  ( -68.00669563604516554, 209.8844732041982013, -6.500000000000000888 ) ) ;
#35148=CARTESIAN_POINT ( 'NONE',  ( -49.80580436395490551, 216.5000000000000000, 0.1155267958017343610 ) ) ;
#35177=CARTESIAN_POINT ( 'NONE',  ( -35.55580436395489130, 214.5000000000000284, 0.1155267958017899832 ) ) ;
#35181=CARTESIAN_POINT ( 'NONE',  ( -57.92038769728821990, 208.1428034533959703, 6.469044688360770401 ) ) ;
#35182=CARTESIAN_POINT ( 'NONE',  ( -67.42038769728826253, 207.6069050685337913, 8.469044688360781947 ) ) ;
#35188=CARTESIAN_POINT ( 'NONE',  ( -62.06919563604516554, 216.5000000000000000, -0.1155267958017906493 ) ) ;
#35233=CARTESIAN_POINT ( 'NONE',  ( -36.34747103062156981, 213.3500491399821328, -5.571401726697985168 ) ) ;
#35265=CARTESIAN_POINT ( 'NONE',  ( -32.77752896937850124, 213.3500491399821613, 5.571401726697954970 ) ) ;
#35268=CARTESIAN_POINT ( 'NONE',  ( -62.66294563604517265, 213.2096571498974527, -3.378800118222469617 ) ) ;
#35275=CARTESIAN_POINT ( 'NONE',  ( -64.05580436395490551, 218.5000000000000000, 0.1155267958017064944 ) ) ;
#35281=CARTESIAN_POINT ( 'NONE',  ( -33.97247103062156270, 206.6499508600178672, 5.571401726697986057 ) ) ;
#35310=CARTESIAN_POINT ( 'NONE',  ( -39.11086230271183695, 213.1499508600178387, -5.686928522499747451 ) ) ;
#35312=CARTESIAN_POINT ( 'NONE',  ( -35.54836230271182984, 206.0451222850691977, -2.149950860017851184 ) ) ;
#35315=CARTESIAN_POINT ( 'NONE',  ( -55.54538769728824832, 211.3212981617418222, -4.469044688360751749 ) ) ;
#35317=CARTESIAN_POINT ( 'NONE',  ( -68.21205436395489130, 214.6737587650352168, 4.842901733360204908 ) ) ;
#35321=CARTESIAN_POINT ( 'NONE',  ( -53.16294563604516554, 216.1378603801729241, -6.307003348498026796 ) ) ;
#35332=CARTESIAN_POINT ( 'NONE',  ( -53.76413769728823411, 213.1499508600178672, 5.686928522499718142 ) ) ;
#35349=CIRCLE ( 'NONE', #24471, 1.000000000000002220 ) ;
#35362=CARTESIAN_POINT ( 'NONE',  ( -37.33705436395491262, 206.7903428501026042, -3.378800118222489157 ) ) ;
#35366=CARTESIAN_POINT ( 'NONE',  ( -61.87872103062154849, 203.4690446883607535, 1.626142955000567936 ) ) ;
#35367=CARTESIAN_POINT ( 'NONE',  ( -32.18377896937850124, 207.8379586601372750, 8.530955311639258909 ) ) ;
#35372=CARTESIAN_POINT ( 'NONE',  ( -58.90252896937850124, 206.6499508600178387, -5.571401726697954970 ) ) ;
#35380=CARTESIAN_POINT ( 'NONE',  ( -69.99330436395490551, 210.1155267958017134, -6.500000000000000888 ) ) ;
#35420=CARTESIAN_POINT ( 'NONE',  ( -64.64955436395490551, 213.3788001182225003, -3.209657149897400252 ) ) ;
#35460=CARTESIAN_POINT ( 'NONE',  ( -33.56919563604517265, 216.5000000000000000, -0.1155267958017906493 ) ) ;
#35463=CARTESIAN_POINT ( 'NONE',  ( -47.42336230271184405, 213.9548777149308023, 2.149950860017852960 ) ) ;
#35469=CARTESIAN_POINT ( 'NONE',  ( -50.59747103062156981, 214.3500491399821044, -7.303452534266878793 ) ) ;
#35504=CARTESIAN_POINT ( 'NONE',  ( -32.77752896937850124, 213.3500491399821613, 5.571401726697954970 ) ) ;
#35506=CARTESIAN_POINT ( 'NONE',  ( -34.16294563604517265, 213.2096571498974527, -3.378800118222469617 ) ) ;
#35510=CARTESIAN_POINT ( 'NONE',  ( -52.57663769728824832, 206.0451222850691408, 2.149950860017832532 ) ) ;
#35511=CARTESIAN_POINT ( 'NONE',  ( -38.32663769728823411, 202.5810206699313767, 4.149950860017909804 ) ) ;
#35516=CARTESIAN_POINT ( 'NONE',  ( -52.37127896937850835, 218.5309553116392465, 2.162041339862725842 ) ) ;
#35529=CARTESIAN_POINT ( 'NONE',  ( -34.36830436395490551, 209.8844732041982581, 6.500000000000000888 ) ) ;
#35556=CARTESIAN_POINT ( 'NONE',  ( -32.78497103062156981, 206.1606490808709111, -2.350049139982163027 ) ) ;
#35561=CARTESIAN_POINT ( 'NONE',  ( -61.48288769728821990, 203.5309553116391612, -1.857196546604028775 ) ) ;
#35562=CARTESIAN_POINT ( 'NONE',  ( -30.20461230271183339, 207.6069050685336492, -8.469044688360751749 ) ) ;
#35566=CARTESIAN_POINT ( 'NONE',  ( -63.85044563604516554, 205.1570982666397072, -4.673758765035155527 ) ) ;
#35574=CARTESIAN_POINT ( 'NONE',  ( -69.00372103062156270, 216.5309553116392181, -1.626142955000564383 ) ) ;
#35578=CARTESIAN_POINT ( 'NONE',  ( -33.57663769728823411, 202.5810206699313767, 4.149950860017909804 ) ) ;
#35605=CLOSED_SHELL ( 'NONE', ( #33228, #1215, #24657, #13716 ) ) ;
#35651=CARTESIAN_POINT ( 'NONE',  ( -61.27752896937849414, 214.3500491399821897, 7.303452534266821949 ) ) ;
#35654=CARTESIAN_POINT ( 'NONE',  ( -44.85044563604516554, 206.6211998817775566, -3.209657149897419348 ) ) ;
#35660=CARTESIAN_POINT ( 'NONE',  ( -53.76413769728823411, 214.1499508600179240, 7.418979330068584233 ) ) ;
#35689=CARTESIAN_POINT ( 'NONE',  ( -36.14211230271182984, 203.5309553116391896, 1.857196546604092724 ) ) ;
#35691=CARTESIAN_POINT ( 'NONE',  ( -34.55877896937850124, 211.0902445701383101, -4.530955311639234040 ) ) ;
#35694=CARTESIAN_POINT ( 'NONE',  ( -44.26413769728823411, 212.1499508600178387, 3.954877714930865817 ) ) ;
#35695=CARTESIAN_POINT ( 'NONE',  ( -32.58705436395489841, 203.8621396198270475, -6.307003348497942419 ) ) ;
#35699=CARTESIAN_POINT ( 'NONE',  ( -39.90252896937850124, 205.6499508600178103, -7.303452534266820173 ) ) ;
#35740=CARTESIAN_POINT ( 'NONE',  ( -32.58705436395489841, 206.7903428501026042, -3.378800118222489157 ) ) ;
#35744=CARTESIAN_POINT ( 'NONE',  ( -48.02455436395488420, 205.1570982666397356, 4.673758765035198159 ) ) ;
#35745=CARTESIAN_POINT ( 'NONE',  ( -65.63913769728821990, 205.8500491399820760, -7.418979330068584233 ) ) ;
#35750=CARTESIAN_POINT ( 'NONE',  ( -40.69419563604516554, 203.5000000000000000, 0.1155267958017914542 ) ) ;
#35758=CARTESIAN_POINT ( 'NONE',  ( -51.19122103062156270, 208.3738570449994256, -6.530955311639227823 ) ) ;
#35762=CARTESIAN_POINT ( 'NONE',  ( -33.77455436395489841, 203.6929966515020283, 6.137860380172978303 ) ) ;
#35838=CARTESIAN_POINT ( 'NONE',  ( -50.59002896937850835, 202.6965474657332038, 4.350049139982197666 ) ) ;
#35841=CARTESIAN_POINT ( 'NONE',  ( -46.63169563604517265, 210.1155267958017703, 4.499999999999996447 ) ) ;
#35847=CARTESIAN_POINT ( 'NONE',  ( -46.83705436395489130, 203.8621396198270475, -6.307003348497942419 ) ) ;
#35877=CARTESIAN_POINT ( 'NONE',  ( -39.50669563604517265, 209.8844732041982013, -6.500000000000000888 ) ) ;
#35878=CARTESIAN_POINT ( 'NONE',  ( -56.32961230271183695, 211.8571965466040297, 6.469044688360755302 ) ) ;
#35881=CARTESIAN_POINT ( 'NONE',  ( -52.18080436395490551, 205.4999999999999716, -0.1155267958017894420 ) ) ;
#35883=CARTESIAN_POINT ( 'NONE',  ( -56.53497103062156270, 204.4285982733020148, -3.350049139982115509 ) ) ;
#35887=CARTESIAN_POINT ( 'NONE',  ( -50.39211230271182984, 201.5309553116392181, 2.393094931466368980 ) ) ;
#35900=CARTESIAN_POINT ( 'NONE',  ( -43.67038769728823411, 208.1428034533959703, 6.469044688360770401 ) ) ;
#35928=CARTESIAN_POINT ( 'NONE',  ( -58.30877896937849414, 211.0902445701383101, -4.530955311639234040 ) ) ;
#35932=CARTESIAN_POINT ( 'NONE',  ( -43.47247103062156981, 206.6499508600178672, 5.571401726697986057 ) ) ;
#35933=CARTESIAN_POINT ( 'NONE',  ( -31.59002896937850124, 202.6965474657332038, 4.350049139982197666 ) ) ;
#35935=APPLICATION_CONTEXT ( 'automotive_design' ) ;
#35939=CARTESIAN_POINT ( 'NONE',  ( -42.47544563604516554, 214.8429017333602360, 4.673758765035156415 ) ) ;
#35948=CARTESIAN_POINT ( 'NONE',  ( -49.21205436395489841, 214.6737587650351884, 4.842901733360205796 ) ) ;
#35952=CARTESIAN_POINT ( 'NONE',  ( -40.50372103062156981, 218.5309553116391896, -2.162041339862839084 ) ) ;
#35963=CARTESIAN_POINT ( 'NONE',  ( -64.84747103062156270, 213.3500491399821328, -5.571401726697985168 ) ) ;
#35979=CARTESIAN_POINT ( 'NONE',  ( -52.37872103062156981, 205.4690446883607535, 1.090244570138264368 ) ) ;
#36025=CARTESIAN_POINT ( 'NONE',  ( -53.95461230271185116, 207.6069050685336492, -8.469044688360751749 ) ) ;
#36029=CARTESIAN_POINT ( 'NONE',  ( -49.40252896937850124, 207.6499508600178387, -3.839350919129087547 ) ) ;
#36036=CARTESIAN_POINT ( 'NONE',  ( -47.82663769728823411, 202.5810206699313767, 4.149950860017909804 ) ) ;
#36067=CARTESIAN_POINT ( 'NONE',  ( -35.94419563604516554, 203.5000000000000000, 0.1155267958017914542 ) ) ;
#36068=CARTESIAN_POINT ( 'NONE',  ( -56.92336230271182984, 215.6869285224997270, 3.149950860017831200 ) ) ;
#36071=CARTESIAN_POINT ( 'NONE',  ( -51.98288769728823411, 205.5309553116392465, -1.321298161741839117 ) ) ;
#36072=CARTESIAN_POINT ( 'NONE',  ( -57.52455436395488420, 205.1570982666397356, 4.673758765035198159 ) ) ;
#36076=CARTESIAN_POINT ( 'NONE',  ( -46.82961230271182984, 212.3930949314663792, 8.469044688360751749 ) ) ;
#36088=CARTESIAN_POINT ( 'NONE',  ( -41.88913769728823411, 206.8500491399821044, -5.686928522499717253 ) ) ;
#36118=CARTESIAN_POINT ( 'NONE',  ( -49.79836230271183695, 206.0451222850691977, -2.149950860017851184 ) ) ;
#36122=CARTESIAN_POINT ( 'NONE',  ( -41.49330436395490551, 210.1155267958017134, -6.500000000000000888 ) ) ;
#36123=CARTESIAN_POINT ( 'NONE',  ( -59.50372103062157692, 218.5309553116391896, -2.162041339862839084 ) ) ;
#36127=CARTESIAN_POINT ( 'NONE',  ( -48.61086230271182984, 213.1499508600178387, -5.686928522499747451 ) ) ;
#36135=CARTESIAN_POINT ( 'NONE',  ( -60.69122103062155560, 208.3738570449994256, -6.530955311639227823 ) ) ;
#36139=CARTESIAN_POINT ( 'NONE',  ( -32.78497103062156981, 202.6965474657331185, -4.350049139982091084 ) ) ;
#36161=CARTESIAN_POINT ( 'NONE',  ( -53.76413769728823411, 212.1499508600178387, 3.954877714930865817 ) ) ;
#36208=CARTESIAN_POINT ( 'NONE',  ( -59.69419563604517265, 201.5000000000000000, 0.1155267958018195706 ) ) ;
#36213=CARTESIAN_POINT ( 'NONE',  ( -41.88169563604517265, 210.1155267958017703, 4.499999999999996447 ) ) ;
#36219=CARTESIAN_POINT ( 'NONE',  ( -50.20163769728823411, 217.4189793300686233, -4.149950860017907139 ) ) ;
#36250=CARTESIAN_POINT ( 'NONE',  ( -57.12127896937847993, 216.5309553116391612, 1.626142955000506873 ) ) ;
#36254=CARTESIAN_POINT ( 'NONE',  ( -50.39955436395490551, 213.3788001182225003, -3.209657149897400252 ) ) ;
#36255=CARTESIAN_POINT ( 'NONE',  ( -56.73288769728823411, 203.5309553116391612, -1.857196546604028775 ) ) ;
#36260=CARTESIAN_POINT ( 'NONE',  ( -47.81919563604517265, 218.5000000000000000, -0.1155267958018185298 ) ) ;
#36271=CARTESIAN_POINT ( 'NONE',  ( -41.09747103062156981, 213.3500491399821328, -5.571401726697985168 ) ) ;
#36297=CARTESIAN_POINT ( 'NONE',  ( -55.73586230271182984, 207.8500491399821613, 3.954877714930852495 ) ) ;
#36301=CARTESIAN_POINT ( 'NONE',  ( -47.82663769728823411, 204.3130714775002730, 3.149950860017883603 ) ) ;
#36302=CARTESIAN_POINT ( 'NONE',  ( -57.52455436395489841, 203.6929966515020283, 6.137860380172978303 ) ) ;
#36307=CARTESIAN_POINT ( 'NONE',  ( -50.59002896937850124, 204.4285982733020433, 3.350049139982171020 ) ) ;
#36316=CARTESIAN_POINT ( 'NONE',  ( -50.99330436395489841, 210.1155267958017134, -6.500000000000000888 ) ) ;
#36321=CARTESIAN_POINT ( 'NONE',  ( -41.49330436395490551, 210.1155267958016850, -8.500000000000003553 ) ) ;
#36340=ORIENTED_EDGE ( 'NONE', *, *, #33116, .T. ) ;
#36347=CARTESIAN_POINT ( 'NONE',  ( -59.10788769728823411, 214.4690446883608104, 1.321298161741840893 ) ) ;
#36395=CARTESIAN_POINT ( 'NONE',  ( -59.29836230271182984, 202.5810206699313767, -4.149950860017804111 ) ) ;
#36398=CARTESIAN_POINT ( 'NONE',  ( -31.78794563604516910, 206.7903428501025758, 3.378800118222471838 ) ) ;
#36434=CARTESIAN_POINT ( 'NONE',  ( -60.48586230271183695, 206.8500491399821328, 5.686928522499748340 ) ) ;
#36440=CARTESIAN_POINT ( 'NONE',  ( -32.78497103062156981, 206.1606490808709111, -2.350049139982163027 ) ) ;
#36441=CARTESIAN_POINT ( 'NONE',  ( -55.34747103062156981, 213.3500491399821328, -5.571401726697985168 ) ) ;
#36445=CARTESIAN_POINT ( 'NONE',  ( -50.98586230271183695, 205.8500491399821613, 7.418979330068642852 ) ) ;
#36483=CARTESIAN_POINT ( 'NONE',  ( -67.61086230271183695, 213.1499508600178387, -5.686928522499747451 ) ) ;
#36485=CARTESIAN_POINT ( 'NONE',  ( -54.54836230271183695, 206.0451222850691977, -2.149950860017851184 ) ) ;
#36490=CARTESIAN_POINT ( 'NONE',  ( -46.63913769728824121, 206.8500491399821044, -5.686928522499717253 ) ) ;
#36491=CARTESIAN_POINT ( 'NONE',  ( -61.68080436395489841, 201.5000000000000000, -0.1155267958017054536 ) ) ;
#36495=CARTESIAN_POINT ( 'NONE',  ( -42.67336230271183695, 215.6869285224997270, 3.149950860017831200 ) ) ;
#36504=CARTESIAN_POINT ( 'NONE',  ( -52.37872103062156270, 203.4690446883607535, 1.626142955000567936 ) ) ;
#36509=CARTESIAN_POINT ( 'NONE',  ( -61.08705436395488420, 205.3262412349647263, -4.842901733360204020 ) ) ;
#36534=CARTESIAN_POINT ( 'NONE',  ( -60.29538769728823411, 211.3212981617418222, -4.469044688360751749 ) ) ;
#36584=CARTESIAN_POINT ( 'NONE',  ( -47.81919563604517265, 218.5000000000000000, -0.1155267958018185298 ) ) ;
#36588=CARTESIAN_POINT ( 'NONE',  ( -64.84002896937850835, 204.4285982733020433, 3.350049139982171020 ) ) ;
#36625=CARTESIAN_POINT ( 'NONE',  ( -47.62127896937847993, 216.5309553116391612, 1.626142955000506873 ) ) ;
#36628=CARTESIAN_POINT ( 'NONE',  ( -65.43377896937850835, 208.9097554298617183, 4.530955311639234040 ) ) ;
#36629=CARTESIAN_POINT ( 'NONE',  ( -61.08705436395488420, 205.3262412349647263, -4.842901733360204020 ) ) ;
#36634=CARTESIAN_POINT ( 'NONE',  ( -39.30877896937850124, 212.1620413398627534, -8.530955311639255356 ) ) ;
#36655=CARTESIAN_POINT ( 'NONE',  ( -63.06622103062156981, 211.6261429550005744, 6.530955311639227823 ) ) ;
#36675=CARTESIAN_POINT ( 'NONE',  ( -59.10044563604517265, 205.1570982666397072, -4.673758765035155527 ) ) ;
#36677=CARTESIAN_POINT ( 'NONE',  ( -52.37127896937850835, 214.5309553116392749, 1.090244570138288127 ) ) ;
#36681=CARTESIAN_POINT ( 'NONE',  ( -67.22247103062156270, 207.6499508600178387, 3.839350919129076445 ) ) ;
#36682=CARTESIAN_POINT ( 'NONE',  ( -57.32663769728824121, 202.5810206699313767, 4.149950860017909804 ) ) ;
#36686=CARTESIAN_POINT ( 'NONE',  ( -34.95461230271183695, 208.1428034533959135, -6.469044688360754414 ) ) ;
#36694=CARTESIAN_POINT ( 'NONE',  ( -44.06622103062156981, 211.6261429550005744, 6.530955311639228711 ) ) ;
#36698=CARTESIAN_POINT ( 'NONE',  ( -68.80580436395490551, 216.5000000000000000, 0.1155267958017343610 ) ) ;
#36700=( NAMED_UNIT ( * ) PLANE_ANGLE_UNIT ( ) SI_UNIT ( $, .RADIAN. ) );
#36724=CARTESIAN_POINT ( 'NONE',  ( -60.69122103062156981, 208.9097554298617752, -4.530955311639240257 ) ) ;
#36770=CARTESIAN_POINT ( 'NONE',  ( -42.27752896937850835, 214.3500491399821897, 7.303452534266821949 ) ) ;
#36772=CARTESIAN_POINT ( 'NONE',  ( -65.82961230271179431, 211.8571965466040297, 6.469044688360755302 ) ) ;
#36775=CARTESIAN_POINT ( 'NONE',  ( -47.43080436395489841, 203.5000000000000000, -0.1155267958017335561 ) ) ;
#36809=CARTESIAN_POINT ( 'NONE',  ( -43.66294563604516554, 214.6737587650350747, -4.842901733360249317 ) ) ;
#36814=CARTESIAN_POINT ( 'NONE',  ( -38.72247103062156981, 207.6499508600178387, 3.839350919129076445 ) ) ;
#36815=CARTESIAN_POINT ( 'NONE',  ( -39.90997103062156270, 215.5714017266979852, 3.350049139982118618 ) ) ;
#36820=CARTESIAN_POINT ( 'NONE',  ( -33.76711230271183695, 218.4690446883607535, -2.393094931466363651 ) ) ;
#36838=CARTESIAN_POINT ( 'NONE',  ( -67.42038769728823411, 208.1428034533959703, 6.469044688360770401 ) ) ;
#36855=CARTESIAN_POINT ( 'NONE',  ( -61.87127896937849414, 216.5309553116392181, 1.626142955000506429 ) ) ;
#36857=CARTESIAN_POINT ( 'NONE',  ( -44.25669563604517265, 209.8844732041982297, -4.499999999999996447 ) ) ;
#36861=CARTESIAN_POINT ( 'NONE',  ( -66.23288769728823411, 205.5309553116392465, -1.321298161741839117 ) ) ;
#36862=CARTESIAN_POINT ( 'NONE',  ( -60.88913769728824121, 205.8500491399820760, -7.418979330068584233 ) ) ;
#36866=CARTESIAN_POINT ( 'NONE',  ( -32.57961230271183695, 211.8571965466040297, 6.469044688360755302 ) ) ;
#36874=CARTESIAN_POINT ( 'NONE',  ( -48.02455436395489841, 205.1570982666397640, 4.673758765035199048 ) ) ;
#36878=CARTESIAN_POINT ( 'NONE',  ( -65.44122103062157692, 208.3738570449993404, -6.530955311639226935 ) ) ;
#36902=CARTESIAN_POINT ( 'NONE',  ( -38.12872103062156270, 205.4690446883607535, 1.090244570138264368 ) ) ;
#36952=CARTESIAN_POINT ( 'NONE',  ( -48.41294563604517265, 216.1378603801729241, -6.307003348498026796 ) ) ;
#36956=CARTESIAN_POINT ( 'NONE',  ( -67.01711230271183695, 216.4690446883607535, -1.857196546604089393 ) ) ;
#36960=CARTESIAN_POINT ( 'NONE',  ( -48.02455436395488420, 205.1570982666397356, 4.673758765035198159 ) ) ;
#36994=CARTESIAN_POINT ( 'NONE',  ( -46.03794563604517265, 205.3262412349647832, 4.842901733360250205 ) ) ;
#36998=CARTESIAN_POINT ( 'NONE',  ( -40.70163769728823411, 213.9548777149308592, -2.149950860017830756 ) ) ;
#36999=CARTESIAN_POINT ( 'NONE',  ( -41.29538769728821990, 211.8571965466039444, -6.469044688360768625 ) ) ;
#37004=CARTESIAN_POINT ( 'NONE',  ( -35.35044563604517265, 203.6929966515019430, -6.137860380172892150 ) ) ;
#37014=CARTESIAN_POINT ( 'NONE',  ( -69.00000000000002842, 209.9999999999999716, -6.500000000000000888 ) ) ;
#37040=CARTESIAN_POINT ( 'NONE',  ( -66.02752896937849414, 213.3500491399821613, 5.571401726697954970 ) ) ;
#37042=CARTESIAN_POINT ( 'NONE',  ( -37.52752896937849414, 212.3500491399821613, 3.839350919129088435 ) ) ;
#37047=CARTESIAN_POINT ( 'NONE',  ( -34.17038769728823411, 208.1428034533959703, 6.469044688360770401 ) ) ;
#37048=CARTESIAN_POINT ( 'NONE',  ( -45.05580436395490551, 218.5000000000000000, 0.1155267958017064944 ) ) ;
#37053=CARTESIAN_POINT ( 'NONE',  ( -36.34002896937850124, 204.4285982733020433, 3.350049139982171020 ) ) ;
#37065=CARTESIAN_POINT ( 'NONE',  ( -59.70163769728823411, 215.6869285224996986, -3.149950860017881382 ) ) ;
#37090=CARTESIAN_POINT ( 'NONE',  ( -49.01413769728823411, 212.1499508600178387, 3.954877714930865817 ) ) ;
#37140=CARTESIAN_POINT ( 'NONE',  ( -40.89211230271183695, 201.5309553116392181, 2.393094931466368980 ) ) ;
#37143=CARTESIAN_POINT ( 'NONE',  ( -36.14211230271182984, 205.5309553116392465, 1.321298161741817356 ) ) ;
#37147=CARTESIAN_POINT ( 'NONE',  ( -43.67038769728823411, 208.1428034533959703, 6.469044688360770401 ) ) ;
#37181=CARTESIAN_POINT ( 'NONE',  ( -38.91294563604516554, 214.6737587650350747, -4.842901733360249317 ) ) ;
#37184=CARTESIAN_POINT ( 'NONE',  ( -35.95163769728824121, 213.9548777149308592, -2.149950860017830756 ) ) ;
#37185=CARTESIAN_POINT ( 'NONE',  ( -45.64955436395490551, 214.8429017333601792, -4.673758765035196383 ) ) ;
#37191=CARTESIAN_POINT ( 'NONE',  ( -69.99330436395489130, 210.1155267958016850, -8.500000000000003553 ) ) ;
#37228=CARTESIAN_POINT ( 'NONE',  ( -65.63169563604516554, 210.1155267958017703, 6.500000000000000888 ) ) ;
#37230=CARTESIAN_POINT ( 'NONE',  ( -46.03794563604517975, 206.7903428501025758, 3.378800118222471838 ) ) ;
#37233=CARTESIAN_POINT ( 'NONE',  ( -39.11830436395489841, 209.8844732041982581, 6.500000000000000888 ) ) ;
#37234=CARTESIAN_POINT ( 'NONE',  ( -49.80580436395490551, 218.5000000000000000, 0.1155267958017064944 ) ) ;
#37238=CARTESIAN_POINT ( 'NONE',  ( -37.52752896937850124, 213.3500491399821613, 5.571401726697954970 ) ) ;
#37251=CARTESIAN_POINT ( 'NONE',  ( -60.09747103062156981, 213.3500491399821328, -5.571401726697985168 ) ) ;
#37252=( LENGTH_UNIT ( ) NAMED_UNIT ( * ) SI_UNIT ( .MILLI., .METRE. ) );
#37277=CARTESIAN_POINT ( 'NONE',  ( -44.46205436395490551, 213.2096571498974242, 3.378800118222489601 ) ) ;
#37323=CARTESIAN_POINT ( 'NONE',  ( -53.55877896937850124, 211.6261429550004607, -6.530955311639245586 ) ) ;
#37326=CARTESIAN_POINT ( 'NONE',  ( -39.51413769728823411, 213.1499508600178672, 5.686928522499718142 ) ) ;
#37358=CARTESIAN_POINT ( 'NONE',  ( -42.27752896937850124, 213.3500491399821613, 5.571401726697954970 ) ) ;
#37361=CARTESIAN_POINT ( 'NONE',  ( -59.49627896937850835, 205.4690446883607535, -1.090244570138286351 ) ) ;
#37363=CARTESIAN_POINT ( 'NONE',  ( -40.70163769728823411, 215.6869285224996986, -3.149950860017881382 ) ) ;
#37370=CARTESIAN_POINT ( 'NONE',  ( -36.14211230271182984, 201.5309553116392181, 2.393094931466368980 ) ) ;
#37388=CARTESIAN_POINT ( 'NONE',  ( -52.57663769728823411, 204.3130714775002730, 3.149950860017883603 ) ) ;
#37407=CARTESIAN_POINT ( 'NONE',  ( -52.96502896937850124, 215.5714017266979567, -3.350049139982168800 ) ) ;
#37410=CARTESIAN_POINT ( 'NONE',  ( -36.93377896937849414, 208.9097554298617183, 4.530955311639234040 ) ) ;
#37414=CARTESIAN_POINT ( 'NONE',  ( -35.55580436395490551, 216.5000000000000000, 0.1155267958017343610 ) ) ;
#37415=CARTESIAN_POINT ( 'NONE',  ( -42.68080436395489841, 201.5000000000000000, -0.1155267958017054536 ) ) ;
#37419=CARTESIAN_POINT ( 'NONE',  ( -30.00669563604516910, 209.8844732041982013, -6.500000000000000888 ) ) ;
#37431=CARTESIAN_POINT ( 'NONE',  ( -49.01413769728823411, 213.1499508600178672, 5.686928522499718142 ) ) ;
#37456=CARTESIAN_POINT ( 'NONE',  ( -45.25372103062157692, 214.5309553116392749, -1.090244570138262148 ) ) ;
#37536=COLOUR_RGB('Grey',0.48,0.52,0.57);
#37537=FILL_AREA_STYLE_COLOUR('',#37536);
#37538=FILL_AREA_STYLE('',(#37537));
#37539=SURFACE_STYLE_FILL_AREA(#37538);
#37540=SURFACE_SIDE_STYLE('',(#37539));
#37541=SURFACE_STYLE_USAGE(.BOTH.,#37540);
#37542=PRESENTATION_STYLE_ASSIGNMENT((#37541));
ENDSEC;
END-ISO-10303-21;
